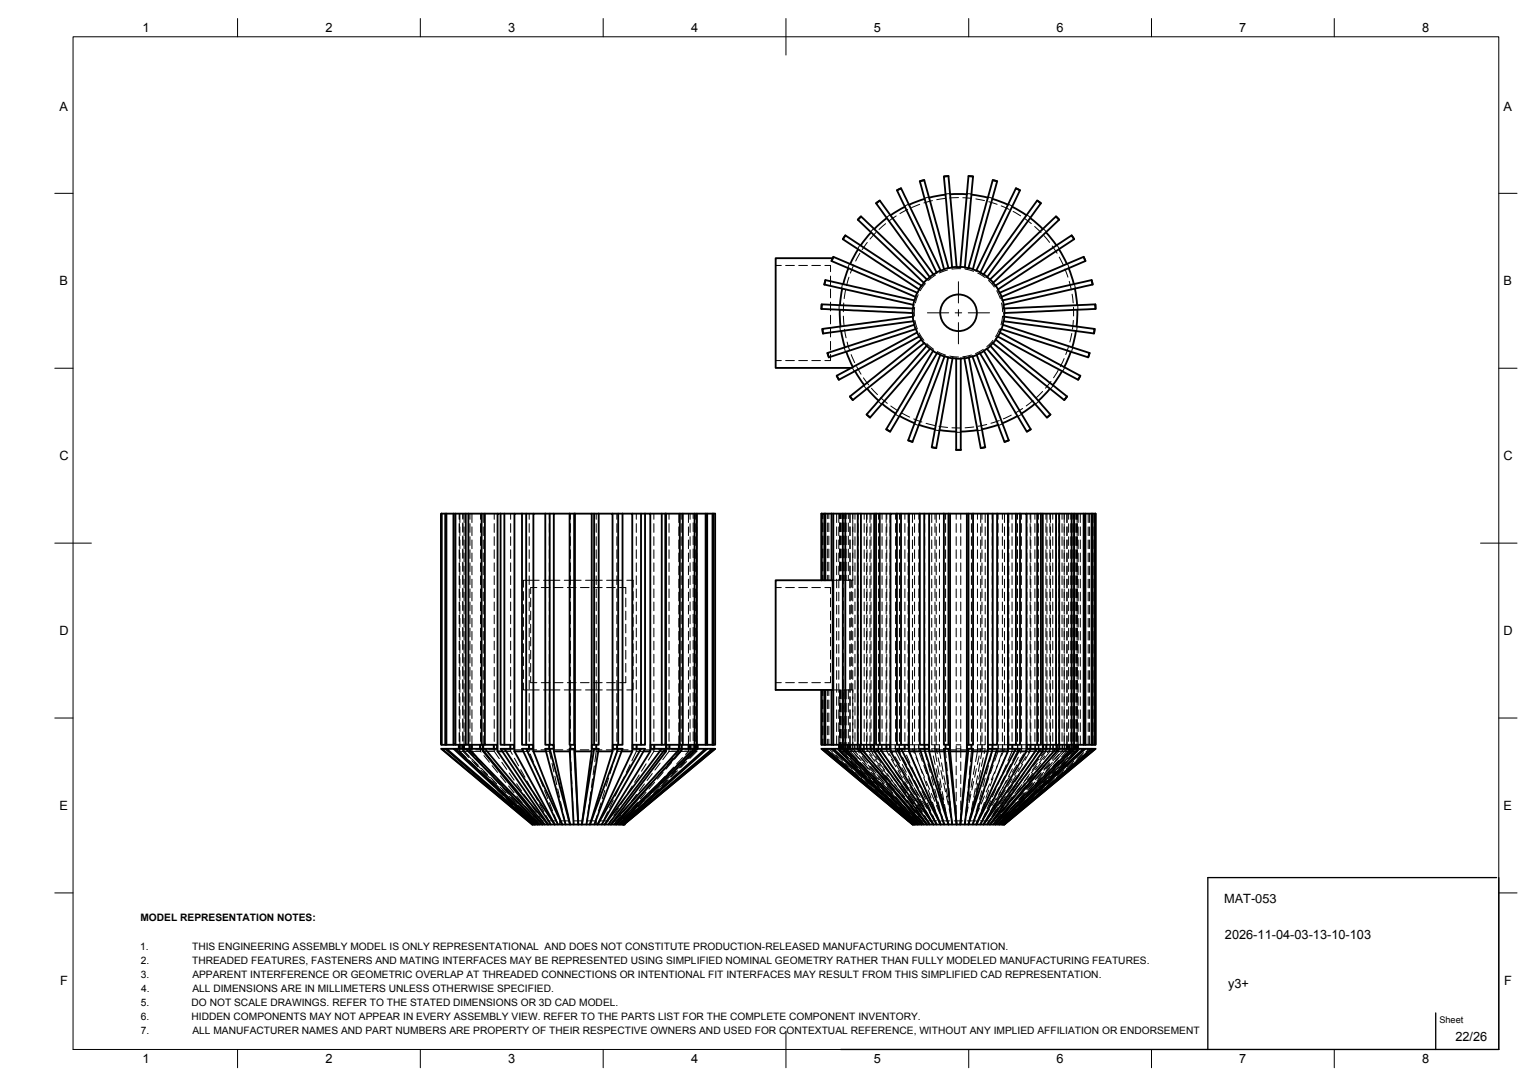
ISO-10303-21;
HEADER;
FILE_DESCRIPTION (('STEP AP214'),
    '1' );
FILE_NAME ('y3+.step',
    '2026-10-10T03:43:58',
    ( '' ),
    ( '' ),
    'SwSTEP 2.0',
    'SolidWorks 2026',
    '' );
FILE_SCHEMA (( 'AUTOMOTIVE_DESIGN' ));
ENDSEC;

DATA;
#2=ORIENTED_EDGE ( 'NONE', *, *, #57099, .F. ) ;
#4=DIRECTION ( 'NONE',  ( 0.000000000000000000, 0.000000000000000000, -1.000000000000000000 ) ) ;
#5=CARTESIAN_POINT ( 'NONE',  ( -64.61430802170492882, 7.070445451047391749, 170.0000000000000000 ) ) ;
#16=VERTEX_POINT ( 'NONE', #24964 ) ;
#40=CARTESIAN_POINT ( 'NONE',  ( 0.000000000000000000, 0.000000000000000000, 170.0000000000000000 ) ) ;
#47=ORIENTED_EDGE ( 'NONE', *, *, #8300, .T. ) ;
#51=CARTESIAN_POINT ( 'NONE',  ( -21.95369412746239846, -11.95973721106846455, 0.000000000000000000 ) ) ;
#52=ORIENTED_EDGE ( 'NONE', *, *, #19951, .T. ) ;
#76=ORIENTED_EDGE ( 'NONE', *, *, #47792, .F. ) ;
#86=ORIENTED_EDGE ( 'NONE', *, *, #42856, .F. ) ;
#93=ORIENTED_EDGE ( 'NONE', *, *, #10645, .F. ) ;
#99=CARTESIAN_POINT ( 'NONE',  ( -67.57266509268163190, 32.54128043381644630, 0.000000000000000000 ) ) ;
#100=DIRECTION ( 'NONE',  ( -0.000000000000000000, -0.000000000000000000, -1.000000000000000000 ) ) ;
#117=DIRECTION ( 'NONE',  ( 1.000000000000000000, 0.000000000000000000, 0.000000000000000000 ) ) ;
#121=ORIENTED_EDGE ( 'NONE', *, *, #21419, .T. ) ;
#132=ORIENTED_EDGE ( 'NONE', *, *, #17716, .F. ) ;
#133=EDGE_CURVE ( 'NONE', #13308, #45468, #35156, .T. ) ;
#167=CIRCLE ( 'NONE', #18114, 65.36598343705435354 ) ;
#172=DIRECTION ( 'NONE',  ( -0.000000000000000000, -0.000000000000000000, -1.000000000000000000 ) ) ;
#181=ORIENTED_EDGE ( 'NONE', *, *, #66204, .T. ) ;
#187=LINE ( 'NONE', #36804, #20712 ) ;
#194=CARTESIAN_POINT ( 'NONE',  ( 0.000000000000000000, 0.000000000000000000, 43.58025477438756212 ) ) ;
#196=CARTESIAN_POINT ( 'NONE',  ( -9.964117946888929822, -64.24592483216726180, 170.0000000000000000 ) ) ;
#200=DIRECTION ( 'NONE',  ( -0.000000000000000000, -0.000000000000000000, -1.000000000000000000 ) ) ;
#201=CIRCLE ( 'NONE', #46254, 65.00000000000000000 ) ;
#202=ORIENTED_EDGE ( 'NONE', *, *, #20149, .F. ) ;
#211=EDGE_CURVE ( 'NONE', #44289, #2530, #5891, .T. ) ;
#214=ORIENTED_EDGE ( 'NONE', *, *, #67051, .T. ) ;
#215=ORIENTED_EDGE ( 'NONE', *, *, #11970, .T. ) ;
#220=DIRECTION ( 'NONE',  ( 0.9639628606958550172, -0.2660368455666687892, 0.000000000000000000 ) ) ;
#221=DIRECTION ( 'NONE',  ( -0.3930250316539278255, 0.9195277725514487965, 0.000000000000000000 ) ) ;
#223=CARTESIAN_POINT ( 'NONE',  ( 23.81581464765719502, -7.603089679099516829, 0.000000000000000000 ) ) ;
#238=CARTESIAN_POINT ( 'NONE',  ( -44.00727179482512241, -47.83680621839620528, 170.0000000000000000 ) ) ;
#240=CARTESIAN_POINT ( 'NONE',  ( -52.69240448066584293, -53.30312580971443026, 41.38025477438755928 ) ) ;
#242=VERTEX_POINT ( 'NONE', #53046 ) ;
#247=CARTESIAN_POINT ( 'NONE',  ( -51.55432476821989951, -3.384920738951192387, 26.66469104408689006 ) ) ;
#249=CARTESIAN_POINT ( 'NONE',  ( 53.32245423372616244, -37.19594572654634845, 0.000000000000000000 ) ) ;
#251=ORIENTED_EDGE ( 'NONE', *, *, #47236, .T. ) ;
#252=VECTOR ( 'NONE', #36887, 999.9999999999998863 ) ;
#254=CARTESIAN_POINT ( 'NONE',  ( 63.74253542338309586, -39.54050679744447194, 170.0000000000000000 ) ) ;
#255=CARTESIAN_POINT ( 'NONE',  ( -3.364862276288897558, 74.92447999059858432, 0.000000000000000000 ) ) ;
#259=ORIENTED_EDGE ( 'NONE', *, *, #53036, .T. ) ;
#288=EDGE_CURVE ( 'NONE', #56752, #64051, #11518, .T. ) ;
#291=CARTESIAN_POINT ( 'NONE',  ( 21.98745393275193294, 71.71550996510526943, 170.0000000000000000 ) ) ;
#304=FACE_OUTER_BOUND ( 'NONE', #28790, .T. ) ;
#308=VERTEX_POINT ( 'NONE', #33352 ) ;
#310=ORIENTED_EDGE ( 'NONE', *, *, #16110, .F. ) ;
#337=ORIENTED_EDGE ( 'NONE', *, *, #57085, .T. ) ;
#341=LINE ( 'NONE', #41886, #16088 ) ;
#348=CARTESIAN_POINT ( 'NONE',  ( 46.76173513940489812, 58.63736118510233553, 0.000000000000000000 ) ) ;
#351=CARTESIAN_POINT ( 'NONE',  ( 0.000000000000000000, 0.000000000000000000, 170.0000000000000000 ) ) ;
#354=VECTOR ( 'NONE', #29148, 1000.000000000000000 ) ;
#363=EDGE_CURVE ( 'NONE', #35105, #14663, #10362, .T. ) ;
#367=LINE ( 'NONE', #1073, #48782 ) ;
#369=FACE_OUTER_BOUND ( 'NONE', #27784, .T. ) ;
#378=FACE_OUTER_BOUND ( 'NONE', #48491, .T. ) ;
#380=EDGE_CURVE ( 'NONE', #35096, #37085, #27704, .T. ) ;
#391=CARTESIAN_POINT ( 'NONE',  ( 43.69793136154977020, -27.56441338823224640, 26.66469104408688651 ) ) ;
#407=ADVANCED_FACE ( 'NONE', ( #49850 ), #23142, .T. ) ;
#411=VECTOR ( 'NONE', #777, 999.9999999999998863 ) ;
#417=VERTEX_POINT ( 'NONE', #18553 ) ;
#424=LINE ( 'NONE', #15226, #9320 ) ;
#425=ORIENTED_EDGE ( 'NONE', *, *, #19954, .T. ) ;
#434=DIRECTION ( 'NONE',  ( 3.687791819402438921E-18, 3.525890001671295931E-18, -1.000000000000000000 ) ) ;
#438=LINE ( 'NONE', #10639, #37259 ) ;
#451=PLANE ( 'NONE',  #68993 ) ;
#452=LINE ( 'NONE', #27883, #8566 ) ;
#460=VECTOR ( 'NONE', #45689, 1000.000000000000000 ) ;
#461=CARTESIAN_POINT ( 'NONE',  ( -4.337405327940998312, -24.62086340933521456, 0.000000000000000000 ) ) ;
#469=EDGE_CURVE ( 'NONE', #64523, #66077, #7997, .T. ) ;
#472=DIRECTION ( 'NONE',  ( -1.000000000000000000, 0.000000000000000000, 0.000000000000000000 ) ) ;
#475=CARTESIAN_POINT ( 'NONE',  ( -59.42430146430388049, -27.22983999535795618, 41.38025477438755928 ) ) ;
#476=VERTEX_POINT ( 'NONE', #20615 ) ;
#478=ORIENTED_EDGE ( 'NONE', *, *, #43254, .F. ) ;
#482=FACE_OUTER_BOUND ( 'NONE', #35633, .T. ) ;
#488=ORIENTED_EDGE ( 'NONE', *, *, #3364, .T. ) ;
#489=LINE ( 'NONE', #22994, #3698 ) ;
#496=LINE ( 'NONE', #54649, #32650 ) ;
#497=CARTESIAN_POINT ( 'NONE',  ( 7.533997733928855745, 64.93035244659017735, 43.58025477438756212 ) ) ;
#498=EDGE_CURVE ( 'NONE', #7475, #40883, #67262, .T. ) ;
#501=ORIENTED_EDGE ( 'NONE', *, *, #47379, .F. ) ;
#509=EDGE_LOOP ( 'NONE', ( #15892, #23987, #55681, #42144 ) ) ;
#510=VECTOR ( 'NONE', #66224, 1000.000000000000227 ) ;
#511=DIRECTION ( 'NONE',  ( -1.000000000000000000, 0.000000000000000000, 0.000000000000000000 ) ) ;
#515=FACE_OUTER_BOUND ( 'NONE', #61318, .T. ) ;
#520=DIRECTION ( 'NONE',  ( -0.000000000000000000, -0.000000000000000000, -1.000000000000000000 ) ) ;
#523=AXIS2_PLACEMENT_3D ( 'NONE', #9987, #4698, #14905 ) ;
#528=FACE_OUTER_BOUND ( 'NONE', #60025, .T. ) ;
#531=ORIENTED_EDGE ( 'NONE', *, *, #31450, .F. ) ;
#532=ORIENTED_EDGE ( 'NONE', *, *, #61150, .T. ) ;
#535=CARTESIAN_POINT ( 'NONE',  ( -45.81425895439360829, -46.10914959592906115, 40.00000000000003553 ) ) ;
#541=ORIENTED_EDGE ( 'NONE', *, *, #47134, .F. ) ;
#547=LINE ( 'NONE', #52959, #56357 ) ;
#552=AXIS2_PLACEMENT_3D ( 'NONE', #54276, #10682, #49001 ) ;
#554=EDGE_CURVE ( 'NONE', #23240, #35650, #11353, .T. ) ;
#555=DIRECTION ( 'NONE',  ( -0.9909497617679352555, 0.1342332658176522697, 2.500042656554811326E-16 ) ) ;
#562=AXIS2_PLACEMENT_3D ( 'NONE', #30602, #57334, #47443 ) ;
#563=AXIS2_PLACEMENT_3D ( 'NONE', #26561, #16346, #37803 ) ;
#566=DIRECTION ( 'NONE',  ( 0.000000000000000000, 0.000000000000000000, 1.000000000000000000 ) ) ;
#567=CARTESIAN_POINT ( 'NONE',  ( -65.36598343705435354, 0.000000000000000000, 41.38025477438755928 ) ) ;
#574=DIRECTION ( 'NONE',  ( -0.000000000000000000, -0.000000000000000000, -1.000000000000000000 ) ) ;
#579=LINE ( 'NONE', #5503, #875 ) ;
#581=DIRECTION ( 'NONE',  ( 0.000000000000000000, 0.000000000000000000, 1.000000000000000000 ) ) ;
#590=DIRECTION ( 'NONE',  ( -0.000000000000000000, -0.000000000000000000, 1.000000000000000000 ) ) ;
#591=LINE ( 'NONE', #22043, #68889 ) ;
#594=CARTESIAN_POINT ( 'NONE',  ( -4.613603609465552147, 74.86839895266042788, 43.58025477438756923 ) ) ;
#597=CARTESIAN_POINT ( 'NONE',  ( -58.00979178563854077, 29.32343869649098878, 170.0000000000000000 ) ) ;
#608=VECTOR ( 'NONE', #24397, 1000.000000000000000 ) ;
#611=FACE_OUTER_BOUND ( 'NONE', #10480, .T. ) ;
#616=ORIENTED_EDGE ( 'NONE', *, *, #58079, .T. ) ;
#623=EDGE_CURVE ( 'NONE', #36282, #8304, #15353, .T. ) ;
#634=VERTEX_POINT ( 'NONE', #30845 ) ;
#636=B_SPLINE_CURVE_WITH_KNOTS ( 'NONE', 3,
 ( #25804, #40931, #40580, #34971, #29685, #46197 ),
 .UNSPECIFIED., .F., .F.,
 ( 4, 2, 4 ),
 ( 1.095770181104900047E-06, 0.03239442681617710901, 0.06478775786217311206 ),
 .UNSPECIFIED. ) ;
#659=VECTOR ( 'NONE', #43417, 1000.000000000000000 ) ;
#662=CARTESIAN_POINT ( 'NONE',  ( 8.820885042878503057, -74.43053605947400797, 41.38025477438755928 ) ) ;
#668=AXIS2_PLACEMENT_3D ( 'NONE', #7424, #55591, #18310 ) ;
#670=LINE ( 'NONE', #22117, #19760 ) ;
#671=VERTEX_POINT ( 'NONE', #68799 ) ;
#672=CARTESIAN_POINT ( 'NONE',  ( 36.85262215550149278, -53.56030941157680303, 41.38025477438755928 ) ) ;
#677=CARTESIAN_POINT ( 'NONE',  ( 21.98745393275290994, -71.71550996510497100, 170.0000000000000000 ) ) ;
#679=CARTESIAN_POINT ( 'NONE',  ( -39.55079474733700096, 51.59997227570983114, 43.58025477438756923 ) ) ;
#682=DIRECTION ( 'NONE',  ( -0.000000000000000000, -0.000000000000000000, -1.000000000000000000 ) ) ;
#686=CARTESIAN_POINT ( 'NONE',  ( -28.30427060690108476, 69.40159203110296460, 41.38025477438755928 ) ) ;
#688=ORIENTED_EDGE ( 'NONE', *, *, #20639, .F. ) ;
#695=VERTEX_POINT ( 'NONE', #62510 ) ;
#697=LINE ( 'NONE', #39377, #69339 ) ;
#700=CYLINDRICAL_SURFACE ( 'NONE', #28223, 65.00000000000000000 ) ;
#704=EDGE_CURVE ( 'NONE', #58577, #50465, #36961, .T. ) ;
#705=FACE_OUTER_BOUND ( 'NONE', #37615, .T. ) ;
#706=AXIS2_PLACEMENT_3D ( 'NONE', #9153, #14435, #51716 ) ;
#707=B_SPLINE_CURVE_WITH_KNOTS ( 'NONE', 3,
 ( #53839, #38731, #5658, #1443, #27118, #43988 ),
 .UNSPECIFIED., .F., .F.,
 ( 4, 2, 4 ),
 ( 1.095770181099519270E-06, 0.03239442681617710207, 0.06478775786217311206 ),
 .UNSPECIFIED. ) ;
#714=CARTESIAN_POINT ( 'NONE',  ( 49.76301652092224970, -41.81676920493044491, 170.0000000000000000 ) ) ;
#716=EDGE_CURVE ( 'NONE', #67683, #29070, #35781, .T. ) ;
#718=VECTOR ( 'NONE', #42490, 1000.000000000000227 ) ;
#720=DIRECTION ( 'NONE',  ( -0.000000000000000000, -0.000000000000000000, -1.000000000000000000 ) ) ;
#724=ORIENTED_EDGE ( 'NONE', *, *, #31613, .F. ) ;
#725=ADVANCED_FACE ( 'NONE', ( #30491 ), #68140, .T. ) ;
#731=ORIENTED_EDGE ( 'NONE', *, *, #55277, .F. ) ;
#733=CARTESIAN_POINT ( 'NONE',  ( -2.116120943111210906, -74.98056102853675497, 170.0000000000000000 ) ) ;
#736=DIRECTION ( 'NONE',  ( -1.000000000000000000, 0.000000000000000000, 0.000000000000000000 ) ) ;
#739=ORIENTED_EDGE ( 'NONE', *, *, #39691, .T. ) ;
#741=CARTESIAN_POINT ( 'NONE',  ( 0.000000000000000000, 0.000000000000000000, 43.58025477438756212 ) ) ;
#747=LINE ( 'NONE', #64413, #62651 ) ;
#749=DIRECTION ( 'NONE',  ( -0.000000000000000000, -0.000000000000000000, 1.000000000000000000 ) ) ;
#759=DIRECTION ( 'NONE',  ( 1.469488203625002396E-16, 2.022576995815139509E-16, 1.000000000000000000 ) ) ;
#766=AXIS2_PLACEMENT_3D ( 'NONE', #19277, #30885, #3455 ) ;
#775=ADVANCED_FACE ( 'NONE', ( #1507 ), #17696, .F. ) ;
#777=DIRECTION ( 'NONE',  ( 0.7530714660036099684, 0.6579387259397138088, 0.000000000000000000 ) ) ;
#786=CARTESIAN_POINT ( 'NONE',  ( 18.66447700095702444, -37.32227186998856894, 13.79046340968177553 ) ) ;
#797=EDGE_CURVE ( 'NONE', #15914, #43922, #8376, .T. ) ;
#809=EDGE_CURVE ( 'NONE', #32676, #18463, #67463, .T. ) ;
#813=CARTESIAN_POINT ( 'NONE',  ( 0.000000000000000000, 0.000000000000000000, 43.58025477438756212 ) ) ;
#816=EDGE_CURVE ( 'NONE', #58443, #61153, #12692, .T. ) ;
#822=VECTOR ( 'NONE', #43573, 1000.000000000000114 ) ;
#830=ORIENTED_EDGE ( 'NONE', *, *, #22808, .F. ) ;
#831=ORIENTED_EDGE ( 'NONE', *, *, #67075, .T. ) ;
#834=CARTESIAN_POINT ( 'NONE',  ( 17.98081503251174240, -17.36923402935755689, 0.000000000000000000 ) ) ;
#852=ORIENTED_EDGE ( 'NONE', *, *, #43049, .T. ) ;
#860=VECTOR ( 'NONE', #7201, 1000.000000000000000 ) ;
#863=VERTEX_POINT ( 'NONE', #31892 ) ;
#871=EDGE_CURVE ( 'NONE', #64668, #6453, #9752, .T. ) ;
#872=LINE ( 'NONE', #58556, #659 ) ;
#875=VECTOR ( 'NONE', #26956, 1000.000000000000000 ) ;
#887=CARTESIAN_POINT ( 'NONE',  ( 0.000000000000000000, 0.000000000000000000, 170.0000000000000000 ) ) ;
#900=VECTOR ( 'NONE', #4776, 1000.000000000000000 ) ;
#905=CARTESIAN_POINT ( 'NONE',  ( -65.00200000000002376, 1.249999999999979350, 170.0000000000000000 ) ) ;
#925=VERTEX_POINT ( 'NONE', #60704 ) ;
#926=DIRECTION ( 'NONE',  ( 0.2660368455666687892, 0.9639628606958550172, -0.000000000000000000 ) ) ;
#928=CARTESIAN_POINT ( 'NONE',  ( 32.06997139192792901, -56.95813133885440749, 41.38025477438755928 ) ) ;
#936=EDGE_CURVE ( 'NONE', #57871, #43209, #58711, .T. ) ;
#937=VERTEX_POINT ( 'NONE', #1979 ) ;
#939=EDGE_LOOP ( 'NONE', ( #6618, #33629, #34700, #50943, #34117, #44911, #4182, #50730, #17595 ) ) ;
#945=LINE ( 'NONE', #32946, #35612 ) ;
#948=CARTESIAN_POINT ( 'NONE',  ( -23.98664764928003734, -23.27925803097926050, 6.893343212288939981 ) ) ;
#951=CARTESIAN_POINT ( 'NONE',  ( -18.89790202299212396, 62.20684691518604836, 170.0000000000000000 ) ) ;
#962=ADVANCED_FACE ( 'NONE', ( #2322 ), #45219, .F. ) ;
#974=CARTESIAN_POINT ( 'NONE',  ( -16.20761984364699870, -34.73915265837867850, 13.32819397642333037 ) ) ;
#976=CARTESIAN_POINT ( 'NONE',  ( -58.00979178563811445, -29.32343869649178814, 170.0000000000000000 ) ) ;
#995=FACE_OUTER_BOUND ( 'NONE', #20434, .T. ) ;
#998=CARTESIAN_POINT ( 'NONE',  ( 0.000000000000000000, 0.000000000000000000, 40.00000000000003553 ) ) ;
#1004=ORIENTED_EDGE ( 'NONE', *, *, #19047, .F. ) ;
#1012=CARTESIAN_POINT ( 'NONE',  ( -4.610955605662443446, -74.80943656680585718, 41.38025477438755928 ) ) ;
#1026=CARTESIAN_POINT ( 'NONE',  ( 9.962235950564874543, 64.23203137738424573, 170.0000000000000000 ) ) ;
#1032=EDGE_LOOP ( 'NONE', ( #4642, #65171, #45931, #15526 ) ) ;
#1043=EDGE_CURVE ( 'NONE', #48718, #23096, #46599, .T. ) ;
#1044=EDGE_CURVE ( 'NONE', #21376, #7953, #3355, .T. ) ;
#1046=ORIENTED_EDGE ( 'NONE', *, *, #35292, .F. ) ;
#1048=ORIENTED_EDGE ( 'NONE', *, *, #61066, .T. ) ;
#1050=DIRECTION ( 'NONE',  ( 0.000000000000000000, 0.000000000000000000, 1.000000000000000000 ) ) ;
#1061=DIRECTION ( 'NONE',  ( 0.000000000000000000, 0.000000000000000000, 1.000000000000000000 ) ) ;
#1064=CARTESIAN_POINT ( 'NONE',  ( 9.068001575458771057, -57.63052812422861138, 27.58472369369409094 ) ) ;
#1071=DIRECTION ( 'NONE',  ( 1.000000000000000000, 0.000000000000000000, 0.000000000000000000 ) ) ;
#1073=CARTESIAN_POINT ( 'NONE',  ( -31.90315521289150524, 56.64813493366005304, 41.38025477438755928 ) ) ;
#1074=CIRCLE ( 'NONE', #13440, 25.12245591505646303 ) ;
#1085=VERTEX_POINT ( 'NONE', #8291 ) ;
#1088=B_SPLINE_CURVE_WITH_KNOTS ( 'NONE', 3,
 ( #39692, #51297, #61148, #29140, #22816, #34436 ),
 .UNSPECIFIED., .F., .F.,
 ( 4, 2, 4 ),
 ( 1.095770181107971388E-06, 0.03239442681617708819, 0.06478775786217308430 ),
 .UNSPECIFIED. ) ;
#1094=DIRECTION ( 'NONE',  ( -1.000000000000000000, 0.000000000000000000, 0.000000000000000000 ) ) ;
#1096=DIRECTION ( 'NONE',  ( -0.5877852522924686962, -0.8090169943749506709, 2.500042656554809354E-16 ) ) ;
#1097=DIRECTION ( 'NONE',  ( 1.000000000000000000, 0.000000000000000000, 0.000000000000000000 ) ) ;
#1115=AXIS2_PLACEMENT_3D ( 'NONE', #49664, #60929, #1492 ) ;
#1123=LINE ( 'NONE', #12371, #41190 ) ;
#1124=DIRECTION ( 'NONE',  ( -0.3513748240813305279, -0.9362348706397417564, 5.102127870520021228E-18 ) ) ;
#1127=ADVANCED_FACE ( 'NONE', ( #53591 ), #52006, .T. ) ;
#1143=CYLINDRICAL_SURFACE ( 'NONE', #35228, 65.36598343705435354 ) ;
#1144=CONICAL_SURFACE ( 'NONE', #55059, 65.00000000000000000, 0.7853981633974497223 ) ;
#1146=VERTEX_POINT ( 'NONE', #15293 ) ;
#1148=CARTESIAN_POINT ( 'NONE',  ( -1.666933348992581942, 64.97862212458815634, 40.00000000000003553 ) ) ;
#1152=CARTESIAN_POINT ( 'NONE',  ( -28.30427060690011132, -69.40159203110334829, 41.38025477438755928 ) ) ;
#1154=ORIENTED_EDGE ( 'NONE', *, *, #54505, .F. ) ;
#1156=CARTESIAN_POINT ( 'NONE',  ( -41.50537345350635121, -50.04124777106354571, 3.061616997868437868E-16 ) ) ;
#1161=CARTESIAN_POINT ( 'NONE',  ( 1.667562369266827327, 64.99262834925669097, 170.0000000000000000 ) ) ;
#1168=CARTESIAN_POINT ( 'NONE',  ( 70.34686579112866411, -18.11777090454118877, 41.38025477438755928 ) ) ;
#1171=ORIENTED_EDGE ( 'NONE', *, *, #16376, .T. ) ;
#1182=CARTESIAN_POINT ( 'NONE',  ( 47.70222499156757578, 57.81185381817647340, 41.38025477438755928 ) ) ;
#1185=ORIENTED_EDGE ( 'NONE', *, *, #50012, .T. ) ;
#1197=DIRECTION ( 'NONE',  ( -0.000000000000000000, -0.000000000000000000, -1.000000000000000000 ) ) ;
#1199=ORIENTED_EDGE ( 'NONE', *, *, #5184, .F. ) ;
#1215=LINE ( 'NONE', #65590, #12769 ) ;
#1217=FACE_OUTER_BOUND ( 'NONE', #47662, .T. ) ;
#1223=AXIS2_PLACEMENT_3D ( 'NONE', #64449, #31748, #54221 ) ;
#1230=ORIENTED_EDGE ( 'NONE', *, *, #60967, .T. ) ;
#1237=LINE ( 'NONE', #11423, #47052 ) ;
#1240=DIRECTION ( 'NONE',  ( -0.1342332658176667304, 0.9909497617679331460, 0.000000000000000000 ) ) ;
#1243=CARTESIAN_POINT ( 'NONE',  ( -25.87147652227456263, 70.00000000000000000, 129.5802547743875550 ) ) ;
#1246=EDGE_CURVE ( 'NONE', #2785, #21253, #66340, .T. ) ;
#1258=CARTESIAN_POINT ( 'NONE',  ( 14.59045944429412600, 20.30070179093326743, 0.000000000000000000 ) ) ;
#1259=FACE_OUTER_BOUND ( 'NONE', #14240, .T. ) ;
#1266=DIRECTION ( 'NONE',  ( -0.000000000000000000, -0.000000000000000000, 1.000000000000000000 ) ) ;
#1269=ORIENTED_EDGE ( 'NONE', *, *, #19129, .T. ) ;
#1270=EDGE_CURVE ( 'NONE', #30832, #4530, #489, .T. ) ;
#1278=CARTESIAN_POINT ( 'NONE',  ( 18.66447740837935854, 37.32227262710744498, 13.79046412339527805 ) ) ;
#1284=LINE ( 'NONE', #28007, #53475 ) ;
#1286=AXIS2_PLACEMENT_3D ( 'NONE', #32056, #27454, #22537 ) ;
#1290=LINE ( 'NONE', #61422, #65606 ) ;
#1294=PLANE ( 'NONE',  #9088 ) ;
#1295=ADVANCED_FACE ( 'NONE', ( #22639 ), #18070, .T. ) ;
#1296=ADVANCED_FACE ( 'NONE', ( #39520 ), #6806, .T. ) ;
#1298=CARTESIAN_POINT ( 'NONE',  ( -29.72794928047597551, -29.28418875150963174, 13.79046340968179329 ) ) ;
#1305=CARTESIAN_POINT ( 'NONE',  ( 19.62566184736102315, -15.48655536434847413, 0.000000000000000000 ) ) ;
#1318=DIRECTION ( 'NONE',  ( -0.000000000000000000, -0.000000000000000000, -1.000000000000000000 ) ) ;
#1325=AXIS2_PLACEMENT_3D ( 'NONE', #67107, #4108, #14995 ) ;
#1327=ORIENTED_EDGE ( 'NONE', *, *, #10704, .T. ) ;
#1328=CARTESIAN_POINT ( 'NONE',  ( -42.36049017605959932, 61.90437280228238137, 170.0000000000000000 ) ) ;
#1341=DIRECTION ( 'NONE',  ( -1.000000000000000000, 0.000000000000000000, 0.000000000000000000 ) ) ;
#1343=EDGE_LOOP ( 'NONE', ( #19373, #43322, #68066, #46993 ) ) ;
#1345=ADVANCED_FACE ( 'NONE', ( #65205 ), #27915, .T. ) ;
#1354=ORIENTED_EDGE ( 'NONE', *, *, #2252, .T. ) ;
#1360=CARTESIAN_POINT ( 'NONE',  ( 64.38365952014046911, -38.46744580544211800, 0.000000000000000000 ) ) ;
#1364=ORIENTED_EDGE ( 'NONE', *, *, #65796, .F. ) ;
#1367=B_SPLINE_CURVE_WITH_KNOTS ( 'NONE', 3,
 ( #22102, #64670, #38274, #43542, #60435, #59720 ),
 .UNSPECIFIED., .F., .F.,
 ( 4, 2, 4 ),
 ( 0.03218934490037923812, 0.06469832469447826806, 0.09720730448857729800 ),
 .UNSPECIFIED. ) ;
#1372=CIRCLE ( 'NONE', #41799, 65.36598343705435354 ) ;
#1376=CARTESIAN_POINT ( 'NONE',  ( 24.36509522348982060, 70.94296747916789059, 170.0000000000000000 ) ) ;
#1377=FACE_OUTER_BOUND ( 'NONE', #3277, .T. ) ;
#1380=EDGE_CURVE ( 'NONE', #42777, #60210, #17354, .T. ) ;
#1388=ORIENTED_EDGE ( 'NONE', *, *, #34429, .T. ) ;
#1401=ORIENTED_EDGE ( 'NONE', *, *, #67407, .F. ) ;
#1403=FACE_OUTER_BOUND ( 'NONE', #22851, .T. ) ;
#1407=LINE ( 'NONE', #55564, #7161 ) ;
#1412=ORIENTED_EDGE ( 'NONE', *, *, #13505, .F. ) ;
#1418=EDGE_LOOP ( 'NONE', ( #66100, #12328, #6607, #20703 ) ) ;
#1423=VERTEX_POINT ( 'NONE', #51467 ) ;
#1430=AXIS2_PLACEMENT_3D ( 'NONE', #24335, #67253, #13759 ) ;
#1439=AXIS2_PLACEMENT_3D ( 'NONE', #31545, #574, #22025 ) ;
#1443=CARTESIAN_POINT ( 'NONE',  ( 32.23328773803155656, 26.50150638838968931, 13.79046340968178441 ) ) ;
#1444=DIRECTION ( 'NONE',  ( -1.000000000000000000, 0.000000000000000000, 0.000000000000000000 ) ) ;
#1447=CYLINDRICAL_SURFACE ( 'NONE', #33698, 65.36598343705435354 ) ;
#1452=ORIENTED_EDGE ( 'NONE', *, *, #49262, .F. ) ;
#1455=CARTESIAN_POINT ( 'NONE',  ( 0.000000000000000000, 0.000000000000000000, 170.0000000000000000 ) ) ;
#1461=FACE_OUTER_BOUND ( 'NONE', #63718, .T. ) ;
#1472=ORIENTED_EDGE ( 'NONE', *, *, #33458, .F. ) ;
#1490=EDGE_CURVE ( 'NONE', #21376, #25377, #62094, .T. ) ;
#1492=DIRECTION ( 'NONE',  ( -1.000000000000000000, 0.000000000000000000, 0.000000000000000000 ) ) ;
#1499=EDGE_CURVE ( 'NONE', #64497, #58120, #57102, .T. ) ;
#1501=ORIENTED_EDGE ( 'NONE', *, *, #10704, .F. ) ;
#1504=DIRECTION ( 'NONE',  ( -1.000000000000000000, 0.000000000000000000, 0.000000000000000000 ) ) ;
#1507=FACE_OUTER_BOUND ( 'NONE', #30878, .T. ) ;
#1511=CIRCLE ( 'NONE', #41934, 25.12245591505646303 ) ;
#1512=DIRECTION ( 'NONE',  ( -1.000000000000000000, 0.000000000000000000, 0.000000000000000000 ) ) ;
#1517=DIRECTION ( 'NONE',  ( 0.000000000000000000, -0.000000000000000000, -1.000000000000000000 ) ) ;
#1527=VECTOR ( 'NONE', #25037, 1000.000000000000000 ) ;
#1542=CARTESIAN_POINT ( 'NONE',  ( 20.89850557012451659, -13.94239061780404043, 0.000000000000000000 ) ) ;
#1546=EDGE_LOOP ( 'NONE', ( #41839, #52195, #39224, #64714 ) ) ;
#1547=LINE ( 'NONE', #6482, #48398 ) ;
#1567=CARTESIAN_POINT ( 'NONE',  ( -51.84164840787185113, 39.21024726209461875, 40.00000000000003553 ) ) ;
#1568=PLANE ( 'NONE',  #65557 ) ;
#1571=CARTESIAN_POINT ( 'NONE',  ( 0.000000000000000000, 0.000000000000000000, 41.38025477438755928 ) ) ;
#1572=VERTEX_POINT ( 'NONE', #44260 ) ;
#1573=AXIS2_PLACEMENT_3D ( 'NONE', #37705, #53531, #59155 ) ;
#1574=ORIENTED_EDGE ( 'NONE', *, *, #43551, .F. ) ;
#1576=VECTOR ( 'NONE', #39227, 1000.000000000000000 ) ;
#1579=EDGE_LOOP ( 'NONE', ( #58682, #202, #19140, #26203 ) ) ;
#1584=DIRECTION ( 'NONE',  ( -0.000000000000000000, -0.000000000000000000, -1.000000000000000000 ) ) ;
#1585=EDGE_LOOP ( 'NONE', ( #52041, #42802, #63554, #14608 ) ) ;
#1586=CARTESIAN_POINT ( 'NONE',  ( 55.46196446482127840, -34.59309596431295120, 6.377659838150088165E-18 ) ) ;
#1587=LINE ( 'NONE', #12150, #22150 ) ;
#1604=ADVANCED_FACE ( 'NONE', ( #63911 ), #11468, .F. ) ;
#1605=ORIENTED_EDGE ( 'NONE', *, *, #40738, .T. ) ;
#1614=CARTESIAN_POINT ( 'NONE',  ( -33.00964028082890422, -25.52799247005623329, 13.79046412380261799 ) ) ;
#1622=DIRECTION ( 'NONE',  ( -1.000000000000000000, 0.000000000000000000, 0.000000000000000000 ) ) ;
#1630=VECTOR ( 'NONE', #25226, 1000.000000000000000 ) ;
#1633=PLANE ( 'NONE',  #28492 ) ;
#1637=CARTESIAN_POINT ( 'NONE',  ( 55.46196446482078812, 34.59309596431376121, 43.58025477438756212 ) ) ;
#1647=DIRECTION ( 'NONE',  ( -0.9749279121818227312, -0.2225209339563184729, 2.500042656554810833E-16 ) ) ;
#1649=DIRECTION ( 'NONE',  ( -1.000000000000000000, 0.000000000000000000, 0.000000000000000000 ) ) ;
#1655=CARTESIAN_POINT ( 'NONE',  ( 0.000000000000000000, 0.000000000000000000, 0.000000000000000000 ) ) ;
#1667=CARTESIAN_POINT ( 'NONE',  ( -21.44923269555038203, 47.00251555413245796, 26.66469066592269144 ) ) ;
#1671=CARTESIAN_POINT ( 'NONE',  ( -21.27554331372999741, 61.43430442924864820, 41.38025477438755928 ) ) ;
#1678=LINE ( 'NONE', #60760, #6233 ) ;
#1682=AXIS2_PLACEMENT_3D ( 'NONE', #36378, #26165, #16299 ) ;
#1683=ORIENTED_EDGE ( 'NONE', *, *, #47236, .F. ) ;
#1684=ORIENTED_EDGE ( 'NONE', *, *, #9687, .F. ) ;
#1689=DIRECTION ( 'NONE',  ( 0.000000000000000000, 0.000000000000000000, -1.000000000000000000 ) ) ;
#1691=CARTESIAN_POINT ( 'NONE',  ( -14.79841479960649053, 20.14961338137236524, 0.000000000000000000 ) ) ;
#1692=CARTESIAN_POINT ( 'NONE',  ( 0.000000000000000000, 0.000000000000000000, 170.0000000000000000 ) ) ;
#1693=ADVANCED_FACE ( 'NONE', ( #50514 ), #28004, .F. ) ;
#1710=DIRECTION ( 'NONE',  ( -0.000000000000000000, -0.000000000000000000, 1.000000000000000000 ) ) ;
#1714=VERTEX_POINT ( 'NONE', #60375 ) ;
#1720=EDGE_LOOP ( 'NONE', ( #58958, #10654, #36258, #10054 ) ) ;
#1723=AXIS2_PLACEMENT_3D ( 'NONE', #47192, #4301, #14500 ) ;
#1733=CARTESIAN_POINT ( 'NONE',  ( -65.36598343705435354, 0.000000000000000000, 41.38025477438755928 ) ) ;
#1734=VERTEX_POINT ( 'NONE', #23450 ) ;
#1747=ORIENTED_EDGE ( 'NONE', *, *, #14153, .F. ) ;
#1749=ORIENTED_EDGE ( 'NONE', *, *, #35351, .F. ) ;
#1751=CARTESIAN_POINT ( 'NONE',  ( -53.09243148547984248, -24.18057212396687206, 27.58472315868180402 ) ) ;
#1757=CARTESIAN_POINT ( 'NONE',  ( -25.87147652227456263, 70.00000000000000000, 129.5802547743875550 ) ) ;
#1758=ORIENTED_EDGE ( 'NONE', *, *, #20251, .T. ) ;
#1760=LINE ( 'NONE', #39734, #62732 ) ;
#1762=ORIENTED_EDGE ( 'NONE', *, *, #15857, .T. ) ;
#1765=LINE ( 'NONE', #12662, #64488 ) ;
#1766=FACE_OUTER_BOUND ( 'NONE', #21460, .T. ) ;
#1773=CONICAL_SURFACE ( 'NONE', #21987, 74.95140232871122521, 0.8777644062502172329 ) ;
#1775=DIRECTION ( 'NONE',  ( -0.000000000000000000, -0.000000000000000000, -1.000000000000000000 ) ) ;
#1777=ORIENTED_EDGE ( 'NONE', *, *, #26829, .F. ) ;
#1782=CIRCLE ( 'NONE', #53411, 65.00000000000000000 ) ;
#1809=CARTESIAN_POINT ( 'NONE',  ( -7.486743542469090684, -64.58150799671139453, 0.000000000000000000 ) ) ;
#1816=DIRECTION ( 'NONE',  ( -0.9639628606958550172, 0.2660368455666687892, 0.000000000000000000 ) ) ;
#1820=CARTESIAN_POINT ( 'NONE',  ( 69.72313848477159581, -27.50266661387038170, 41.38025477438755928 ) ) ;
#1825=EDGE_LOOP ( 'NONE', ( #14686, #30540, #26848, #56419 ) ) ;
#1829=DIRECTION ( 'NONE',  ( -1.000000000000000000, 0.000000000000000000, 0.000000000000000000 ) ) ;
#1830=AXIS2_PLACEMENT_3D ( 'NONE', #9232, #40890, #24728 ) ;
#1834=AXIS2_PLACEMENT_3D ( 'NONE', #63579, #5178, #9774 ) ;
#1862=ORIENTED_EDGE ( 'NONE', *, *, #67850, .F. ) ;
#1865=CARTESIAN_POINT ( 'NONE',  ( 41.49663191311347532, 50.03028622612080767, 170.0000000000000000 ) ) ;
#1871=DIRECTION ( 'NONE',  ( 0.9510565162951545304, -0.3090169943749447312, 5.102127870520021228E-18 ) ) ;
#1874=LINE ( 'NONE', #65182, #66878 ) ;
#1880=CARTESIAN_POINT ( 'NONE',  ( -53.31111153860250340, -37.18770477615797176, 40.00000000000003553 ) ) ;
#1884=CARTESIAN_POINT ( 'NONE',  ( 15.68296563925591514, -63.09411298019745828, 41.38025477438755928 ) ) ;
#1889=EDGE_LOOP ( 'NONE', ( #31139, #2749, #9487, #15334 ) ) ;
#1897=DIRECTION ( 'NONE',  ( -1.000000000000000000, 0.000000000000000000, 0.000000000000000000 ) ) ;
#1905=DIRECTION ( 'NONE',  ( 0.000000000000000000, 0.000000000000000000, 1.000000000000000000 ) ) ;
#1906=CARTESIAN_POINT ( 'NONE',  ( 60.74750367560238828, -24.13405452624855130, 6.377659838150107425E-18 ) ) ;
#1908=CARTESIAN_POINT ( 'NONE',  ( 69.72313848477159581, -27.50266661387038170, 41.38025477438755928 ) ) ;
#1913=VERTEX_POINT ( 'NONE', #62456 ) ;
#1919=LINE ( 'NONE', #23373, #50231 ) ;
#1932=CYLINDRICAL_SURFACE ( 'NONE', #27329, 65.36598343705435354 ) ;
#1948=ORIENTED_EDGE ( 'NONE', *, *, #5686, .T. ) ;
#1953=DIRECTION ( 'NONE',  ( -0.000000000000000000, -0.000000000000000000, 1.000000000000000000 ) ) ;
#1954=ORIENTED_EDGE ( 'NONE', *, *, #17726, .F. ) ;
#1962=CARTESIAN_POINT ( 'NONE',  ( -2.368959188627906887, 24.88750755625416744, 0.000000000000000000 ) ) ;
#1969=VERTEX_POINT ( 'NONE', #10026 ) ;
#1971=VECTOR ( 'NONE', #42579, 1000.000000000000227 ) ;
#1976=VECTOR ( 'NONE', #23288, 1000.000000000000000 ) ;
#1979=CARTESIAN_POINT ( 'NONE',  ( 0.1285234777254253835, 24.99966963213046611, 0.000000000000000000 ) ) ;
#1995=ORIENTED_EDGE ( 'NONE', *, *, #35814, .T. ) ;
#1998=PLANE ( 'NONE',  #19559 ) ;
#1999=VECTOR ( 'NONE', #221, 1000.000000000000114 ) ;
#2009=DIRECTION ( 'NONE',  ( 0.000000000000000000, 0.000000000000000000, 1.000000000000000000 ) ) ;
#2010=EDGE_LOOP ( 'NONE', ( #40359, #25395, #54246, #10560 ) ) ;
#2017=EDGE_CURVE ( 'NONE', #53513, #46954, #10698, .T. ) ;
#2024=ORIENTED_EDGE ( 'NONE', *, *, #65884, .F. ) ;
#2026=VECTOR ( 'NONE', #28313, 1000.000000000000000 ) ;
#2028=LINE ( 'NONE', #13271, #49296 ) ;
#2030=VECTOR ( 'NONE', #4341, 1000.000000000000227 ) ;
#2031=CARTESIAN_POINT ( 'NONE',  ( 50.03867889673313130, 42.05760816978183669, 41.38025477438755928 ) ) ;
#2032=ORIENTED_EDGE ( 'NONE', *, *, #30523, .F. ) ;
#2037=DIRECTION ( 'NONE',  ( 1.000000000000000000, 0.000000000000000000, -0.000000000000000000 ) ) ;
#2039=DIRECTION ( 'NONE',  ( 1.000000000000000000, 0.000000000000000000, 0.000000000000000000 ) ) ;
#2042=VERTEX_POINT ( 'NONE', #47293 ) ;
#2050=LINE ( 'NONE', #45644, #44193 ) ;
#2052=VERTEX_POINT ( 'NONE', #36760 ) ;
#2061=ORIENTED_EDGE ( 'NONE', *, *, #33182, .T. ) ;
#2062=ORIENTED_EDGE ( 'NONE', *, *, #21925, .T. ) ;
#2064=CARTESIAN_POINT ( 'NONE',  ( -59.94154301275570162, 45.09516516490385385, 43.58025477438756212 ) ) ;
#2073=EDGE_CURVE ( 'NONE', #52786, #23236, #40804, .T. ) ;
#2074=VERTEX_POINT ( 'NONE', #55348 ) ;
#2077=DIRECTION ( 'NONE',  ( -0.000000000000000000, -0.000000000000000000, -1.000000000000000000 ) ) ;
#2078=VERTEX_POINT ( 'NONE', #44452 ) ;
#2081=VECTOR ( 'NONE', #29184, 1000.000000000000114 ) ;
#2082=DIRECTION ( 'NONE',  ( -0.9009688679024155933, -0.4338837391175656699, 0.000000000000000000 ) ) ;
#2085=CARTESIAN_POINT ( 'NONE',  ( 73.79471914489741380, -13.39176710989671726, 0.000000000000000000 ) ) ;
#2110=CARTESIAN_POINT ( 'NONE',  ( 15.68296563925591514, -63.09411298019745828, 170.0000000000000000 ) ) ;
#2117=DIRECTION ( 'NONE',  ( 0.4338837391175656699, -0.9009688679024155933, 2.500042656554809847E-16 ) ) ;
#2118=CARTESIAN_POINT ( 'NONE',  ( 34.76618902119740540, 54.93755186520760958, 170.0000000000000000 ) ) ;
#2142=ORIENTED_EDGE ( 'NONE', *, *, #4964, .F. ) ;
#2150=CARTESIAN_POINT ( 'NONE',  ( 19.62566184736079578, 15.48655536434876900, 0.000000000000000000 ) ) ;
#2151=FACE_OUTER_BOUND ( 'NONE', #2415, .T. ) ;
#2153=ADVANCED_FACE ( 'NONE', ( #50772 ), #39873, .F. ) ;
#2155=EDGE_CURVE ( 'NONE', #64382, #37468, #14528, .T. ) ;
#2190=EDGE_CURVE ( 'NONE', #41640, #36722, #58803, .T. ) ;
#2192=DIRECTION ( 'NONE',  ( -1.000000000000000000, 0.000000000000000000, 0.000000000000000000 ) ) ;
#2194=CARTESIAN_POINT ( 'NONE',  ( 0.000000000000000000, 0.000000000000000000, 133.5802547743875550 ) ) ;
#2197=AXIS2_PLACEMENT_3D ( 'NONE', #57678, #3864, #3179 ) ;
#2202=ORIENTED_EDGE ( 'NONE', *, *, #5625, .T. ) ;
#2204=VERTEX_POINT ( 'NONE', #69369 ) ;
#2212=AXIS2_PLACEMENT_3D ( 'NONE', #15468, #36921, #58360 ) ;
#2218=ADVANCED_FACE ( 'NONE', ( #5683 ), #9947, .F. ) ;
#2228=ORIENTED_EDGE ( 'NONE', *, *, #33111, .F. ) ;
#2245=ORIENTED_EDGE ( 'NONE', *, *, #24861, .F. ) ;
#2246=EDGE_CURVE ( 'NONE', #31208, #26272, #51977, .T. ) ;
#2252=EDGE_CURVE ( 'NONE', #18701, #68876, #20486, .T. ) ;
#2266=ORIENTED_EDGE ( 'NONE', *, *, #53514, .T. ) ;
#2274=CARTESIAN_POINT ( 'NONE',  ( 0.000000000000000000, 0.000000000000000000, 0.000000000000000000 ) ) ;
#2284=AXIS2_PLACEMENT_3D ( 'NONE', #40684, #4107, #3755 ) ;
#2289=EDGE_LOOP ( 'NONE', ( #44687, #20070, #18258, #6680 ) ) ;
#2290=ORIENTED_EDGE ( 'NONE', *, *, #17551, .F. ) ;
#2304=VERTEX_POINT ( 'NONE', #12717 ) ;
#2309=DIRECTION ( 'NONE',  ( 0.4738686624729966379, 0.8805955318567391110, 0.000000000000000000 ) ) ;
#2322=FACE_OUTER_BOUND ( 'NONE', #39212, .T. ) ;
#2323=ORIENTED_EDGE ( 'NONE', *, *, #38041, .F. ) ;
#2324=EDGE_CURVE ( 'NONE', #66023, #3025, #33490, .T. ) ;
#2326=EDGE_CURVE ( 'NONE', #19391, #30922, #18475, .T. ) ;
#2351=ORIENTED_EDGE ( 'NONE', *, *, #40585, .F. ) ;
#2353=CARTESIAN_POINT ( 'NONE',  ( -59.94154301275507635, -45.09516516490467808, 170.0000000000000000 ) ) ;
#2355=CARTESIAN_POINT ( 'NONE',  ( -65.36598343705435354, 0.000000000000000000, 41.38025477438755928 ) ) ;
#2359=ORIENTED_EDGE ( 'NONE', *, *, #8756, .T. ) ;
#2364=CARTESIAN_POINT ( 'NONE',  ( -72.57286576968782299, -18.73210786364450442, 41.38025477438755928 ) ) ;
#2377=ORIENTED_EDGE ( 'NONE', *, *, #20334, .T. ) ;
#2380=EDGE_CURVE ( 'NONE', #27926, #37383, #54205, .T. ) ;
#2386=DIRECTION ( 'NONE',  ( 1.000000000000000000, 0.000000000000000000, 0.000000000000000000 ) ) ;
#2393=VECTOR ( 'NONE', #37049, 1000.000000000000000 ) ;
#2399=CARTESIAN_POINT ( 'NONE',  ( 0.000000000000000000, 0.000000000000000000, 0.000000000000000000 ) ) ;
#2402=VERTEX_POINT ( 'NONE', #56664 ) ;
#2404=VERTEX_POINT ( 'NONE', #13411 ) ;
#2415=EDGE_LOOP ( 'NONE', ( #22354, #8411, #56637, #13834 ) ) ;
#2419=CARTESIAN_POINT ( 'NONE',  ( 20.79325243092023001, -13.87950479462515396, 0.000000000000000000 ) ) ;
#2423=PLANE ( 'NONE',  #28142 ) ;
#2424=ORIENTED_EDGE ( 'NONE', *, *, #44709, .F. ) ;
#2439=ORIENTED_EDGE ( 'NONE', *, *, #13053, .F. ) ;
#2444=EDGE_CURVE ( 'NONE', #13950, #58737, #55978, .T. ) ;
#2450=AXIS2_PLACEMENT_3D ( 'NONE', #32714, #5964, #27425 ) ;
#2452=ORIENTED_EDGE ( 'NONE', *, *, #16743, .T. ) ;
#2457=FACE_OUTER_BOUND ( 'NONE', #58163, .T. ) ;
#2465=LINE ( 'NONE', #61884, #68216 ) ;
#2471=CARTESIAN_POINT ( 'NONE',  ( -25.87147652227456263, 70.00000000000000000, 77.58025477438755502 ) ) ;
#2472=CARTESIAN_POINT ( 'NONE',  ( 0.000000000000000000, 0.000000000000000000, 40.00000000000003553 ) ) ;
#2491=VECTOR ( 'NONE', #11976, 1000.000000000000114 ) ;
#2496=VECTOR ( 'NONE', #42537, 1000.000000000000000 ) ;
#2499=DIRECTION ( 'NONE',  ( -1.000000000000000000, 0.000000000000000000, 0.000000000000000000 ) ) ;
#2508=DIRECTION ( 'NONE',  ( 1.000000000000000000, 0.000000000000000000, 0.000000000000000000 ) ) ;
#2514=EDGE_LOOP ( 'NONE', ( #42301, #32097, #17830, #68201, #41419, #24026, #6192, #42764, #12951 ) ) ;
#2516=CARTESIAN_POINT ( 'NONE',  ( 41.49663191311417165, -50.03028622612021792, 40.00000000000003553 ) ) ;
#2522=CARTESIAN_POINT ( 'NONE',  ( -3.120068508582665157, -41.61225602822255354, 13.79046340968177553 ) ) ;
#2525=CARTESIAN_POINT ( 'NONE',  ( 7.484861546145032740, 64.56761454192837846, 170.0000000000000000 ) ) ;
#2530=VERTEX_POINT ( 'NONE', #64348 ) ;
#2531=DIRECTION ( 'NONE',  ( -1.000000000000000000, 0.000000000000000000, 0.000000000000000000 ) ) ;
#2547=LINE ( 'NONE', #40867, #69041 ) ;
#2551=EDGE_CURVE ( 'NONE', #35639, #58973, #65437, .T. ) ;
#2556=EDGE_CURVE ( 'NONE', #10732, #61153, #15137, .T. ) ;
#2567=ORIENTED_EDGE ( 'NONE', *, *, #16266, .F. ) ;
#2591=LINE ( 'NONE', #61331, #12397 ) ;
#2592=DIRECTION ( 'NONE',  ( -1.000000000000000000, 0.000000000000000000, 0.000000000000000000 ) ) ;
#2599=VECTOR ( 'NONE', #20855, 1000.000000000000000 ) ;
#2615=VERTEX_POINT ( 'NONE', #44275 ) ;
#2619=LINE ( 'NONE', #39563, #860 ) ;
#2620=LINE ( 'NONE', #24085, #58061 ) ;
#2627=AXIS2_PLACEMENT_3D ( 'NONE', #18525, #51577, #23805 ) ;
#2628=PLANE ( 'NONE',  #6078 ) ;
#2632=ORIENTED_EDGE ( 'NONE', *, *, #31478, .F. ) ;
#2639=CARTESIAN_POINT ( 'NONE',  ( 11.70038220502452297, -40.05515866293553984, 13.79046340968177553 ) ) ;
#2652=CARTESIAN_POINT ( 'NONE',  ( -12.71198166530289342, -21.52685583500284139, 0.000000000000000000 ) ) ;
#2653=VECTOR ( 'NONE', #5003, 1000.000000000000114 ) ;
#2658=CARTESIAN_POINT ( 'NONE',  ( 0.000000000000000000, 0.000000000000000000, 41.38025477438755928 ) ) ;
#2665=ORIENTED_EDGE ( 'NONE', *, *, #60967, .F. ) ;
#2675=ORIENTED_EDGE ( 'NONE', *, *, #59329, .T. ) ;
#2676=EDGE_LOOP ( 'NONE', ( #13530, #3406, #22223, #37378, #48877, #45798, #46771, #41194, #5341 ) ) ;
#2685=VECTOR ( 'NONE', #29942, 1000.000000000000000 ) ;
#2693=CIRCLE ( 'NONE', #30760, 24.99999999999985434 ) ;
#2696=EDGE_CURVE ( 'NONE', #22856, #4959, #22574, .T. ) ;
#2698=AXIS2_PLACEMENT_3D ( 'NONE', #27431, #33074, #22512 ) ;
#2700=ADVANCED_FACE ( 'NONE', ( #39025 ), #49904, .T. ) ;
#2702=ORIENTED_EDGE ( 'NONE', *, *, #58656, .F. ) ;
#2705=PLANE ( 'NONE',  #8270 ) ;
#2714=ADVANCED_FACE ( 'NONE', ( #37969 ), #53779, .T. ) ;
#2719=ADVANCED_FACE ( 'NONE', ( #1377 ), #48841, .F. ) ;
#2729=VECTOR ( 'NONE', #44518, 1000.000000000000000 ) ;
#2737=VERTEX_POINT ( 'NONE', #59750 ) ;
#2743=DIRECTION ( 'NONE',  ( -1.000000000000000000, 0.000000000000000000, 0.000000000000000000 ) ) ;
#2746=CARTESIAN_POINT ( 'NONE',  ( -61.34830047412111043, 62.92641549729705019, 73.58025477438758344 ) ) ;
#2748=ORIENTED_EDGE ( 'NONE', *, *, #4984, .T. ) ;
#2749=ORIENTED_EDGE ( 'NONE', *, *, #60610, .F. ) ;
#2753=DIRECTION ( 'NONE',  ( 0.7530714660036195163, -0.6579387259397027066, 0.000000000000000000 ) ) ;
#2754=CARTESIAN_POINT ( 'NONE',  ( -41.50537345350708307, 50.04124777106294886, 170.0000000000000000 ) ) ;
#2770=ORIENTED_EDGE ( 'NONE', *, *, #33124, .F. ) ;
#2777=ORIENTED_EDGE ( 'NONE', *, *, #40056, .F. ) ;
#2778=CARTESIAN_POINT ( 'NONE',  ( 40.81683821231161602, -8.677580169988223346, 13.79046340968177731 ) ) ;
#2785=VERTEX_POINT ( 'NONE', #27754 ) ;
#2786=EDGE_CURVE ( 'NONE', #2737, #32221, #49196, .T. ) ;
#2788=CARTESIAN_POINT ( 'NONE',  ( -56.55682214211910974, -14.31196067865754173, 27.58472315868180402 ) ) ;
#2801=VERTEX_POINT ( 'NONE', #4074 ) ;
#2806=CARTESIAN_POINT ( 'NONE',  ( 10.06749493632391967, 74.32123213259514216, 43.58025477438756212 ) ) ;
#2807=ORIENTED_EDGE ( 'NONE', *, *, #46761, .T. ) ;
#2810=ORIENTED_EDGE ( 'NONE', *, *, #43574, .F. ) ;
#2813=ORIENTED_EDGE ( 'NONE', *, *, #33035, .F. ) ;
#2820=FACE_OUTER_BOUND ( 'NONE', #53008, .T. ) ;
#2827=ORIENTED_EDGE ( 'NONE', *, *, #13092, .F. ) ;
#2829=CARTESIAN_POINT ( 'NONE',  ( -52.69240448066660321, 53.30312580971368419, 41.38025477438755928 ) ) ;
#2835=AXIS2_PLACEMENT_3D ( 'NONE', #39813, #25639, #30556 ) ;
#2840=( GEOMETRIC_REPRESENTATION_CONTEXT ( 3 ) GLOBAL_UNCERTAINTY_ASSIGNED_CONTEXT ( ( #34628 ) ) GLOBAL_UNIT_ASSIGNED_CONTEXT ( ( #27587, #26214, #43758 ) ) REPRESENTATION_CONTEXT ( 'NONE', 'WORKASPACE' ) );
#2845=VERTEX_POINT ( 'NONE', #14956 ) ;
#2846=DIRECTION ( 'NONE',  ( 1.000000000000000000, 0.000000000000000000, 0.000000000000000000 ) ) ;
#2854=CARTESIAN_POINT ( 'NONE',  ( 0.000000000000000000, 0.000000000000000000, 40.82842712474622004 ) ) ;
#2861=DIRECTION ( 'NONE',  ( 1.000000000000000000, 0.000000000000000000, 0.000000000000000000 ) ) ;
#2866=PLANE ( 'NONE',  #1430 ) ;
#2868=CARTESIAN_POINT ( 'NONE',  ( -3.865535725358708596, -58.21137331173960661, 27.58472315868180402 ) ) ;
#2873=AXIS2_PLACEMENT_3D ( 'NONE', #2658, #40623, #50495 ) ;
#2875=EDGE_CURVE ( 'NONE', #42385, #61117, #18253, .T. ) ;
#2876=ORIENTED_EDGE ( 'NONE', *, *, #29372, .T. ) ;
#2877=ORIENTED_EDGE ( 'NONE', *, *, #26267, .F. ) ;
#2881=CARTESIAN_POINT ( 'NONE',  ( -62.66631205405160188, -18.59153367093452758, 43.58025477438756212 ) ) ;
#2913=ORIENTED_EDGE ( 'NONE', *, *, #469, .T. ) ;
#2928=AXIS2_PLACEMENT_3D ( 'NONE', #57417, #46861, #14505 ) ;
#2937=AXIS2_PLACEMENT_3D ( 'NONE', #60307, #49735, #55372 ) ;
#2938=VECTOR ( 'NONE', #32124, 1000.000000000000000 ) ;
#2945=EDGE_CURVE ( 'NONE', #18983, #62629, #43058, .T. ) ;
#2951=CARTESIAN_POINT ( 'NONE',  ( 64.97411640938653932, -37.36411256620218069, 41.38025477438755928 ) ) ;
#2977=EDGE_CURVE ( 'NONE', #2404, #30106, #39541, .T. ) ;
#2988=CARTESIAN_POINT ( 'NONE',  ( 7.484861546145933353, -64.56761454192826477, 40.00000000000003553 ) ) ;
#2989=CONICAL_SURFACE ( 'NONE', #27665, 74.95140232871122521, 0.8777644062502172329 ) ;
#2993=LINE ( 'NONE', #45893, #29240 ) ;
#2997=ORIENTED_EDGE ( 'NONE', *, *, #22900, .T. ) ;
#3004=ORIENTED_EDGE ( 'NONE', *, *, #29144, .F. ) ;
#3005=CARTESIAN_POINT ( 'NONE',  ( 0.000000000000000000, 0.000000000000000000, 170.0000000000000000 ) ) ;
#3016=VERTEX_POINT ( 'NONE', #7885 ) ;
#3018=DIRECTION ( 'NONE',  ( -0.000000000000000000, -0.000000000000000000, -1.000000000000000000 ) ) ;
#3019=DIRECTION ( 'NONE',  ( 1.000000000000000000, 0.000000000000000000, -0.000000000000000000 ) ) ;
#3025=VERTEX_POINT ( 'NONE', #49725 ) ;
#3032=VECTOR ( 'NONE', #4571, 1000.000000000000000 ) ;
#3046=CARTESIAN_POINT ( 'NONE',  ( 73.95984195137799588, -12.15131637179793955, 41.38025477438755928 ) ) ;
#3049=DIRECTION ( 'NONE',  ( -0.8584487936018655452, -0.5128992774059070170, 0.000000000000000000 ) ) ;
#3054=VERTEX_POINT ( 'NONE', #12118 ) ;
#3071=DIRECTION ( 'NONE',  ( 1.000000000000000000, 0.000000000000000000, 0.000000000000000000 ) ) ;
#3106=CARTESIAN_POINT ( 'NONE',  ( -37.04655464516766727, -53.85410457537912521, 6.377659838150125914E-18 ) ) ;
#3117=ORIENTED_EDGE ( 'NONE', *, *, #29794, .F. ) ;
#3128=CARTESIAN_POINT ( 'NONE',  ( -16.68907004672388084, 73.11959341363670717, 0.000000000000000000 ) ) ;
#3130=LINE ( 'NONE', #4162, #38433 ) ;
#3131=DIRECTION ( 'NONE',  ( 0.6234898018587318180, 0.7818314824680311359, 0.000000000000000000 ) ) ;
#3133=ORIENTED_EDGE ( 'NONE', *, *, #33675, .T. ) ;
#3134=B_SPLINE_CURVE_WITH_KNOTS ( 'NONE', 3,
 ( #16768, #10451, #59668, #21356, #53703, #11481 ),
 .UNSPECIFIED., .F., .F.,
 ( 4, 2, 4 ),
 ( 0.03218947840871073246, 0.06469842185262329737, 0.09720736529653584146 ),
 .UNSPECIFIED. ) ;
#3139=DIRECTION ( 'NONE',  ( -1.000000000000000000, 0.000000000000000000, 0.000000000000000000 ) ) ;
#3142=ORIENTED_EDGE ( 'NONE', *, *, #54067, .T. ) ;
#3148=ORIENTED_EDGE ( 'NONE', *, *, #20639, .T. ) ;
#3153=CONICAL_SURFACE ( 'NONE', #46918, 74.95140232871122521, 0.8777644062502172329 ) ;
#3155=ORIENTED_EDGE ( 'NONE', *, *, #17216, .F. ) ;
#3160=CARTESIAN_POINT ( 'NONE',  ( 0.000000000000000000, 0.000000000000000000, 40.00000000000003553 ) ) ;
#3163=ORIENTED_EDGE ( 'NONE', *, *, #53873, .F. ) ;
#3177=DIRECTION ( 'NONE',  ( -0.000000000000000000, -0.000000000000000000, -1.000000000000000000 ) ) ;
#3179=DIRECTION ( 'NONE',  ( -1.000000000000000000, 0.000000000000000000, 0.000000000000000000 ) ) ;
#3183=CARTESIAN_POINT ( 'NONE',  ( 34.76618902119824384, -54.93755186520707667, 170.0000000000000000 ) ) ;
#3187=EDGE_CURVE ( 'NONE', #40883, #22781, #424, .T. ) ;
#3190=CARTESIAN_POINT ( 'NONE',  ( 0.1230226671127766652, 25.12215469714594107, 0.000000000000000000 ) ) ;
#3197=CARTESIAN_POINT ( 'NONE',  ( 0.000000000000000000, 0.000000000000000000, 170.0010000000000048 ) ) ;
#3203=EDGE_CURVE ( 'NONE', #40013, #14673, #39651, .T. ) ;
#3211=DIRECTION ( 'NONE',  ( -0.000000000000000000, -0.000000000000000000, -1.000000000000000000 ) ) ;
#3214=ORIENTED_EDGE ( 'NONE', *, *, #44601, .T. ) ;
#3222=FACE_OUTER_BOUND ( 'NONE', #5487, .T. ) ;
#3230=VERTEX_POINT ( 'NONE', #37355 ) ;
#3239=B_SPLINE_CURVE_WITH_KNOTS ( 'NONE', 3,
 ( #58474, #37364, #5369, #786, #10287, #59165 ),
 .UNSPECIFIED., .F., .F.,
 ( 4, 2, 4 ),
 ( 1.095770181108577017E-06, 0.03239442681617711595, 0.06478775786217312593 ),
 .UNSPECIFIED. ) ;
#3247=ORIENTED_EDGE ( 'NONE', *, *, #55021, .F. ) ;
#3275=EDGE_LOOP ( 'NONE', ( #20431, #61803, #15637, #3793 ) ) ;
#3277=EDGE_LOOP ( 'NONE', ( #37757, #39085, #17297, #3492 ) ) ;
#3286=AXIS2_PLACEMENT_3D ( 'NONE', #22504, #42574, #16179 ) ;
#3292=VERTEX_POINT ( 'NONE', #53533 ) ;
#3303=CYLINDRICAL_SURFACE ( 'NONE', #9373, 65.00000000000000000 ) ;
#3306=ORIENTED_EDGE ( 'NONE', *, *, #52121, .F. ) ;
#3317=EDGE_LOOP ( 'NONE', ( #10425, #3809, #37410, #62214 ) ) ;
#3320=DIRECTION ( 'NONE',  ( -0.9009688679024155933, -0.4338837391175656699, 0.000000000000000000 ) ) ;
#3325=AXIS2_PLACEMENT_3D ( 'NONE', #33184, #21917, #38095 ) ;
#3326=DIRECTION ( 'NONE',  ( -0.6234898018587318180, -0.7818314824680311359, 0.000000000000000000 ) ) ;
#3334=EDGE_LOOP ( 'NONE', ( #10103, #31150, #43388, #49165 ) ) ;
#3345=VECTOR ( 'NONE', #10581, 1000.000000000000000 ) ;
#3348=CARTESIAN_POINT ( 'NONE',  ( 7.705763971469675511, -66.19838173227481093, 34.48241795236665297 ) ) ;
#3350=DIRECTION ( 'NONE',  ( 0.4738686624730094610, -0.8805955318567321166, 0.000000000000000000 ) ) ;
#3355=LINE ( 'NONE', #13564, #8173 ) ;
#3364=EDGE_CURVE ( 'NONE', #29619, #68173, #28557, .T. ) ;
#3378=CARTESIAN_POINT ( 'NONE',  ( 60.74750367560205433, 24.13405452624939329, 3.125053320693559764E-16 ) ) ;
#3382=ORIENTED_EDGE ( 'NONE', *, *, #57602, .T. ) ;
#3383=DIRECTION ( 'NONE',  ( -1.000000000000000000, 0.000000000000000000, 0.000000000000000000 ) ) ;
#3406=ORIENTED_EDGE ( 'NONE', *, *, #15857, .F. ) ;
#3409=CARTESIAN_POINT ( 'NONE',  ( -46.95151391448268896, 47.29862502947880643, 34.48241824012614387 ) ) ;
#3417=VERTEX_POINT ( 'NONE', #18005 ) ;
#3431=CARTESIAN_POINT ( 'NONE',  ( -41.31727360890708667, -62.59299402909810084, 43.58025477438756212 ) ) ;
#3433=ORIENTED_EDGE ( 'NONE', *, *, #31602, .T. ) ;
#3455=DIRECTION ( 'NONE',  ( 0.000000000000000000, 0.000000000000000000, -1.000000000000000000 ) ) ;
#3457=LINE ( 'NONE', #19631, #60271 ) ;
#3469=CARTESIAN_POINT ( 'NONE',  ( 24.46491470961361614, -5.710143558202974923, 0.000000000000000000 ) ) ;
#3479=DIRECTION ( 'NONE',  ( -0.000000000000000000, -0.000000000000000000, -1.000000000000000000 ) ) ;
#3489=CARTESIAN_POINT ( 'NONE',  ( 0.000000000000000000, 0.000000000000000000, 170.0000000000000000 ) ) ;
#3492=ORIENTED_EDGE ( 'NONE', *, *, #60667, .T. ) ;
#3501=ORIENTED_EDGE ( 'NONE', *, *, #36557, .F. ) ;
#3517=ORIENTED_EDGE ( 'NONE', *, *, #33458, .T. ) ;
#3523=ADVANCED_FACE ( 'NONE', ( #56675 ), #2866, .F. ) ;
#3537=CYLINDRICAL_SURFACE ( 'NONE', #63646, 65.00000000000000000 ) ;
#3538=VERTEX_POINT ( 'NONE', #8494 ) ;
#3552=CARTESIAN_POINT ( 'NONE',  ( -4.238248308523542285, -66.51046379052904456, 34.48241795236666718 ) ) ;
#3558=EDGE_CURVE ( 'NONE', #38399, #17506, #28422, .T. ) ;
#3560=ADVANCED_FACE ( 'NONE', ( #39678 ), #67728, .T. ) ;
#3564=CARTESIAN_POINT ( 'NONE',  ( 0.000000000000000000, 0.000000000000000000, 0.000000000000000000 ) ) ;
#3570=VERTEX_POINT ( 'NONE', #13307 ) ;
#3593=CARTESIAN_POINT ( 'NONE',  ( 73.57152302639893549, 14.62167909564604429, 170.0000000000000000 ) ) ;
#3624=ORIENTED_EDGE ( 'NONE', *, *, #9148, .T. ) ;
#3627=DIRECTION ( 'NONE',  ( -0.000000000000000000, -0.000000000000000000, -1.000000000000000000 ) ) ;
#3633=DIRECTION ( 'NONE',  ( 1.792759282944491616E-18, -4.776790026843708002E-18, -1.000000000000000000 ) ) ;
#3642=EDGE_CURVE ( 'NONE', #3054, #66077, #28394, .T. ) ;
#3643=AXIS2_PLACEMENT_3D ( 'NONE', #58333, #69236, #32312 ) ;
#3657=DIRECTION ( 'NONE',  ( -0.000000000000000000, -0.000000000000000000, -1.000000000000000000 ) ) ;
#3658=ORIENTED_EDGE ( 'NONE', *, *, #56244, .F. ) ;
#3662=CARTESIAN_POINT ( 'NONE',  ( -64.83840629396348731, 4.580509716059292913, 170.0000000000000000 ) ) ;
#3672=ORIENTED_EDGE ( 'NONE', *, *, #12701, .F. ) ;
#3678=EDGE_LOOP ( 'NONE', ( #22909, #31406, #7315, #35548, #23744, #13705, #14515, #10673, #19243 ) ) ;
#3681=CONICAL_SURFACE ( 'NONE', #16025, 65.00000000000000000, 0.7853981633974497223 ) ;
#3683=VECTOR ( 'NONE', #69513, 1000.000000000000000 ) ;
#3685=DIRECTION ( 'NONE',  ( 1.000000000000000000, 0.000000000000000000, -0.000000000000000000 ) ) ;
#3688=AXIS2_PLACEMENT_3D ( 'NONE', #57880, #42390, #47306 ) ;
#3697=LINE ( 'NONE', #61741, #36098 ) ;
#3698=VECTOR ( 'NONE', #49701, 1000.000000000000000 ) ;
#3710=CARTESIAN_POINT ( 'NONE',  ( -24.87827947785784133, 3.494138152041632583, 0.000000000000000000 ) ) ;
#3720=CARTESIAN_POINT ( 'NONE',  ( -56.44201257846587083, -32.26641783793643725, 41.38025477438755928 ) ) ;
#3727=ORIENTED_EDGE ( 'NONE', *, *, #39222, .F. ) ;
#3728=AXIS2_PLACEMENT_3D ( 'NONE', #49624, #7078, #1816 ) ;
#3730=EDGE_CURVE ( 'NONE', #40116, #20254, #63256, .T. ) ;
#3731=CARTESIAN_POINT ( 'NONE',  ( 48.11816970607237209, 43.69944786994017250, 40.00000000000003553 ) ) ;
#3736=VERTEX_POINT ( 'NONE', #33589 ) ;
#3737=CIRCLE ( 'NONE', #64433, 10.00000000000000000 ) ;
#3741=B_SPLINE_CURVE_WITH_KNOTS ( 'NONE', 3,
 ( #26161, #58495, #46573, #63103 ),
 .UNSPECIFIED., .F., .F.,
 ( 4, 4 ),
 ( 0.1259919275528360028, 0.1829744153748751323 ),
 .UNSPECIFIED. ) ;
#3755=DIRECTION ( 'NONE',  ( -1.000000000000000000, 0.000000000000000000, 0.000000000000000000 ) ) ;
#3757=CARTESIAN_POINT ( 'NONE',  ( 0.000000000000000000, 0.000000000000000000, 40.00000000000003553 ) ) ;
#3758=ORIENTED_EDGE ( 'NONE', *, *, #8617, .T. ) ;
#3760=ORIENTED_EDGE ( 'NONE', *, *, #30873, .F. ) ;
#3762=DIRECTION ( 'NONE',  ( -1.000000000000000000, 0.000000000000000000, 0.000000000000000000 ) ) ;
#3765=ORIENTED_EDGE ( 'NONE', *, *, #65097, .T. ) ;
#3768=ORIENTED_EDGE ( 'NONE', *, *, #68082, .T. ) ;
#3769=CYLINDRICAL_SURFACE ( 'NONE', #69250, 65.00000000000000000 ) ;
#3773=CARTESIAN_POINT ( 'NONE',  ( -71.90777365577140756, 21.14201501538314076, 41.38025477438755928 ) ) ;
#3780=CARTESIAN_POINT ( 'NONE',  ( -31.90315521289150524, 56.64813493366005304, 43.58025477438756923 ) ) ;
#3785=CARTESIAN_POINT ( 'NONE',  ( -72.62976060914719767, -18.74780984163136566, 170.0000000000000000 ) ) ;
#3788=FACE_OUTER_BOUND ( 'NONE', #19947, .T. ) ;
#3793=ORIENTED_EDGE ( 'NONE', *, *, #13114, .T. ) ;
#3796=VECTOR ( 'NONE', #59516, 1000.000000000000000 ) ;
#3798=EDGE_LOOP ( 'NONE', ( #4231, #15355, #58430, #58254 ) ) ;
#3800=DIRECTION ( 'NONE',  ( -0.9639628606958512425, -0.2660368455666826670, 0.000000000000000000 ) ) ;
#3806=DIRECTION ( 'NONE',  ( -0.000000000000000000, -0.000000000000000000, -1.000000000000000000 ) ) ;
#3809=ORIENTED_EDGE ( 'NONE', *, *, #30277, .F. ) ;
#3818=ADVANCED_FACE ( 'NONE', ( #1217 ), #1932, .T. ) ;
#3819=ORIENTED_EDGE ( 'NONE', *, *, #66204, .F. ) ;
#3830=CARTESIAN_POINT ( 'NONE',  ( 73.95984195137785377, 12.15131637179898583, 41.38025477438755928 ) ) ;
#3831=VECTOR ( 'NONE', #5641, 1000.000000000000114 ) ;
#3845=ORIENTED_EDGE ( 'NONE', *, *, #1380, .F. ) ;
#3852=AXIS2_PLACEMENT_3D ( 'NONE', #4188, #25656, #42829 ) ;
#3858=VERTEX_POINT ( 'NONE', #65592 ) ;
#3859=CARTESIAN_POINT ( 'NONE',  ( 28.73969596345624211, -50.76944258518214070, 27.58472369392173107 ) ) ;
#3863=CARTESIAN_POINT ( 'NONE',  ( 53.32245423372562243, 37.19594572654711584, 3.061616997868437868E-16 ) ) ;
#3864=DIRECTION ( 'NONE',  ( -0.000000000000000000, -0.000000000000000000, -1.000000000000000000 ) ) ;
#3871=CARTESIAN_POINT ( 'NONE',  ( -40.24154210098803475, 63.23235722614447951, 41.38025477438755928 ) ) ;
#3874=PLANE ( 'NONE',  #706 ) ;
#3875=DIRECTION ( 'NONE',  ( -0.000000000000000000, 0.000000000000000000, -1.000000000000000000 ) ) ;
#3882=CARTESIAN_POINT ( 'NONE',  ( 0.000000000000000000, 0.000000000000000000, 0.000000000000000000 ) ) ;
#3885=DIRECTION ( 'NONE',  ( -0.04486483035050447404, -0.9989930665413151445, 0.000000000000000000 ) ) ;
#3894=EDGE_LOOP ( 'NONE', ( #61364, #1472, #45906, #56335 ) ) ;
#3897=ADVANCED_FACE ( 'NONE', ( #56414 ), #3303, .T. ) ;
#3903=CIRCLE ( 'NONE', #523, 65.36598343705435354 ) ;
#3920=EDGE_CURVE ( 'NONE', #35022, #39565, #636, .T. ) ;
#3921=B_SPLINE_CURVE_WITH_KNOTS ( 'NONE', 3,
 ( #27555, #33895, #6801, #18755, #66959, #33557 ),
 .UNSPECIFIED., .F., .F.,
 ( 4, 2, 4 ),
 ( 0.03218945466321621734, 0.06469840457090983432, 0.09720735447860343048 ),
 .UNSPECIFIED. ) ;
#3924=EDGE_CURVE ( 'NONE', #671, #69067, #51148, .T. ) ;
#3925=CARTESIAN_POINT ( 'NONE',  ( 13.24564585880136036, -63.65041531508826012, 170.0000000000000000 ) ) ;
#3930=AXIS2_PLACEMENT_3D ( 'NONE', #64672, #21748, #44244 ) ;
#3936=CARTESIAN_POINT ( 'NONE',  ( 55.65793654284613012, 50.28674377798307660, 43.58025477438756923 ) ) ;
#3938=CIRCLE ( 'NONE', #23016, 65.00000000000000000 ) ;
#3940=VERTEX_POINT ( 'NONE', #13851 ) ;
#3941=CONICAL_SURFACE ( 'NONE', #67971, 74.95140232871122521, 0.8777644062502172329 ) ;
#3960=CARTESIAN_POINT ( 'NONE',  ( -10.96274578891745755, -22.46815979931523799, 0.000000000000000000 ) ) ;
#3964=EDGE_CURVE ( 'NONE', #11003, #3736, #67338, .T. ) ;
#3971=DIRECTION ( 'NONE',  ( -1.000000000000000000, 0.000000000000000000, 0.000000000000000000 ) ) ;
#3974=CARTESIAN_POINT ( 'NONE',  ( -15.67984581961064450, 63.08044415722863363, 170.0000000000000000 ) ) ;
#3983=DIRECTION ( 'NONE',  ( 0.8584487936018728726, -0.5128992774058949156, 0.000000000000000000 ) ) ;
#3985=EDGE_CURVE ( 'NONE', #26979, #34764, #36288, .T. ) ;
#3986=EDGE_CURVE ( 'NONE', #49220, #59826, #14882, .T. ) ;
#3991=AXIS2_PLACEMENT_3D ( 'NONE', #255, #64636, #38596 ) ;
#3994=CARTESIAN_POINT ( 'NONE',  ( 0.000000000000000000, 0.000000000000000000, 40.00000000000003553 ) ) ;
#4001=ORIENTED_EDGE ( 'NONE', *, *, #55018, .T. ) ;
#4004=CARTESIAN_POINT ( 'NONE',  ( -1.368053087914143706, -58.32353603131943487, 27.58472369367942889 ) ) ;
#4019=PLANE ( 'NONE',  #57823 ) ;
#4030=CARTESIAN_POINT ( 'NONE',  ( 0.000000000000000000, 0.000000000000000000, 0.000000000000000000 ) ) ;
#4035=VERTEX_POINT ( 'NONE', #68691 ) ;
#4040=DIRECTION ( 'NONE',  ( -0.000000000000000000, -0.000000000000000000, -1.000000000000000000 ) ) ;
#4042=PRODUCT_DEFINITION_FORMATION_WITH_SPECIFIED_SOURCE ( 'ANY', '', #51893, .NOT_KNOWN. ) ;
#4047=LINE ( 'NONE', #20909, #68127 ) ;
#4049=VECTOR ( 'NONE', #11638, 1000.000000000000000 ) ;
#4051=DIRECTION ( 'NONE',  ( 0.000000000000000000, 0.000000000000000000, 1.000000000000000000 ) ) ;
#4066=DIRECTION ( 'NONE',  ( -0.000000000000000000, -0.000000000000000000, -1.000000000000000000 ) ) ;
#4072=B_SPLINE_CURVE_WITH_KNOTS ( 'NONE', 3,
 ( #48225, #37009, #48565, #51 ),
 .UNSPECIFIED., .F., .F.,
 ( 4, 4 ),
 ( 9.900409499089635938E-07, 0.05658314289920116785 ),
 .UNSPECIFIED. ) ;
#4074=CARTESIAN_POINT ( 'NONE',  ( -24.75616454008739709, -3.483147608717210630, 0.000000000000000000 ) ) ;
#4077=VERTEX_POINT ( 'NONE', #69027 ) ;
#4078=PLANE ( 'NONE',  #3688 ) ;
#4089=CARTESIAN_POINT ( 'NONE',  ( 23.63370729589335184, -52.11334794818031924, 133.5802547743875550 ) ) ;
#4090=CARTESIAN_POINT ( 'NONE',  ( -12.77952633087662093, -21.62918162951127243, 3.061616997868437868E-16 ) ) ;
#4095=CIRCLE ( 'NONE', #6335, 65.36598343705435354 ) ;
#4103=EDGE_LOOP ( 'NONE', ( #11564, #8330, #38539, #59538 ) ) ;
#4107=DIRECTION ( 'NONE',  ( -0.000000000000000000, -0.000000000000000000, -1.000000000000000000 ) ) ;
#4108=DIRECTION ( 'NONE',  ( -0.000000000000000000, -0.000000000000000000, 1.000000000000000000 ) ) ;
#4109=DIRECTION ( 'NONE',  ( -1.000000000000000000, 0.000000000000000000, 0.000000000000000000 ) ) ;
#4111=DIRECTION ( 'NONE',  ( -0.000000000000000000, -0.000000000000000000, -1.000000000000000000 ) ) ;
#4113=ORIENTED_EDGE ( 'NONE', *, *, #40667, .T. ) ;
#4121=EDGE_LOOP ( 'NONE', ( #15370, #59184, #63446, #6452 ) ) ;
#4127=CARTESIAN_POINT ( 'NONE',  ( -23.85457283326439182, 7.880174245944055578, 0.000000000000000000 ) ) ;
#4129=ORIENTED_EDGE ( 'NONE', *, *, #4673, .T. ) ;
#4137=CARTESIAN_POINT ( 'NONE',  ( 61.28323125814129213, -21.66484633135379667, 40.00000000000003553 ) ) ;
#4139=FACE_OUTER_BOUND ( 'NONE', #54207, .T. ) ;
#4144=ORIENTED_EDGE ( 'NONE', *, *, #53038, .F. ) ;
#4153=CARTESIAN_POINT ( 'NONE',  ( 70.60157554497493493, -25.16207943727098950, 41.38025477438755928 ) ) ;
#4158=DIRECTION ( 'NONE',  ( -1.000000000000000000, 0.000000000000000000, 0.000000000000000000 ) ) ;
#4160=CARTESIAN_POINT ( 'NONE',  ( -23.14886993799567705, -9.760512885997105315, 0.000000000000000000 ) ) ;
#4162=CARTESIAN_POINT ( 'NONE',  ( 74.39890044415633952, 7.951074708187157114, 170.0000000000000000 ) ) ;
#4171=CARTESIAN_POINT ( 'NONE',  ( -13.24252603915519444, -63.63674649211960599, 170.0000000000000000 ) ) ;
#4180=CARTESIAN_POINT ( 'NONE',  ( 0.000000000000000000, 0.000000000000000000, 43.58025477438756212 ) ) ;
#4182=ORIENTED_EDGE ( 'NONE', *, *, #46122, .F. ) ;
#4188=CARTESIAN_POINT ( 'NONE',  ( 0.000000000000000000, 0.000000000000000000, 0.000000000000000000 ) ) ;
#4191=EDGE_CURVE ( 'NONE', #55532, #38915, #26137, .T. ) ;
#4200=DIRECTION ( 'NONE',  ( 0.000000000000000000, 0.000000000000000000, 1.000000000000000000 ) ) ;
#4206=FACE_OUTER_BOUND ( 'NONE', #56753, .T. ) ;
#4209=FACE_OUTER_BOUND ( 'NONE', #6614, .T. ) ;
#4210=ORIENTED_EDGE ( 'NONE', *, *, #53344, .T. ) ;
#4222=FACE_OUTER_BOUND ( 'NONE', #2289, .T. ) ;
#4226=CARTESIAN_POINT ( 'NONE',  ( 37.34307124463426675, -44.82188588777072624, 27.58472369417913583 ) ) ;
#4228=ORIENTED_EDGE ( 'NONE', *, *, #11749, .T. ) ;
#4231=ORIENTED_EDGE ( 'NONE', *, *, #26052, .T. ) ;
#4236=CARTESIAN_POINT ( 'NONE',  ( 0.000000000000000000, 0.000000000000000000, 40.00000000000003553 ) ) ;
#4239=EDGE_CURVE ( 'NONE', #2530, #28747, #69404, .T. ) ;
#4240=EDGE_CURVE ( 'NONE', #40678, #25506, #42573, .T. ) ;
#4243=DIRECTION ( 'NONE',  ( -1.000000000000000000, 0.000000000000000000, 0.000000000000000000 ) ) ;
#4245=CARTESIAN_POINT ( 'NONE',  ( 16.83496191631032346, 55.85777011067597897, 27.58472369377037481 ) ) ;
#4261=DIRECTION ( 'NONE',  ( -0.9639628606958550172, 0.2660368455666687892, 0.000000000000000000 ) ) ;
#4262=ORIENTED_EDGE ( 'NONE', *, *, #58288, .T. ) ;
#4267=CARTESIAN_POINT ( 'NONE',  ( 29.31537786019797664, 16.05900809008567975, 6.893343212288939093 ) ) ;
#4282=VECTOR ( 'NONE', #5457, 1000.000000000000114 ) ;
#4283=VERTEX_POINT ( 'NONE', #4938 ) ;
#4289=EDGE_CURVE ( 'NONE', #66440, #49450, #4845, .T. ) ;
#4290=EDGE_CURVE ( 'NONE', #36739, #40678, #341, .T. ) ;
#4297=EDGE_CURVE ( 'NONE', #24824, #66237, #10464, .T. ) ;
#4299=DIRECTION ( 'NONE',  ( -0.000000000000000000, -0.000000000000000000, -1.000000000000000000 ) ) ;
#4301=DIRECTION ( 'NONE',  ( -0.000000000000000000, -0.000000000000000000, -1.000000000000000000 ) ) ;
#4304=DIRECTION ( 'NONE',  ( -1.000000000000000000, 0.000000000000000000, 0.000000000000000000 ) ) ;
#4309=CARTESIAN_POINT ( 'NONE',  ( -23.70047331481904251, -76.98764151615553430, 133.5802547743875550 ) ) ;
#4312=ORIENTED_EDGE ( 'NONE', *, *, #17546, .T. ) ;
#4320=FACE_OUTER_BOUND ( 'NONE', #58122, .T. ) ;
#4323=DIRECTION ( 'NONE',  ( 1.000000000000000000, 0.000000000000000000, -0.000000000000000000 ) ) ;
#4330=ORIENTED_EDGE ( 'NONE', *, *, #55674, .F. ) ;
#4331=VECTOR ( 'NONE', #69217, 1000.000000000000000 ) ;
#4341=DIRECTION ( 'NONE',  ( 0.5508969814520944253, 0.8345732537213078617, -0.000000000000000000 ) ) ;
#4346=DIRECTION ( 'NONE',  ( -1.000000000000000000, 0.000000000000000000, 0.000000000000000000 ) ) ;
#4347=DIRECTION ( 'NONE',  ( -1.000000000000000000, 0.000000000000000000, 0.000000000000000000 ) ) ;
#4349=CARTESIAN_POINT ( 'NONE',  ( -6.774725108395606377, -24.06456107444444825, 0.000000000000000000 ) ) ;
#4350=DIRECTION ( 'NONE',  ( -0.3930250316539278255, 0.9195277725514487965, 0.000000000000000000 ) ) ;
#4354=CARTESIAN_POINT ( 'NONE',  ( -4.164416015344989397, -64.86646004871190030, 170.0000000000000000 ) ) ;
#4366=CARTESIAN_POINT ( 'NONE',  ( 24.39800339187844003, 60.26242556095705538, 41.38025477438755928 ) ) ;
#4369=CARTESIAN_POINT ( 'NONE',  ( 0.000000000000000000, 0.000000000000000000, 41.38025477438755928 ) ) ;
#4375=EDGE_CURVE ( 'NONE', #56665, #43797, #55551, .T. ) ;
#4382=ORIENTED_EDGE ( 'NONE', *, *, #4520, .T. ) ;
#4383=VERTEX_POINT ( 'NONE', #34811 ) ;
#4393=ORIENTED_EDGE ( 'NONE', *, *, #4520, .F. ) ;
#4401=ADVANCED_FACE ( 'NONE', ( #14035 ), #66831, .F. ) ;
#4402=CARTESIAN_POINT ( 'NONE',  ( 1.667562369267758360, -64.99262834925670518, 43.58025477438756923 ) ) ;
#4406=DIRECTION ( 'NONE',  ( -1.000000000000000000, 0.000000000000000000, 0.000000000000000000 ) ) ;
#4412=CYLINDRICAL_SURFACE ( 'NONE', #21049, 65.00000000000000000 ) ;
#4416=CARTESIAN_POINT ( 'NONE',  ( 16.92909711280922735, 28.82167224275331208, 6.893343212288921329 ) ) ;
#4418=DIRECTION ( 'NONE',  ( -1.000000000000000000, 0.000000000000000000, 0.000000000000000000 ) ) ;
#4419=CARTESIAN_POINT ( 'NONE',  ( -13.24252603915608617, 63.63674649211943546, 133.5802547743875550 ) ) ;
#4423=EDGE_LOOP ( 'NONE', ( #51163, #12212, #67956, #68008 ) ) ;
#4427=CARTESIAN_POINT ( 'NONE',  ( -17.35806700812657155, -28.56537427343508995, 6.893342935626296963 ) ) ;
#4440=DIRECTION ( 'NONE',  ( -1.000000000000000000, 0.000000000000000000, 0.000000000000000000 ) ) ;
#4444=CARTESIAN_POINT ( 'NONE',  ( -25.87147652227456263, 70.00000000000000000, 129.5802547743875550 ) ) ;
#4456=EDGE_CURVE ( 'NONE', #7966, #64522, #50106, .T. ) ;
#4462=DIRECTION ( 'NONE',  ( 1.156482317317871478E-16, 0.000000000000000000, 1.000000000000000000 ) ) ;
#4463=AXIS2_PLACEMENT_3D ( 'NONE', #8026, #23865, #29827 ) ;
#4465=VERTEX_POINT ( 'NONE', #38962 ) ;
#4477=CIRCLE ( 'NONE', #13469, 25.12245591505646303 ) ;
#4485=PLANE ( 'NONE',  #61384 ) ;
#4488=PLANE ( 'NONE',  #10493 ) ;
#4491=CARTESIAN_POINT ( 'NONE',  ( -67.03031041878467988, 33.66749151869449008, 170.0000000000000000 ) ) ;
#4495=VECTOR ( 'NONE', #58359, 1000.000000000000227 ) ;
#4497=EDGE_LOOP ( 'NONE', ( #21687, #30146, #44935, #48645 ) ) ;
#4500=CARTESIAN_POINT ( 'NONE',  ( 64.98797965777978902, -1.250000000000021094, 170.0000000000000000 ) ) ;
#4501=CARTESIAN_POINT ( 'NONE',  ( -27.92096271590487788, -31.01184599629533167, 13.79046412439886460 ) ) ;
#4518=EDGE_CURVE ( 'NONE', #28008, #68407, #60749, .T. ) ;
#4520=EDGE_CURVE ( 'NONE', #9355, #65052, #29182, .T. ) ;
#4528=CARTESIAN_POINT ( 'NONE',  ( -21.27554331372911278, -61.43430442924894663, 41.38025477438755928 ) ) ;
#4529=VECTOR ( 'NONE', #51177, 1000.000000000000000 ) ;
#4530=VERTEX_POINT ( 'NONE', #44576 ) ;
#4543=VERTEX_POINT ( 'NONE', #5882 ) ;
#4545=DIRECTION ( 'NONE',  ( -0.04486483035051862939, 0.9989930665413143673, 0.000000000000000000 ) ) ;
#4553=VECTOR ( 'NONE', #17826, 1000.000000000000000 ) ;
#4562=CARTESIAN_POINT ( 'NONE',  ( -15.45727656667689409, 73.34020256436167529, 41.38025477438755928 ) ) ;
#4569=LINE ( 'NONE', #30280, #63057 ) ;
#4571=DIRECTION ( 'NONE',  ( -0.8090169943749422332, -0.5877852522924802425, 0.000000000000000000 ) ) ;
#4575=CARTESIAN_POINT ( 'NONE',  ( 0.000000000000000000, 0.000000000000000000, 0.000000000000000000 ) ) ;
#4577=VERTEX_POINT ( 'NONE', #23126 ) ;
#4582=CARTESIAN_POINT ( 'NONE',  ( -26.28838124991334979, 20.64471194235530049, 6.893343212288937316 ) ) ;
#4592=DIRECTION ( 'NONE',  ( -0.000000000000000000, -0.000000000000000000, -1.000000000000000000 ) ) ;
#4603=AXIS2_PLACEMENT_3D ( 'NONE', #54725, #6552, #6195 ) ;
#4606=CARTESIAN_POINT ( 'NONE',  ( 11.30618213853490239, -74.15344055032291237, 170.0000000000000000 ) ) ;
#4608=ORIENTED_EDGE ( 'NONE', *, *, #19669, .T. ) ;
#4612=ORIENTED_EDGE ( 'NONE', *, *, #31145, .F. ) ;
#4619=ORIENTED_EDGE ( 'NONE', *, *, #21593, .T. ) ;
#4620=DIRECTION ( 'NONE',  ( 0.9839295885986295565, 0.1785568947986370392, 0.000000000000000000 ) ) ;
#4621=LINE ( 'NONE', #59459, #61269 ) ;
#4622=LINE ( 'NONE', #38017, #64786 ) ;
#4625=CARTESIAN_POINT ( 'NONE',  ( -13.24252603915608617, 63.63674649211943546, 40.00000000000003553 ) ) ;
#4628=CARTESIAN_POINT ( 'NONE',  ( 47.91750368872954624, -19.31887499200363223, 26.66469104408689006 ) ) ;
#4639=VECTOR ( 'NONE', #59498, 1000.000000000000114 ) ;
#4642=ORIENTED_EDGE ( 'NONE', *, *, #18650, .T. ) ;
#4645=ORIENTED_EDGE ( 'NONE', *, *, #62722, .F. ) ;
#4655=LINE ( 'NONE', #26116, #55110 ) ;
#4671=ADVANCED_FACE ( 'NONE', ( #46909 ), #52095, .T. ) ;
#4673=EDGE_CURVE ( 'NONE', #3292, #41626, #41975, .T. ) ;
#4678=VECTOR ( 'NONE', #35673, 1000.000000000000114 ) ;
#4681=EDGE_CURVE ( 'NONE', #64121, #16854, #19506, .T. ) ;
#4686=ORIENTED_EDGE ( 'NONE', *, *, #66109, .F. ) ;
#4694=CARTESIAN_POINT ( 'NONE',  ( -50.92620509423012720, -55.07344309828840068, 170.0000000000000000 ) ) ;
#4696=VERTEX_POINT ( 'NONE', #32805 ) ;
#4698=DIRECTION ( 'NONE',  ( -0.000000000000000000, -0.000000000000000000, -1.000000000000000000 ) ) ;
#4714=CARTESIAN_POINT ( 'NONE',  ( 74.39890044415652426, -7.951074708186050444, 170.0000000000000000 ) ) ;
#4725=ORIENTED_EDGE ( 'NONE', *, *, #60038, .T. ) ;
#4733=CARTESIAN_POINT ( 'NONE',  ( -68.06184294702747195, 31.38946074233368222, 41.38025477438755928 ) ) ;
#4738=VERTEX_POINT ( 'NONE', #6056 ) ;
#4741=CARTESIAN_POINT ( 'NONE',  ( -63.73419499958998813, 12.83646726144838013, 41.38025477438755928 ) ) ;
#4745=DIRECTION ( 'NONE',  ( -0.000000000000000000, -0.000000000000000000, -1.000000000000000000 ) ) ;
#4748=ORIENTED_EDGE ( 'NONE', *, *, #50280, .T. ) ;
#4754=PLANE ( 'NONE',  #29745 ) ;
#4756=CARTESIAN_POINT ( 'NONE',  ( 63.72039997003725631, -12.83396383267754537, 40.00000000000003553 ) ) ;
#4758=DIRECTION ( 'NONE',  ( 0.9510565162951500895, 0.3090169943749583314, 2.500042656554809847E-16 ) ) ;
#4761=EDGE_CURVE ( 'NONE', #28769, #14491, #60577, .T. ) ;
#4770=EDGE_LOOP ( 'NONE', ( #62843, #29806, #13390, #1354 ) ) ;
#4776=DIRECTION ( 'NONE',  ( -2.616877698022195692E-18, -4.379915515250404077E-18, -1.000000000000000000 ) ) ;
#4780=ADVANCED_FACE ( 'NONE', ( #33159 ), #1143, .T. ) ;
#4783=CIRCLE ( 'NONE', #63194, 65.36598343705435354 ) ;
#4787=DIRECTION ( 'NONE',  ( -0.000000000000000000, -0.000000000000000000, -1.000000000000000000 ) ) ;
#4788=ORIENTED_EDGE ( 'NONE', *, *, #53257, .F. ) ;
#4793=LINE ( 'NONE', #26258, #10044 ) ;
#4806=ORIENTED_EDGE ( 'NONE', *, *, #27448, .F. ) ;
#4820=EDGE_LOOP ( 'NONE', ( #62298, #10740, #2877, #36069, #7715, #7144, #60896, #28446, #21234 ) ) ;
#4824=CARTESIAN_POINT ( 'NONE',  ( 14.66690460840507804, -20.39656099473392814, 0.000000000000000000 ) ) ;
#4828=DIRECTION ( 'NONE',  ( 4.974206872490772509E-18, 1.135330258912677140E-18, -1.000000000000000000 ) ) ;
#4835=DIRECTION ( 'NONE',  ( 0.1342332658176667304, -0.9909497617679331460, 0.000000000000000000 ) ) ;
#4845=CIRCLE ( 'NONE', #31809, 74.95140232871122521 ) ;
#4857=LINE ( 'NONE', #42492, #4331 ) ;
#4862=ORIENTED_EDGE ( 'NONE', *, *, #45702, .F. ) ;
#4863=LINE ( 'NONE', #16793, #36809 ) ;
#4866=DIRECTION ( 'NONE',  ( -0.3090169943749447312, -0.9510565162951544194, 0.000000000000000000 ) ) ;
#4879=FACE_OUTER_BOUND ( 'NONE', #7002, .T. ) ;
#4884=VECTOR ( 'NONE', #12771, 999.9999999999998863 ) ;
#4891=VERTEX_POINT ( 'NONE', #9893 ) ;
#4896=CARTESIAN_POINT ( 'NONE',  ( 36.64089410029568228, 65.45232906116417837, 43.58025477438756212 ) ) ;
#4902=CARTESIAN_POINT ( 'NONE',  ( -51.82969867401513397, 54.20961478705410030, 43.58025477438756212 ) ) ;
#4905=CARTESIAN_POINT ( 'NONE',  ( 63.00000000000000000, 7.715274834628325378E-15, 170.0000000000000000 ) ) ;
#4906=ORIENTED_EDGE ( 'NONE', *, *, #35345, .F. ) ;
#4908=EDGE_CURVE ( 'NONE', #37858, #36451, #7392, .T. ) ;
#4909=EDGE_LOOP ( 'NONE', ( #310, #34298, #9189, #55164 ) ) ;
#4917=EDGE_LOOP ( 'NONE', ( #61243, #18481, #55829, #16565 ) ) ;
#4920=ORIENTED_EDGE ( 'NONE', *, *, #2190, .T. ) ;
#4922=CARTESIAN_POINT ( 'NONE',  ( 0.000000000000000000, 0.000000000000000000, 0.000000000000000000 ) ) ;
#4925=DIRECTION ( 'NONE',  ( 1.000000000000000000, 0.000000000000000000, 0.000000000000000000 ) ) ;
#4928=EDGE_CURVE ( 'NONE', #9934, #23357, #60498, .T. ) ;
#4930=CIRCLE ( 'NONE', #44230, 10.00000000000000000 ) ;
#4931=EDGE_LOOP ( 'NONE', ( #41920, #43256, #8121, #49854, #5742, #37890, #29263, #26525, #1154 ) ) ;
#4936=CONICAL_SURFACE ( 'NONE', #1573, 74.95140232871122521, 0.8777644062502172329 ) ;
#4938=CARTESIAN_POINT ( 'NONE',  ( -12.77952633087691403, 21.62918162951106993, 0.000000000000000000 ) ) ;
#4939=CIRCLE ( 'NONE', #12784, 65.36598343705435354 ) ;
#4940=DIRECTION ( 'NONE',  ( -0.9639628606958550172, 0.2660368455666687892, 0.000000000000000000 ) ) ;
#4942=DIRECTION ( 'NONE',  ( -0.000000000000000000, -0.000000000000000000, -1.000000000000000000 ) ) ;
#4952=CARTESIAN_POINT ( 'NONE',  ( 49.76301652092226391, -41.81676920493045202, 40.00000000000003553 ) ) ;
#4959=VERTEX_POINT ( 'NONE', #27791 ) ;
#4964=EDGE_CURVE ( 'NONE', #5356, #3417, #49229, .T. ) ;
#4973=AXIS2_PLACEMENT_3D ( 'NONE', #13671, #50611, #3131 ) ;
#4979=DIRECTION ( 'NONE',  ( -0.8584487936018655452, -0.5128992774059070170, 0.000000000000000000 ) ) ;
#4984=EDGE_CURVE ( 'NONE', #12323, #24023, #34483, .T. ) ;
#4991=CARTESIAN_POINT ( 'NONE',  ( -7.306921717852591591, 37.63116478967256739, 13.32819397642332504 ) ) ;
#5003=DIRECTION ( 'NONE',  ( 0.7693125429406515448, 0.000000000000000000, 0.6388726095820577155 ) ) ;
#5004=ORIENTED_EDGE ( 'NONE', *, *, #35996, .T. ) ;
#5009=EDGE_CURVE ( 'NONE', #33759, #34668, #37367, .T. ) ;
#5028=VECTOR ( 'NONE', #63305, 1000.000000000000000 ) ;
#5039=CARTESIAN_POINT ( 'NONE',  ( 0.000000000000000000, 0.000000000000000000, 41.38025477438755928 ) ) ;
#5048=ADVANCED_FACE ( 'NONE', ( #2457 ), #65562, .T. ) ;
#5051=FACE_OUTER_BOUND ( 'NONE', #45723, .T. ) ;
#5055=LINE ( 'NONE', #32486, #53418 ) ;
#5057=ORIENTED_EDGE ( 'NONE', *, *, #30929, .F. ) ;
#5063=EDGE_CURVE ( 'NONE', #29619, #53557, #1407, .T. ) ;
#5065=DIRECTION ( 'NONE',  ( -0.4338837391175656699, 0.9009688679024155933, 5.102127870520019688E-18 ) ) ;
#5070=ORIENTED_EDGE ( 'NONE', *, *, #6132, .T. ) ;
#5071=EDGE_CURVE ( 'NONE', #29654, #21604, #65432, .T. ) ;
#5073=AXIS2_PLACEMENT_3D ( 'NONE', #51772, #46483, #51435 ) ;
#5085=ORIENTED_EDGE ( 'NONE', *, *, #28263, .T. ) ;
#5091=DIRECTION ( 'NONE',  ( 5.096990367256702165E-18, 2.289061013375335776E-19, -1.000000000000000000 ) ) ;
#5093=CARTESIAN_POINT ( 'NONE',  ( 21.38432669263065833, -61.76910524360950916, 3.125053320693560257E-16 ) ) ;
#5096=EDGE_CURVE ( 'NONE', #66616, #22625, #52147, .T. ) ;
#5112=FACE_OUTER_BOUND ( 'NONE', #62244, .T. ) ;
#5114=VERTEX_POINT ( 'NONE', #40430 ) ;
#5119=FACE_OUTER_BOUND ( 'NONE', #39832, .T. ) ;
#5138=VECTOR ( 'NONE', #28617, 1000.000000000000000 ) ;
#5143=ORIENTED_EDGE ( 'NONE', *, *, #21925, .F. ) ;
#5145=ORIENTED_EDGE ( 'NONE', *, *, #67910, .F. ) ;
#5148=ADVANCED_FACE ( 'NONE', ( #51683 ), #13364, .F. ) ;
#5150=EDGE_CURVE ( 'NONE', #417, #634, #12847, .T. ) ;
#5157=EDGE_LOOP ( 'NONE', ( #14135, #29533, #1574, #37825 ) ) ;
#5162=DIRECTION ( 'NONE',  ( -0.3930250316539278255, 0.9195277725514487965, 0.000000000000000000 ) ) ;
#5163=DIRECTION ( 'NONE',  ( -0.5508969814521065267, 0.8345732537212999791, 0.000000000000000000 ) ) ;
#5166=CARTESIAN_POINT ( 'NONE',  ( 23.37466875127750754, -46.07527483894288878, 26.66469104408689361 ) ) ;
#5172=ORIENTED_EDGE ( 'NONE', *, *, #42706, .T. ) ;
#5178=DIRECTION ( 'NONE',  ( -0.000000000000000000, -0.000000000000000000, -1.000000000000000000 ) ) ;
#5182=DIRECTION ( 'NONE',  ( -0.1342332658176522420, -0.9909497617679351444, 0.000000000000000000 ) ) ;
#5184=EDGE_CURVE ( 'NONE', #22856, #4077, #33009, .T. ) ;
#5185=AXIS2_PLACEMENT_3D ( 'NONE', #67857, #26320, #19651 ) ;
#5192=CARTESIAN_POINT ( 'NONE',  ( 22.91085947427763614, -30.73415342201930756, 13.32819397642333392 ) ) ;
#5199=EDGE_LOOP ( 'NONE', ( #19131, #50473, #60429, #68962 ) ) ;
#5212=LINE ( 'NONE', #48433, #21044 ) ;
#5226=ORIENTED_EDGE ( 'NONE', *, *, #40932, .F. ) ;
#5233=DIRECTION ( 'NONE',  ( 0.000000000000000000, 0.000000000000000000, 1.000000000000000000 ) ) ;
#5238=EDGE_CURVE ( 'NONE', #13950, #30161, #35854, .T. ) ;
#5241=EDGE_CURVE ( 'NONE', #30922, #11740, #52371, .T. ) ;
#5244=DIRECTION ( 'NONE',  ( -0.000000000000000000, -0.000000000000000000, -1.000000000000000000 ) ) ;
#5250=CARTESIAN_POINT ( 'NONE',  ( 9.962235950564870990, 64.23203137738423152, 170.0000000000000000 ) ) ;
#5252=CARTESIAN_POINT ( 'NONE',  ( 24.33197399592810228, 22.91807451166457810, 6.893342938366306072 ) ) ;
#5253=ORIENTED_EDGE ( 'NONE', *, *, #58288, .F. ) ;
#5254=CARTESIAN_POINT ( 'NONE',  ( 23.63370729589335895, -52.11334794818031213, 73.58025477438755502 ) ) ;
#5274=CYLINDRICAL_SURFACE ( 'NONE', #41754, 65.00000000000000000 ) ;
#5281=ORIENTED_EDGE ( 'NONE', *, *, #24163, .T. ) ;
#5287=FACE_OUTER_BOUND ( 'NONE', #18779, .T. ) ;
#5290=CARTESIAN_POINT ( 'NONE',  ( 0.000000000000000000, 0.000000000000000000, 133.5802547743875550 ) ) ;
#5296=LINE ( 'NONE', #9892, #65809 ) ;
#5305=ORIENTED_EDGE ( 'NONE', *, *, #22711, .F. ) ;
#5317=DIRECTION ( 'NONE',  ( -0.7227948638273978821, 0.6910626489868580968, 5.102127870520021999E-18 ) ) ;
#5319=CARTESIAN_POINT ( 'NONE',  ( 55.04622673932353649, 19.32405938320713545, 27.58472315868179692 ) ) ;
#5323=VECTOR ( 'NONE', #24064, 1000.000000000000000 ) ;
#5329=CYLINDRICAL_SURFACE ( 'NONE', #1723, 65.36598343705435354 ) ;
#5337=FACE_OUTER_BOUND ( 'NONE', #17010, .T. ) ;
#5341=ORIENTED_EDGE ( 'NONE', *, *, #59299, .F. ) ;
#5342=AXIS2_PLACEMENT_3D ( 'NONE', #63389, #9578, #4304 ) ;
#5344=ORIENTED_EDGE ( 'NONE', *, *, #35996, .F. ) ;
#5347=CARTESIAN_POINT ( 'NONE',  ( 41.49663191311347532, 50.03028622612080767, 40.00000000000003553 ) ) ;
#5349=CARTESIAN_POINT ( 'NONE',  ( -31.90315521289063128, -56.64813493366051489, 170.0000000000000000 ) ) ;
#5350=CARTESIAN_POINT ( 'NONE',  ( -13.90880002535191373, -35.72171433227753568, 13.32819299319724848 ) ) ;
#5356=VERTEX_POINT ( 'NONE', #10485 ) ;
#5369=CARTESIAN_POINT ( 'NONE',  ( 26.53820682833769951, -51.95411367369387534, 27.58472315868180402 ) ) ;
#5372=DIRECTION ( 'NONE',  ( 1.000000000000000000, 0.000000000000000000, 0.000000000000000000 ) ) ;
#5376=VECTOR ( 'NONE', #24854, 1000.000000000000227 ) ;
#5378=CARTESIAN_POINT ( 'NONE',  ( 36.61292551086603453, 65.40035471292272007, 41.38025477438755928 ) ) ;
#5383=ORIENTED_EDGE ( 'NONE', *, *, #25327, .T. ) ;
#5386=ADVANCED_FACE ( 'NONE', ( #37216 ), #43179, .T. ) ;
#5389=EDGE_LOOP ( 'NONE', ( #16285, #24039, #36941, #57316 ) ) ;
#5392=EDGE_CURVE ( 'NONE', #66440, #11134, #64302, .T. ) ;
#5394=ORIENTED_EDGE ( 'NONE', *, *, #8361, .T. ) ;
#5404=CARTESIAN_POINT ( 'NONE',  ( 24.91130694661013578, 3.250319586706704733, 0.000000000000000000 ) ) ;
#5405=EDGE_CURVE ( 'NONE', #34747, #44455, #54167, .T. ) ;
#5408=CARTESIAN_POINT ( 'NONE',  ( -29.87147652227455552, 68.79592317125366208, 133.5802547743875550 ) ) ;
#5411=ORIENTED_EDGE ( 'NONE', *, *, #10375, .T. ) ;
#5415=CARTESIAN_POINT ( 'NONE',  ( 0.000000000000000000, 0.000000000000000000, 41.38025477438755928 ) ) ;
#5420=DIRECTION ( 'NONE',  ( 0.000000000000000000, 0.000000000000000000, 1.000000000000000000 ) ) ;
#5421=ORIENTED_EDGE ( 'NONE', *, *, #32183, .T. ) ;
#5424=ORIENTED_EDGE ( 'NONE', *, *, #44321, .T. ) ;
#5430=VECTOR ( 'NONE', #47117, 1000.000000000000000 ) ;
#5432=DIRECTION ( 'NONE',  ( 1.000000000000000000, 0.000000000000000000, 0.000000000000000000 ) ) ;
#5439=LINE ( 'NONE', #43057, #22524 ) ;
#5441=ORIENTED_EDGE ( 'NONE', *, *, #53962, .F. ) ;
#5442=CARTESIAN_POINT ( 'NONE',  ( -64.18058723658653264, 10.37664328995176888, 170.0000000000000000 ) ) ;
#5443=DIRECTION ( 'NONE',  ( -0.000000000000000000, -0.000000000000000000, -1.000000000000000000 ) ) ;
#5445=CARTESIAN_POINT ( 'NONE',  ( -68.11501976657811497, -31.41506934893937952, 170.0000000000000000 ) ) ;
#5450=DIRECTION ( 'NONE',  ( 1.000000000000000000, 6.217248937900876626E-15, 0.000000000000000000 ) ) ;
#5457=DIRECTION ( 'NONE',  ( -0.04486483035050447404, -0.9989930665413151445, 0.000000000000000000 ) ) ;
#5464=ADVANCED_FACE ( 'NONE', ( #53384 ), #63275, .T. ) ;
#5466=VERTEX_POINT ( 'NONE', #31603 ) ;
#5470=CARTESIAN_POINT ( 'NONE',  ( 4.165045035621077751, -64.88046627338039229, 0.000000000000000000 ) ) ;
#5473=DIRECTION ( 'NONE',  ( 1.000000000000000000, 0.000000000000000000, 0.000000000000000000 ) ) ;
#5474=EDGE_CURVE ( 'NONE', #40228, #3230, #51002, .T. ) ;
#5487=EDGE_LOOP ( 'NONE', ( #6115, #65095, #7510, #30011 ) ) ;
#5492=LINE ( 'NONE', #24635, #69443 ) ;
#5493=CARTESIAN_POINT ( 'NONE',  ( 31.22608597448339651, 41.16111765196011163, 26.66469066592269144 ) ) ;
#5503=CARTESIAN_POINT ( 'NONE',  ( -37.04655464516844177, 53.85410457537858520, 3.125053320693551875E-16 ) ) ;
#5504=AXIS2_PLACEMENT_3D ( 'NONE', #28343, #51459, #6548 ) ;
#5505=DIRECTION ( 'NONE',  ( -0.000000000000000000, -0.000000000000000000, -1.000000000000000000 ) ) ;
#5508=DIRECTION ( 'NONE',  ( -1.000000000000000000, 0.000000000000000000, 0.000000000000000000 ) ) ;
#5524=DIRECTION ( 'NONE',  ( 0.000000000000000000, 0.000000000000000000, 1.000000000000000000 ) ) ;
#5526=EDGE_CURVE ( 'NONE', #15204, #59881, #42001, .T. ) ;
#5527=ORIENTED_EDGE ( 'NONE', *, *, #40906, .T. ) ;
#5528=FACE_OUTER_BOUND ( 'NONE', #23837, .T. ) ;
#5550=EDGE_CURVE ( 'NONE', #63750, #6327, #16795, .T. ) ;
#5551=ORIENTED_EDGE ( 'NONE', *, *, #32245, .T. ) ;
#5555=DIRECTION ( 'NONE',  ( 0.000000000000000000, 0.000000000000000000, -1.000000000000000000 ) ) ;
#5557=CARTESIAN_POINT ( 'NONE',  ( 0.000000000000000000, 0.000000000000000000, 0.000000000000000000 ) ) ;
#5571=EDGE_LOOP ( 'NONE', ( #45400, #6325, #17133, #21972 ) ) ;
#5580=CARTESIAN_POINT ( 'NONE',  ( -24.07306039673040132, -53.14126562679988552, 27.58472315868179692 ) ) ;
#5582=CARTESIAN_POINT ( 'NONE',  ( 48.11816970607237209, 43.69944786994017250, 170.0000000000000000 ) ) ;
#5584=FACE_OUTER_BOUND ( 'NONE', #8189, .T. ) ;
#5586=DIRECTION ( 'NONE',  ( -0.000000000000000000, -0.000000000000000000, 1.000000000000000000 ) ) ;
#5587=ORIENTED_EDGE ( 'NONE', *, *, #8252, .T. ) ;
#5592=CARTESIAN_POINT ( 'NONE',  ( -84.49322488516129681, 0.000000000000000000, 43.58025477438756212 ) ) ;
#5598=CARTESIAN_POINT ( 'NONE',  ( -15.67984581960975632, -63.08044415722883969, 170.0000000000000000 ) ) ;
#5618=DIRECTION ( 'NONE',  ( -1.000000000000000000, 0.000000000000000000, 0.000000000000000000 ) ) ;
#5622=EDGE_CURVE ( 'NONE', #66616, #58443, #6222, .T. ) ;
#5625=EDGE_CURVE ( 'NONE', #25903, #20206, #65615, .T. ) ;
#5632=AXIS2_PLACEMENT_3D ( 'NONE', #45663, #56916, #51293 ) ;
#5639=ORIENTED_EDGE ( 'NONE', *, *, #36868, .F. ) ;
#5641=DIRECTION ( 'NONE',  ( -0.9639628606958512425, -0.2660368455666826670, 0.000000000000000000 ) ) ;
#5649=CARTESIAN_POINT ( 'NONE',  ( 23.93060502292675196, 7.646171227524815706, 0.000000000000000000 ) ) ;
#5654=B_SPLINE_CURVE_WITH_KNOTS ( 'NONE', 3,
 ( #66629, #56062, #13500, #13159, #29327, #50776 ),
 .UNSPECIFIED., .F., .F.,
 ( 4, 2, 4 ),
 ( 0.03218932648122794365, 0.06469831129177422424, 0.09720729610232048401 ),
 .UNSPECIFIED. ) ;
#5658=CARTESIAN_POINT ( 'NONE',  ( 44.74620900418437941, 37.43371647374308964, 27.58472315868181468 ) ) ;
#5659=DIRECTION ( 'NONE',  ( 0.4738686624729965824, 0.8805955318567391110, 0.000000000000000000 ) ) ;
#5670=CARTESIAN_POINT ( 'NONE',  ( 0.000000000000000000, 0.000000000000000000, 40.00000000000003553 ) ) ;
#5681=MECHANICAL_DESIGN_GEOMETRIC_PRESENTATION_REPRESENTATION('',(#61878),#13587);
#5683=FACE_OUTER_BOUND ( 'NONE', #3275, .T. ) ;
#5686=EDGE_CURVE ( 'NONE', #38444, #28906, #48354, .T. ) ;
#5701=DIRECTION ( 'NONE',  ( -0.000000000000000000, -0.000000000000000000, -1.000000000000000000 ) ) ;
#5707=ADVANCED_FACE ( 'NONE', ( #63877 ), #46518, .T. ) ;
#5711=CARTESIAN_POINT ( 'NONE',  ( -30.62628708973388569, 68.47330165179126027, 170.0000000000000000 ) ) ;
#5712=LINE ( 'NONE', #26491, #61329 ) ;
#5718=EDGE_LOOP ( 'NONE', ( #31667, #35976, #1683, #31606, #32399, #42424, #44453, #22662, #11941 ) ) ;
#5741=ORIENTED_EDGE ( 'NONE', *, *, #35158, .F. ) ;
#5742=ORIENTED_EDGE ( 'NONE', *, *, #56209, .F. ) ;
#5747=CARTESIAN_POINT ( 'NONE',  ( 46.76173513940573656, -58.63736118510165340, 0.000000000000000000 ) ) ;
#5758=DIRECTION ( 'NONE',  ( -0.000000000000000000, -0.000000000000000000, -1.000000000000000000 ) ) ;
#5762=DIRECTION ( 'NONE',  ( 0.000000000000000000, 0.000000000000000000, 1.000000000000000000 ) ) ;
#5766=ORIENTED_EDGE ( 'NONE', *, *, #50193, .F. ) ;
#5768=EDGE_LOOP ( 'NONE', ( #13742, #63676, #32036, #66265 ) ) ;
#5786=DIRECTION ( 'NONE',  ( -0.000000000000000000, 0.000000000000000000, -1.000000000000000000 ) ) ;
#5789=EDGE_CURVE ( 'NONE', #9160, #55620, #187, .T. ) ;
#5802=ORIENTED_EDGE ( 'NONE', *, *, #53599, .F. ) ;
#5813=CARTESIAN_POINT ( 'NONE',  ( -84.49322488516129681, 0.000000000000000000, 43.58025477438756212 ) ) ;
#5821=ORIENTED_EDGE ( 'NONE', *, *, #25287, .T. ) ;
#5824=ORIENTED_EDGE ( 'NONE', *, *, #31478, .T. ) ;
#5826=ADVANCED_FACE ( 'NONE', ( #47678 ), #52283, .T. ) ;
#5829=CIRCLE ( 'NONE', #63150, 74.95140232871122521 ) ;
#5868=CARTESIAN_POINT ( 'NONE',  ( 74.94097818310312675, 1.250000000000011546, 41.38025477438755928 ) ) ;
#5875=CARTESIAN_POINT ( 'NONE',  ( 7.484861546145031852, 64.56761454192836425, 170.0000000000000000 ) ) ;
#5882=CARTESIAN_POINT ( 'NONE',  ( 25.09133896793782981, -1.250000000000021982, 0.000000000000000000 ) ) ;
#5886=DIRECTION ( 'NONE',  ( 1.000000000000000000, 0.000000000000000000, 0.000000000000000000 ) ) ;
#5887=ORIENTED_EDGE ( 'NONE', *, *, #64559, .T. ) ;
#5891=CIRCLE ( 'NONE', #12648, 74.95140232871122521 ) ;
#5894=EDGE_LOOP ( 'NONE', ( #28372, #66726, #22629, #16537 ) ) ;
#5895=ORIENTED_EDGE ( 'NONE', *, *, #37393, .F. ) ;
#5901=DIRECTION ( 'NONE',  ( -0.2225209339563184452, 0.9749279121818226201, 0.000000000000000000 ) ) ;
#5903=ORIENTED_EDGE ( 'NONE', *, *, #61323, .T. ) ;
#5904=EDGE_CURVE ( 'NONE', #66023, #20436, #10747, .T. ) ;
#5911=EDGE_LOOP ( 'NONE', ( #25814, #22824, #25180, #69077 ) ) ;
#5918=LINE ( 'NONE', #16828, #32555 ) ;
#5919=PLANE ( 'NONE',  #17971 ) ;
#5923=CARTESIAN_POINT ( 'NONE',  ( 49.35747016781629526, 44.78219207638765909, 34.48241824007786249 ) ) ;
#5932=DIRECTION ( 'NONE',  ( -0.9989930665413151445, 0.04486483035050446017, 0.000000000000000000 ) ) ;
#5934=DIRECTION ( 'NONE',  ( 1.000000000000000000, 0.000000000000000000, 0.000000000000000000 ) ) ;
#5939=DIRECTION ( 'NONE',  ( -0.000000000000000000, -0.000000000000000000, -1.000000000000000000 ) ) ;
#5941=VERTEX_POINT ( 'NONE', #6522 ) ;
#5948=DIRECTION ( 'NONE',  ( 1.000000000000000000, 0.000000000000000000, 0.000000000000000000 ) ) ;
#5958=ORIENTED_EDGE ( 'NONE', *, *, #36362, .F. ) ;
#5964=DIRECTION ( 'NONE',  ( -0.000000000000000000, -0.000000000000000000, -1.000000000000000000 ) ) ;
#5965=AXIS2_PLACEMENT_3D ( 'NONE', #10715, #12124, #49383 ) ;
#5976=ORIENTED_EDGE ( 'NONE', *, *, #41471, .T. ) ;
#5984=ORIENTED_EDGE ( 'NONE', *, *, #33057, .F. ) ;
#5985=DIRECTION ( 'NONE',  ( 0.4738686624730094610, -0.8805955318567321166, 0.000000000000000000 ) ) ;
#5987=PLANE ( 'NONE',  #26082 ) ;
#5989=DIRECTION ( 'NONE',  ( 0.8584487936018728726, -0.5128992774058949156, 0.000000000000000000 ) ) ;
#5997=ORIENTED_EDGE ( 'NONE', *, *, #63943, .T. ) ;
#6004=PLANE ( 'NONE',  #15849 ) ;
#6018=LINE ( 'NONE', #11295, #50880 ) ;
#6026=VECTOR ( 'NONE', #14535, 1000.000000000000114 ) ;
#6029=ORIENTED_EDGE ( 'NONE', *, *, #21529, .T. ) ;
#6031=ORIENTED_EDGE ( 'NONE', *, *, #38207, .F. ) ;
#6049=EDGE_CURVE ( 'NONE', #20617, #62854, #67021, .T. ) ;
#6053=CARTESIAN_POINT ( 'NONE',  ( -29.70166638324878150, -57.83280658984300970, 43.58025477438756923 ) ) ;
#6055=CARTESIAN_POINT ( 'NONE',  ( 21.27121078971613244, 61.42097029141973508, 170.0000000000000000 ) ) ;
#6056=CARTESIAN_POINT ( 'NONE',  ( -24.39249304643357519, -60.24953346690487166, 40.00000000000003553 ) ) ;
#6063=VECTOR ( 'NONE', #200, 1000.000000000000000 ) ;
#6078=AXIS2_PLACEMENT_3D ( 'NONE', #18807, #40952, #41304 ) ;
#6082=AXIS2_PLACEMENT_3D ( 'NONE', #36546, #16462, #5555 ) ;
#6090=VERTEX_POINT ( 'NONE', #59791 ) ;
#6101=CARTESIAN_POINT ( 'NONE',  ( 15.68296563925494702, 63.09411298019766434, 170.0000000000000000 ) ) ;
#6107=DIRECTION ( 'NONE',  ( -0.5508969814521065267, 0.8345732537212999791, 0.000000000000000000 ) ) ;
#6115=ORIENTED_EDGE ( 'NONE', *, *, #51628, .T. ) ;
#6126=LINE ( 'NONE', #59938, #12679 ) ;
#6131=DIRECTION ( 'NONE',  ( -1.000000000000000000, 0.000000000000000000, 0.000000000000000000 ) ) ;
#6132=EDGE_CURVE ( 'NONE', #29614, #23495, #3741, .T. ) ;
#6137=ORIENTED_EDGE ( 'NONE', *, *, #4375, .T. ) ;
#6144=ORIENTED_EDGE ( 'NONE', *, *, #18397, .F. ) ;
#6145=EDGE_LOOP ( 'NONE', ( #2439, #4920, #47219, #8611 ) ) ;
#6147=CARTESIAN_POINT ( 'NONE',  ( 0.000000000000000000, 0.000000000000000000, 170.0000000000000000 ) ) ;
#6149=ORIENTED_EDGE ( 'NONE', *, *, #34558, .F. ) ;
#6158=CARTESIAN_POINT ( 'NONE',  ( 23.05216796272336666, 9.986758404124199018, 3.061616997868437868E-16 ) ) ;
#6174=EDGE_CURVE ( 'NONE', #10843, #21469, #37057, .T. ) ;
#6182=VECTOR ( 'NONE', #34667, 1000.000000000000000 ) ;
#6190=ORIENTED_EDGE ( 'NONE', *, *, #19312, .T. ) ;
#6191=ADVANCED_FACE ( 'NONE', ( #11607 ), #56673, .T. ) ;
#6192=ORIENTED_EDGE ( 'NONE', *, *, #9056, .T. ) ;
#6193=ADVANCED_FACE ( 'NONE', ( #36026 ), #4019, .T. ) ;
#6195=DIRECTION ( 'NONE',  ( -0.000000000000000000, 0.000000000000000000, -1.000000000000000000 ) ) ;
#6197=PLANE ( 'NONE',  #24495 ) ;
#6199=LINE ( 'NONE', #22379, #31098 ) ;
#6204=VERTEX_POINT ( 'NONE', #20190 ) ;
#6222=B_SPLINE_CURVE_WITH_KNOTS ( 'NONE', 3,
 ( #13959, #51601, #62848, #56886, #3409, #24868 ),
 .UNSPECIFIED., .F., .F.,
 ( 4, 2, 4 ),
 ( 0.03218953612796865427, 0.06469846386257042947, 0.09720739159717220468 ),
 .UNSPECIFIED. ) ;
#6224=VECTOR ( 'NONE', #52718, 1000.000000000000227 ) ;
#6233=VECTOR ( 'NONE', #49492, 1000.000000000000114 ) ;
#6234=CARTESIAN_POINT ( 'NONE',  ( 8.828807734115068584, -74.48902371486708773, 170.0000000000000000 ) ) ;
#6236=CARTESIAN_POINT ( 'NONE',  ( -49.77357484059193382, 41.82599373102802076, 0.000000000000000000 ) ) ;
#6239=VECTOR ( 'NONE', #30416, 1000.000000000000000 ) ;
#6242=CARTESIAN_POINT ( 'NONE',  ( -16.20761945673107363, 34.73915175314249382, 13.32819299319723605 ) ) ;
#6251=EDGE_CURVE ( 'NONE', #24023, #32779, #3903, .T. ) ;
#6259=EDGE_CURVE ( 'NONE', #22131, #59849, #36371, .T. ) ;
#6262=ORIENTED_EDGE ( 'NONE', *, *, #363, .F. ) ;
#6263=DIRECTION ( 'NONE',  ( -1.000000000000000000, 0.000000000000000000, 0.000000000000000000 ) ) ;
#6264=AXIS2_PLACEMENT_3D ( 'NONE', #45732, #66859, #18998 ) ;
#6272=VECTOR ( 'NONE', #35114, 1000.000000000000000 ) ;
#6273=VERTEX_POINT ( 'NONE', #68715 ) ;
#6274=CARTESIAN_POINT ( 'NONE',  ( -27.33809837083532557, -60.78020170929433874, 34.48241795236666007 ) ) ;
#6276=AXIS2_PLACEMENT_3D ( 'NONE', #34371, #7282, #28735 ) ;
#6285=VECTOR ( 'NONE', #38101, 1000.000000000000000 ) ;
#6287=ORIENTED_EDGE ( 'NONE', *, *, #13678, .F. ) ;
#6300=VERTEX_POINT ( 'NONE', #69051 ) ;
#6303=ORIENTED_EDGE ( 'NONE', *, *, #5241, .T. ) ;
#6305=CARTESIAN_POINT ( 'NONE',  ( -1.068536297472280960, -51.65427651052054614, 26.66469066592268433 ) ) ;
#6309=CARTESIAN_POINT ( 'NONE',  ( 0.000000000000000000, 0.000000000000000000, 170.0000000000000000 ) ) ;
#6317=CARTESIAN_POINT ( 'NONE',  ( 0.000000000000000000, 0.000000000000000000, 170.0000000000000000 ) ) ;
#6325=ORIENTED_EDGE ( 'NONE', *, *, #65862, .F. ) ;
#6327=VERTEX_POINT ( 'NONE', #29198 ) ;
#6330=PLANE ( 'NONE',  #40632 ) ;
#6331=CIRCLE ( 'NONE', #36672, 65.00000000000000000 ) ;
#6332=CARTESIAN_POINT ( 'NONE',  ( -71.96466849523078224, 21.15771699336999845, 170.0000000000000000 ) ) ;
#6335=AXIS2_PLACEMENT_3D ( 'NONE', #10289, #16265, #4347 ) ;
#6338=EDGE_CURVE ( 'NONE', #16525, #37239, #59168, .T. ) ;
#6344=AXIS2_PLACEMENT_3D ( 'NONE', #44362, #23279, #17644 ) ;
#6345=CARTESIAN_POINT ( 'NONE',  ( 19.25636590080467769, -33.14646233425818878, 13.32819299319722894 ) ) ;
#6346=ORIENTED_EDGE ( 'NONE', *, *, #46476, .T. ) ;
#6352=CARTESIAN_POINT ( 'NONE',  ( 61.62594073580542897, 21.79346734965000820, 6.377659838150158269E-18 ) ) ;
#6357=LINE ( 'NONE', #32055, #17698 ) ;
#6358=CARTESIAN_POINT ( 'NONE',  ( -84.49322488516129681, 0.000000000000000000, 43.58025477438756212 ) ) ;
#6363=ORIENTED_EDGE ( 'NONE', *, *, #5405, .T. ) ;
#6364=EDGE_CURVE ( 'NONE', #37468, #45637, #17234, .T. ) ;
#6365=EDGE_CURVE ( 'NONE', #64051, #48012, #7400, .T. ) ;
#6402=CARTESIAN_POINT ( 'NONE',  ( -59.09450113343203270, -27.07101652673575032, 170.0000000000000000 ) ) ;
#6407=CARTESIAN_POINT ( 'NONE',  ( 45.82394788922869822, -46.11928342727429708, 43.58025477438756923 ) ) ;
#6422=ORIENTED_EDGE ( 'NONE', *, *, #18455, .T. ) ;
#6423=FACE_OUTER_BOUND ( 'NONE', #23439, .T. ) ;
#6424=EDGE_CURVE ( 'NONE', #26839, #37838, #31963, .T. ) ;
#6430=EDGE_CURVE ( 'NONE', #7966, #38444, #21856, .T. ) ;
#6434=EDGE_LOOP ( 'NONE', ( #43960, #21401, #58839, #66124, #25080, #24775, #21189, #501, #27098 ) ) ;
#6439=CARTESIAN_POINT ( 'NONE',  ( -18.89790202299119315, -62.20684691518632548, 170.0000000000000000 ) ) ;
#6444=AXIS2_PLACEMENT_3D ( 'NONE', #32738, #60159, #39408 ) ;
#6452=ORIENTED_EDGE ( 'NONE', *, *, #43333, .T. ) ;
#6453=VERTEX_POINT ( 'NONE', #25317 ) ;
#6456=ORIENTED_EDGE ( 'NONE', *, *, #54218, .F. ) ;
#6465=CARTESIAN_POINT ( 'NONE',  ( 4.360227613243417011, 41.50064055034692956, 13.79046412288134249 ) ) ;
#6474=AXIS2_PLACEMENT_3D ( 'NONE', #7658, #66411, #6945 ) ;
#6479=ORIENTED_EDGE ( 'NONE', *, *, #26766, .F. ) ;
#6481=AXIS2_PLACEMENT_3D ( 'NONE', #44370, #17652, #1829 ) ;
#6482=CARTESIAN_POINT ( 'NONE',  ( -62.66631205405185057, 18.59153367093362874, 6.377659838150142862E-18 ) ) ;
#6498=DIRECTION ( 'NONE',  ( -0.5508969814521065267, 0.8345732537212999791, 0.000000000000000000 ) ) ;
#6512=CARTESIAN_POINT ( 'NONE',  ( -15.47041015649658391, 73.39774458108210808, 170.0000000000000000 ) ) ;
#6513=VERTEX_POINT ( 'NONE', #63630 ) ;
#6517=CARTESIAN_POINT ( 'NONE',  ( 0.000000000000000000, 0.000000000000000000, 170.0000000000000000 ) ) ;
#6522=CARTESIAN_POINT ( 'NONE',  ( 60.40479419793764038, 24.00543350795394915, 40.00000000000003553 ) ) ;
#6528=CIRCLE ( 'NONE', #28993, 24.99999999999985434 ) ;
#6530=CARTESIAN_POINT ( 'NONE',  ( 30.12852347772543737, -74.98256102853682137, 133.5802547743875550 ) ) ;
#6532=CIRCLE ( 'NONE', #45855, 65.00000000000000000 ) ;
#6537=AXIS2_PLACEMENT_3D ( 'NONE', #33889, #28246, #60266 ) ;
#6545=CIRCLE ( 'NONE', #22259, 65.00000000000000000 ) ;
#6546=CARTESIAN_POINT ( 'NONE',  ( 2.112947028649122760, -24.91054906769651112, 0.000000000000000000 ) ) ;
#6548=DIRECTION ( 'NONE',  ( -1.000000000000000000, 0.000000000000000000, 0.000000000000000000 ) ) ;
#6551=EDGE_LOOP ( 'NONE', ( #58643, #8070, #32987, #39910 ) ) ;
#6552=DIRECTION ( 'NONE',  ( -0.3930250316539278810, 0.9195277725514489076, 0.000000000000000000 ) ) ;
#6555=CARTESIAN_POINT ( 'NONE',  ( -25.03927893945753169, 61.76276428842881216, 34.48241795236666718 ) ) ;
#6557=CARTESIAN_POINT ( 'NONE',  ( 34.76618902119740540, 54.93755186520760958, 0.000000000000000000 ) ) ;
#6564=FACE_OUTER_BOUND ( 'NONE', #55655, .T. ) ;
#6570=FACE_OUTER_BOUND ( 'NONE', #48929, .T. ) ;
#6571=DIRECTION ( 'NONE',  ( -1.000000000000000000, 0.000000000000000000, 0.000000000000000000 ) ) ;
#6577=CARTESIAN_POINT ( 'NONE',  ( 14.59045944429442443, -20.30070179093305427, 0.000000000000000000 ) ) ;
#6580=EDGE_CURVE ( 'NONE', #8790, #22641, #69045, .T. ) ;
#6585=AXIS2_PLACEMENT_3D ( 'NONE', #17131, #49136, #38250 ) ;
#6586=ORIENTED_EDGE ( 'NONE', *, *, #29227, .T. ) ;
#6588=CARTESIAN_POINT ( 'NONE',  ( 63.69186821587179281, -39.51023455020688857, 41.38025477438755928 ) ) ;
#6594=DIRECTION ( 'NONE',  ( -0.6910626489868685329, 0.7227948638273878901, 0.000000000000000000 ) ) ;
#6607=ORIENTED_EDGE ( 'NONE', *, *, #8676, .F. ) ;
#6614=EDGE_LOOP ( 'NONE', ( #86, #12869, #17143, #25315 ) ) ;
#6615=CARTESIAN_POINT ( 'NONE',  ( 0.000000000000000000, 0.000000000000000000, 0.000000000000000000 ) ) ;
#6616=CARTESIAN_POINT ( 'NONE',  ( 69.77839676787897361, -27.52340539439948586, 170.0000000000000000 ) ) ;
#6618=ORIENTED_EDGE ( 'NONE', *, *, #67910, .T. ) ;
#6619=CARTESIAN_POINT ( 'NONE',  ( 0.000000000000000000, 0.000000000000000000, 170.0000000000000000 ) ) ;
#6625=AXIS2_PLACEMENT_3D ( 'NONE', #17410, #38887, #56101 ) ;
#6637=CARTESIAN_POINT ( 'NONE',  ( 31.89651141207616192, -56.63578868294582946, 170.0000000000000000 ) ) ;
#6645=LINE ( 'NONE', #17549, #47949 ) ;
#6647=CARTESIAN_POINT ( 'NONE',  ( -4.613603609465520172, 74.86839895266042788, 170.0000000000000000 ) ) ;
#6651=DIRECTION ( 'NONE',  ( -1.000000000000000000, 0.000000000000000000, 0.000000000000000000 ) ) ;
#6654=CARTESIAN_POINT ( 'NONE',  ( 0.000000000000000000, 0.000000000000000000, 40.00000000000003553 ) ) ;
#6656=EDGE_LOOP ( 'NONE', ( #30988, #55051, #251, #3624 ) ) ;
#6664=EDGE_CURVE ( 'NONE', #6513, #7998, #51913, .T. ) ;
#6668=ORIENTED_EDGE ( 'NONE', *, *, #20192, .T. ) ;
#6675=VERTEX_POINT ( 'NONE', #14289 ) ;
#6680=ORIENTED_EDGE ( 'NONE', *, *, #55858, .T. ) ;
#6682=DIRECTION ( 'NONE',  ( -1.000000000000000000, 0.000000000000000000, 0.000000000000000000 ) ) ;
#6686=DIRECTION ( 'NONE',  ( 0.6234898018587431423, -0.7818314824680220321, 0.000000000000000000 ) ) ;
#6693=DIRECTION ( 'NONE',  ( 1.000000000000000000, 0.000000000000000000, 0.000000000000000000 ) ) ;
#6694=ORIENTED_EDGE ( 'NONE', *, *, #28577, .T. ) ;
#6699=ORIENTED_EDGE ( 'NONE', *, *, #35581, .T. ) ;
#6708=VERTEX_POINT ( 'NONE', #9348 ) ;
#6714=CARTESIAN_POINT ( 'NONE',  ( 0.000000000000000000, 0.000000000000000000, 43.58025477438756212 ) ) ;
#6719=CARTESIAN_POINT ( 'NONE',  ( 24.36509522348982060, 70.94296747916789059, 43.58025477438756212 ) ) ;
#6725=ORIENTED_EDGE ( 'NONE', *, *, #53176, .F. ) ;
#6727=ORIENTED_EDGE ( 'NONE', *, *, #2556, .F. ) ;
#6728=DIRECTION ( 'NONE',  ( 0.000000000000000000, 0.000000000000000000, 1.000000000000000000 ) ) ;
#6731=DIRECTION ( 'NONE',  ( -0.000000000000000000, -0.000000000000000000, -1.000000000000000000 ) ) ;
#6737=CARTESIAN_POINT ( 'NONE',  ( -4.610955605663495938, 74.80943656680578613, 41.38025477438755928 ) ) ;
#6743=PLANE ( 'NONE',  #28937 ) ;
#6745=EDGE_CURVE ( 'NONE', #61117, #57624, #65271, .T. ) ;
#6758=ORIENTED_EDGE ( 'NONE', *, *, #52575, .T. ) ;
#6760=DIRECTION ( 'NONE',  ( 1.000000000000000000, 0.000000000000000000, 0.000000000000000000 ) ) ;
#6768=ORIENTED_EDGE ( 'NONE', *, *, #56706, .F. ) ;
#6770=CARTESIAN_POINT ( 'NONE',  ( 0.000000000000000000, 0.000000000000000000, 170.0000000000000000 ) ) ;
#6771=ORIENTED_EDGE ( 'NONE', *, *, #43046, .T. ) ;
#6772=ORIENTED_EDGE ( 'NONE', *, *, #9851, .T. ) ;
#6776=EDGE_LOOP ( 'NONE', ( #2142, #56466, #43071, #32842 ) ) ;
#6778=CARTESIAN_POINT ( 'NONE',  ( 0.000000000000000000, 0.000000000000000000, 41.38025477438755928 ) ) ;
#6786=CYLINDRICAL_SURFACE ( 'NONE', #59485, 65.00000000000000000 ) ;
#6787=DIRECTION ( 'NONE',  ( -0.000000000000000000, -0.000000000000000000, -1.000000000000000000 ) ) ;
#6789=CYLINDRICAL_SURFACE ( 'NONE', #9624, 65.36598343705435354 ) ;
#6790=DIRECTION ( 'NONE',  ( -1.000000000000000000, 0.000000000000000000, 0.000000000000000000 ) ) ;
#6793=VECTOR ( 'NONE', #65656, 1000.000000000000227 ) ;
#6801=CARTESIAN_POINT ( 'NONE',  ( -34.47910341156048020, 23.50544998411836772, 13.79046412380261621 ) ) ;
#6806=PLANE ( 'NONE',  #63259 ) ;
#6810=LINE ( 'NONE', #39523, #32095 ) ;
#6815=LINE ( 'NONE', #28265, #39439 ) ;
#6827=ADVANCED_FACE ( 'NONE', ( #60689 ), #54706, .T. ) ;
#6829=LINE ( 'NONE', #44467, #23697 ) ;
#6831=ORIENTED_EDGE ( 'NONE', *, *, #1246, .T. ) ;
#6839=FACE_OUTER_BOUND ( 'NONE', #47891, .T. ) ;
#6846=ADVANCED_FACE ( 'NONE', ( #23062 ), #39246, .T. ) ;
#6847=DIRECTION ( 'NONE',  ( -0.000000000000000000, -0.000000000000000000, -1.000000000000000000 ) ) ;
#6868=CARTESIAN_POINT ( 'NONE',  ( 54.16779028252168615, 21.66464678626688567, 27.58472369380032774 ) ) ;
#6874=CARTESIAN_POINT ( 'NONE',  ( 32.06997139192709056, 56.95813133885486934, 6.377659838150122832E-18 ) ) ;
#6880=CARTESIAN_POINT ( 'NONE',  ( 22.91085886047801168, 30.73415265233982296, 13.32819299319723605 ) ) ;
#6881=LINE ( 'NONE', #39596, #14118 ) ;
#6884=DIRECTION ( 'NONE',  ( -0.000000000000000000, -0.000000000000000000, -1.000000000000000000 ) ) ;
#6894=DIRECTION ( 'NONE',  ( 0.000000000000000000, 0.000000000000000000, -1.000000000000000000 ) ) ;
#6902=EDGE_CURVE ( 'NONE', #50073, #34263, #55055, .T. ) ;
#6904=ORIENTED_EDGE ( 'NONE', *, *, #54962, .F. ) ;
#6905=CARTESIAN_POINT ( 'NONE',  ( 0.000000000000000000, 0.000000000000000000, 170.0000000000000000 ) ) ;
#6907=VECTOR ( 'NONE', #42934, 1000.000000000000114 ) ;
#6910=CARTESIAN_POINT ( 'NONE',  ( 7.484861546145031852, 64.56761454192836425, 73.58025477438756923 ) ) ;
#6917=AXIS2_PLACEMENT_3D ( 'NONE', #37014, #46877, #9940 ) ;
#6920=CARTESIAN_POINT ( 'NONE',  ( 32.23328838621442571, -26.50150695468921214, 13.79046412417416789 ) ) ;
#6921=CARTESIAN_POINT ( 'NONE',  ( 0.000000000000000000, 0.000000000000000000, 41.38025477438755928 ) ) ;
#6927=CARTESIAN_POINT ( 'NONE',  ( -65.36598343705435354, 0.000000000000000000, 41.38025477438755928 ) ) ;
#6928=DIRECTION ( 'NONE',  ( -0.8090169943749506709, 0.5877852522924686962, 0.000000000000000000 ) ) ;
#6932=CARTESIAN_POINT ( 'NONE',  ( 20.89850557012451659, -13.94239061780404043, 0.000000000000000000 ) ) ;
#6938=DIRECTION ( 'NONE',  ( -0.000000000000000000, -0.000000000000000000, -1.000000000000000000 ) ) ;
#6945=DIRECTION ( 'NONE',  ( -1.000000000000000000, 0.000000000000000000, 0.000000000000000000 ) ) ;
#6965=CARTESIAN_POINT ( 'NONE',  ( -74.81012118577224612, 5.477980300262961677, 170.0000000000000000 ) ) ;
#6967=VERTEX_POINT ( 'NONE', #51533 ) ;
#6968=FACE_OUTER_BOUND ( 'NONE', #36495, .T. ) ;
#6969=EDGE_CURVE ( 'NONE', #24447, #26335, #36538, .T. ) ;
#6977=VERTEX_POINT ( 'NONE', #62430 ) ;
#6987=ORIENTED_EDGE ( 'NONE', *, *, #48024, .F. ) ;
#6989=ORIENTED_EDGE ( 'NONE', *, *, #4518, .F. ) ;
#6992=VERTEX_POINT ( 'NONE', #36041 ) ;
#7002=EDGE_LOOP ( 'NONE', ( #5421, #66848, #37262, #64584 ) ) ;
#7003=VECTOR ( 'NONE', #56273, 1000.000000000000000 ) ;
#7005=CARTESIAN_POINT ( 'NONE',  ( 0.000000000000000000, 0.000000000000000000, 0.000000000000000000 ) ) ;
#7007=LINE ( 'NONE', #23545, #56715 ) ;
#7014=VECTOR ( 'NONE', #55877, 999.9999999999998863 ) ;
#7030=DIRECTION ( 'NONE',  ( 1.000000000000000000, 0.000000000000000000, -0.000000000000000000 ) ) ;
#7044=DIRECTION ( 'NONE',  ( -0.9639628606958513535, -0.2660368455666826670, 0.000000000000000000 ) ) ;
#7048=EDGE_CURVE ( 'NONE', #60623, #47253, #47609, .T. ) ;
#7049=VECTOR ( 'NONE', #39546, 1000.000000000000000 ) ;
#7052=LINE ( 'NONE', #7418, #38717 ) ;
#7054=DIRECTION ( 'NONE',  ( 0.000000000000000000, 1.000000000000000000, 0.000000000000000000 ) ) ;
#7062=ADVANCED_FACE ( 'NONE', ( #27195 ), #25304, .T. ) ;
#7068=CARTESIAN_POINT ( 'NONE',  ( 49.76301652092167416, 41.81676920493115546, 40.00000000000003553 ) ) ;
#7078=DIRECTION ( 'NONE',  ( 0.2660368455666687892, 0.9639628606958550172, 5.102127870520021999E-18 ) ) ;
#7083=DIRECTION ( 'NONE',  ( -1.000000000000000000, 0.000000000000000000, 0.000000000000000000 ) ) ;
#7087=CARTESIAN_POINT ( 'NONE',  ( -3.865535754268288660, 58.21137395544315751, 27.58472369367945376 ) ) ;
#7092=CARTESIAN_POINT ( 'NONE',  ( -84.49322488516129681, 0.000000000000000000, 43.58025477438756212 ) ) ;
#7098=ORIENTED_EDGE ( 'NONE', *, *, #44235, .F. ) ;
#7110=VERTEX_POINT ( 'NONE', #53228 ) ;
#7115=CARTESIAN_POINT ( 'NONE',  ( 0.000000000000000000, 0.000000000000000000, 0.000000000000000000 ) ) ;
#7119=DIRECTION ( 'NONE',  ( -0.000000000000000000, -0.000000000000000000, -1.000000000000000000 ) ) ;
#7120=LINE ( 'NONE', #38431, #45059 ) ;
#7137=DIRECTION ( 'NONE',  ( 0.8805955318567391110, -0.4738686624729965824, 0.000000000000000000 ) ) ;
#7140=DIRECTION ( 'NONE',  ( -1.000000000000000000, 0.000000000000000000, 0.000000000000000000 ) ) ;
#7144=ORIENTED_EDGE ( 'NONE', *, *, #58200, .F. ) ;
#7146=AXIS2_PLACEMENT_3D ( 'NONE', #23872, #2077, #66801 ) ;
#7161=VECTOR ( 'NONE', #65081, 999.9999999999998863 ) ;
#7163=ORIENTED_EDGE ( 'NONE', *, *, #8617, .F. ) ;
#7168=LINE ( 'NONE', #1906, #66495 ) ;
#7186=CARTESIAN_POINT ( 'NONE',  ( 65.35403040894466642, 1.250000000000011546, 41.38025477438755928 ) ) ;
#7195=B_SPLINE_CURVE_WITH_KNOTS ( 'NONE', 3,
 ( #35590, #8158, #45441, #24351 ),
 .UNSPECIFIED., .F., .F.,
 ( 4, 4 ),
 ( 9.900409499100981944E-07, 0.05658314289920116785 ),
 .UNSPECIFIED. ) ;
#7197=VECTOR ( 'NONE', #47640, 1000.000000000000114 ) ;
#7201=DIRECTION ( 'NONE',  ( -9.110201094255651812E-19, -5.020134576618378958E-18, -1.000000000000000000 ) ) ;
#7205=ORIENTED_EDGE ( 'NONE', *, *, #29454, .F. ) ;
#7208=VECTOR ( 'NONE', #61197, 1000.000000000000000 ) ;
#7211=EDGE_CURVE ( 'NONE', #22641, #28657, #50745, .T. ) ;
#7212=ORIENTED_EDGE ( 'NONE', *, *, #15410, .T. ) ;
#7226=ADVANCED_FACE ( 'NONE', ( #44782 ), #6789, .T. ) ;
#7231=CARTESIAN_POINT ( 'NONE',  ( -29.70166638324878150, -57.83280658984300970, 170.0000000000000000 ) ) ;
#7240=LINE ( 'NONE', #28699, #52325 ) ;
#7243=CARTESIAN_POINT ( 'NONE',  ( 65.02478361689782105, -37.39438481343979959, 170.0000000000000000 ) ) ;
#7248=VERTEX_POINT ( 'NONE', #31031 ) ;
#7255=EDGE_CURVE ( 'NONE', #30161, #33967, #41236, .T. ) ;
#7261=AXIS2_PLACEMENT_3D ( 'NONE', #41099, #35475, #30205 ) ;
#7265=VECTOR ( 'NONE', #12636, 1000.000000000000114 ) ;
#7267=CARTESIAN_POINT ( 'NONE',  ( -84.49322488516129681, 0.000000000000000000, 43.58025477438756212 ) ) ;
#7277=CARTESIAN_POINT ( 'NONE',  ( 56.42997683260104225, 32.25922681454269991, 40.00000000000003553 ) ) ;
#7280=CARTESIAN_POINT ( 'NONE',  ( 74.94097818310312675, 1.250000000000011546, 41.38025477438755928 ) ) ;
#7282=DIRECTION ( 'NONE',  ( -0.000000000000000000, -0.000000000000000000, -1.000000000000000000 ) ) ;
#7283=CARTESIAN_POINT ( 'NONE',  ( -53.60725281709914469, 37.40286400928249577, 3.125053320693569132E-16 ) ) ;
#7287=DIRECTION ( 'NONE',  ( -0.000000000000000000, -0.000000000000000000, -1.000000000000000000 ) ) ;
#7290=CARTESIAN_POINT ( 'NONE',  ( -28.32746765835430836, -69.45586423092646555, 170.0000000000000000 ) ) ;
#7297=CARTESIAN_POINT ( 'NONE',  ( -10.96274578891778084, 22.46815979931508167, 0.000000000000000000 ) ) ;
#7298=ORIENTED_EDGE ( 'NONE', *, *, #52571, .F. ) ;
#7304=CONICAL_SURFACE ( 'NONE', #54470, 65.00000000000000000, 0.7853981633974497223 ) ;
#7313=ORIENTED_EDGE ( 'NONE', *, *, #28692, .F. ) ;
#7314=ADVANCED_FACE ( 'NONE', ( #10934 ), #42153, .T. ) ;
#7315=ORIENTED_EDGE ( 'NONE', *, *, #54651, .F. ) ;
#7318=CARTESIAN_POINT ( 'NONE',  ( 21.98745393275192583, 71.71550996510526943, 133.5802547743875550 ) ) ;
#7320=PLANE ( 'NONE',  #25348 ) ;
#7321=VERTEX_POINT ( 'NONE', #49602 ) ;
#7348=VECTOR ( 'NONE', #12333, 999.9999999999998863 ) ;
#7351=VERTEX_POINT ( 'NONE', #61223 ) ;
#7353=LINE ( 'NONE', #62192, #7457 ) ;
#7367=CARTESIAN_POINT ( 'NONE',  ( -29.47687737404459085, 68.96458294135867106, 43.58025477438756212 ) ) ;
#7370=B_SPLINE_CURVE_WITH_KNOTS ( 'NONE', 3,
 ( #25011, #52423, #64010, #4245, #52749, #41871 ),
 .UNSPECIFIED., .F., .F.,
 ( 4, 2, 4 ),
 ( 0.03218935267740795358, 0.06469833035354465023, 0.09720730802968134687 ),
 .UNSPECIFIED. ) ;
#7380=DIRECTION ( 'NONE',  ( -1.000000000000000000, 0.000000000000000000, 0.000000000000000000 ) ) ;
#7383=LINE ( 'NONE', #44998, #11093 ) ;
#7391=PLANE ( 'NONE',  #13086 ) ;
#7392=LINE ( 'NONE', #60144, #13886 ) ;
#7394=EDGE_CURVE ( 'NONE', #51881, #42885, #28154, .T. ) ;
#7400=LINE ( 'NONE', #17950, #12898 ) ;
#7411=B_SPLINE_CURVE_WITH_KNOTS ( 'NONE', 3,
 ( #22498, #33760, #44992, #55195 ),
 .UNSPECIFIED., .F., .F.,
 ( 4, 4 ),
 ( 0.1259919275528359750, 0.1829744153748750768 ),
 .UNSPECIFIED. ) ;
#7418=CARTESIAN_POINT ( 'NONE',  ( 30.12852347772543027, 58.62603998952764783, 73.58025477438759765 ) ) ;
#7424=CARTESIAN_POINT ( 'NONE',  ( 0.000000000000000000, 0.000000000000000000, 40.00000000000003553 ) ) ;
#7427=CARTESIAN_POINT ( 'NONE',  ( 8.904582680624310242, -23.36040254969760355, 0.000000000000000000 ) ) ;
#7446=LINE ( 'NONE', #55976, #54640 ) ;
#7454=AXIS2_PLACEMENT_3D ( 'NONE', #27203, #32837, #54268 ) ;
#7457=VECTOR ( 'NONE', #29149, 1000.000000000000227 ) ;
#7461=VECTOR ( 'NONE', #32886, 1000.000000000000114 ) ;
#7462=VECTOR ( 'NONE', #26412, 1000.000000000000000 ) ;
#7472=EDGE_CURVE ( 'NONE', #28358, #37085, #8102, .T. ) ;
#7475=VERTEX_POINT ( 'NONE', #46418 ) ;
#7485=VERTEX_POINT ( 'NONE', #7766 ) ;
#7486=CARTESIAN_POINT ( 'NONE',  ( -56.55682276332724712, 14.31196085009922569, 27.58472369374502264 ) ) ;
#7488=DIRECTION ( 'NONE',  ( -0.000000000000000000, -0.000000000000000000, -1.000000000000000000 ) ) ;
#7494=EDGE_LOOP ( 'NONE', ( #35220, #61141, #17764, #20602 ) ) ;
#7495=DIRECTION ( 'NONE',  ( 0.6234898018587318180, 0.7818314824680311359, 0.000000000000000000 ) ) ;
#7499=CARTESIAN_POINT ( 'NONE',  ( -41.31727360890798906, 62.59299402909750398, 43.58025477438756212 ) ) ;
#7503=VECTOR ( 'NONE', #581, 1000.000000000000000 ) ;
#7510=ORIENTED_EDGE ( 'NONE', *, *, #52002, .F. ) ;
#7512=VECTOR ( 'NONE', #9429, 1000.000000000000000 ) ;
#7523=DIRECTION ( 'NONE',  ( 0.000000000000000000, 0.000000000000000000, 1.000000000000000000 ) ) ;
#7528=ORIENTED_EDGE ( 'NONE', *, *, #64229, .F. ) ;
#7538=LINE ( 'NONE', #25100, #28234 ) ;
#7540=CARTESIAN_POINT ( 'NONE',  ( -17.54261641588776754, 37.86253240666081865, 13.79046412320003689 ) ) ;
#7558=DIRECTION ( 'NONE',  ( 0.000000000000000000, 0.000000000000000000, 1.000000000000000000 ) ) ;
#7560=CIRCLE ( 'NONE', #60310, 65.00000000000000000 ) ;
#7565=DIRECTION ( 'NONE',  ( -0.3930250316539278255, 0.9195277725514487965, 0.000000000000000000 ) ) ;
#7594=ORIENTED_EDGE ( 'NONE', *, *, #39222, .T. ) ;
#7601=CIRCLE ( 'NONE', #40176, 65.36598343705435354 ) ;
#7609=DIRECTION ( 'NONE',  ( 2.998955517602045729E-18, 4.127708154724775106E-18, -1.000000000000000000 ) ) ;
#7614=CARTESIAN_POINT ( 'NONE',  ( 34.41143668122415988, 66.58502636910522199, 41.38025477438755928 ) ) ;
#7632=ORIENTED_EDGE ( 'NONE', *, *, #13053, .T. ) ;
#7640=ADVANCED_FACE ( 'NONE', ( #46950 ), #37664, .T. ) ;
#7653=CIRCLE ( 'NONE', #58191, 65.36598343705435354 ) ;
#7658=CARTESIAN_POINT ( 'NONE',  ( 0.000000000000000000, 0.000000000000000000, 41.38025477438755928 ) ) ;
#7659=DIRECTION ( 'NONE',  ( 0.3090169943749582759, -0.9510565162951499785, 0.000000000000000000 ) ) ;
#7669=AXIS2_PLACEMENT_3D ( 'NONE', #35372, #13230, #12525 ) ;
#7682=DIRECTION ( 'NONE',  ( -0.000000000000000000, -0.000000000000000000, -1.000000000000000000 ) ) ;
#7686=LINE ( 'NONE', #55872, #9265 ) ;
#7687=DIRECTION ( 'NONE',  ( 0.9839295885986295565, 0.1785568947986370392, 0.000000000000000000 ) ) ;
#7689=ADVANCED_FACE ( 'NONE', ( #9317 ), #25512, .F. ) ;
#7703=CIRCLE ( 'NONE', #64983, 65.00000000000000000 ) ;
#7711=ORIENTED_EDGE ( 'NONE', *, *, #44198, .F. ) ;
#7712=DIRECTION ( 'NONE',  ( 0.9195277725514487965, 0.3930250316539278255, 0.000000000000000000 ) ) ;
#7715=ORIENTED_EDGE ( 'NONE', *, *, #26960, .F. ) ;
#7731=DIRECTION ( 'NONE',  ( 0.2660368455666687892, 0.9639628606958550172, 0.000000000000000000 ) ) ;
#7732=B_SPLINE_CURVE_WITH_KNOTS ( 'NONE', 3,
 ( #37324, #25418, #4628, #31034 ),
 .UNSPECIFIED., .F., .F.,
 ( 4, 4 ),
 ( 0.1259919275528360860, 0.1829744153748753543 ),
 .UNSPECIFIED. ) ;
#7733=DIRECTION ( 'NONE',  ( 0.9749279121818226201, 0.2225209339563184452, 0.000000000000000000 ) ) ;
#7739=CARTESIAN_POINT ( 'NONE',  ( 73.79471914489722906, 13.39176710989777952, 43.58025477438756212 ) ) ;
#7743=ADVANCED_FACE ( 'NONE', ( #48296 ), #26532, .T. ) ;
#7747=ORIENTED_EDGE ( 'NONE', *, *, #10645, .T. ) ;
#7750=CIRCLE ( 'NONE', #69485, 65.00000000000000000 ) ;
#7756=CARTESIAN_POINT ( 'NONE',  ( 26.69682282325710787, 59.27986298182224800, 43.58025477438756923 ) ) ;
#7759=CARTESIAN_POINT ( 'NONE',  ( 0.000000000000000000, 0.000000000000000000, 40.00000000000003553 ) ) ;
#7766=CARTESIAN_POINT ( 'NONE',  ( -64.97888516016270444, -7.103257987406320417, 41.38025477438755928 ) ) ;
#7770=CARTESIAN_POINT ( 'NONE',  ( 13.02837879071828198, -36.05214194840069553, 13.32819299319723072 ) ) ;
#7787=VECTOR ( 'NONE', #19090, 999.9999999999998863 ) ;
#7793=EDGE_CURVE ( 'NONE', #20799, #36282, #3921, .T. ) ;
#7795=DIRECTION ( 'NONE',  ( -1.000000000000000000, 0.000000000000000000, 0.000000000000000000 ) ) ;
#7798=CARTESIAN_POINT ( 'NONE',  ( -6.802008071587399840, 24.18409554641266368, 3.061616997868437868E-16 ) ) ;
#7801=EDGE_CURVE ( 'NONE', #32122, #46342, #69151, .T. ) ;
#7812=CARTESIAN_POINT ( 'NONE',  ( 0.000000000000000000, 0.000000000000000000, 170.0000000000000000 ) ) ;
#7813=CARTESIAN_POINT ( 'NONE',  ( -15.76129977463437015, -63.43731725181460490, 6.377659838150115899E-18 ) ) ;
#7819=LINE ( 'NONE', #16957, #43428 ) ;
#7824=ORIENTED_EDGE ( 'NONE', *, *, #59236, .T. ) ;
#7827=VERTEX_POINT ( 'NONE', #12089 ) ;
#7831=ORIENTED_EDGE ( 'NONE', *, *, #22808, .T. ) ;
#7848=AXIS2_PLACEMENT_3D ( 'NONE', #13443, #34905, #25043 ) ;
#7854=DIRECTION ( 'NONE',  ( 1.000000000000000000, 0.000000000000000000, 0.000000000000000000 ) ) ;
#7857=EDGE_CURVE ( 'NONE', #3570, #34941, #44074, .T. ) ;
#7862=ADVANCED_FACE ( 'NONE', ( #65558 ), #24036, .F. ) ;
#7885=CARTESIAN_POINT ( 'NONE',  ( 60.74750367560205433, 24.13405452624938263, 41.38025477438755928 ) ) ;
#7886=ORIENTED_EDGE ( 'NONE', *, *, #16289, .F. ) ;
#7887=CARTESIAN_POINT ( 'NONE',  ( -24.98026281234599821, -0.9932118737290694943, 0.000000000000000000 ) ) ;
#7904=ORIENTED_EDGE ( 'NONE', *, *, #34403, .F. ) ;
#7906=CARTESIAN_POINT ( 'NONE',  ( 0.000000000000000000, 0.000000000000000000, 41.38025477438755928 ) ) ;
#7916=VECTOR ( 'NONE', #15980, 1000.000000000000114 ) ;
#7937=LINE ( 'NONE', #49785, #59100 ) ;
#7939=EDGE_CURVE ( 'NONE', #21445, #26335, #17360, .T. ) ;
#7945=FACE_OUTER_BOUND ( 'NONE', #52953, .T. ) ;
#7949=DIRECTION ( 'NONE',  ( -0.000000000000000000, -0.000000000000000000, -1.000000000000000000 ) ) ;
#7952=ORIENTED_EDGE ( 'NONE', *, *, #23621, .T. ) ;
#7953=VERTEX_POINT ( 'NONE', #23351 ) ;
#7966=VERTEX_POINT ( 'NONE', #3960 ) ;
#7979=DIRECTION ( 'NONE',  ( -0.3930250316539278255, 0.9195277725514487965, 0.000000000000000000 ) ) ;
#7995=EDGE_LOOP ( 'NONE', ( #44128, #15177, #1749, #23395, #45298, #66615, #7298, #16890, #21287 ) ) ;
#7997=LINE ( 'NONE', #14657, #63208 ) ;
#7998=VERTEX_POINT ( 'NONE', #41585 ) ;
#8009=CIRCLE ( 'NONE', #47305, 24.99999999999985434 ) ;
#8019=VERTEX_POINT ( 'NONE', #68332 ) ;
#8021=EDGE_CURVE ( 'NONE', #64121, #47461, #45830, .T. ) ;
#8022=DIRECTION ( 'NONE',  ( -0.000000000000000000, -0.000000000000000000, -1.000000000000000000 ) ) ;
#8024=CARTESIAN_POINT ( 'NONE',  ( 36.30976089643145599, -12.29214613588890437, 13.32819299319724315 ) ) ;
#8026=CARTESIAN_POINT ( 'NONE',  ( 74.62299871641495486, 5.461138973199058277, 170.0000000000000000 ) ) ;
#8037=LINE ( 'NONE', #40391, #6272 ) ;
#8046=EDGE_LOOP ( 'NONE', ( #68631, #28224, #7212, #49726 ) ) ;
#8059=ORIENTED_EDGE ( 'NONE', *, *, #60836, .F. ) ;
#8065=DIRECTION ( 'NONE',  ( 1.000000000000000000, 0.000000000000000000, 0.000000000000000000 ) ) ;
#8066=CIRCLE ( 'NONE', #51896, 65.36598343705435354 ) ;
#8067=DIRECTION ( 'NONE',  ( -0.000000000000000000, 0.000000000000000000, 1.000000000000000000 ) ) ;
#8070=ORIENTED_EDGE ( 'NONE', *, *, #18337, .F. ) ;
#8077=ORIENTED_EDGE ( 'NONE', *, *, #28923, .T. ) ;
#8082=EDGE_CURVE ( 'NONE', #34211, #69123, #37682, .T. ) ;
#8087=LINE ( 'NONE', #52633, #52708 ) ;
#8090=ORIENTED_EDGE ( 'NONE', *, *, #46995, .F. ) ;
#8102=LINE ( 'NONE', #3183, #60118 ) ;
#8117=AXIS2_PLACEMENT_3D ( 'NONE', #8779, #24950, #35146 ) ;
#8119=ORIENTED_EDGE ( 'NONE', *, *, #45679, .F. ) ;
#8121=ORIENTED_EDGE ( 'NONE', *, *, #56214, .F. ) ;
#8123=ADVANCED_FACE ( 'NONE', ( #38034 ), #43337, .T. ) ;
#8126=DIRECTION ( 'NONE',  ( -0.000000000000000000, 0.000000000000000000, -1.000000000000000000 ) ) ;
#8129=EDGE_CURVE ( 'NONE', #15646, #4543, #15755, .T. ) ;
#8138=LINE ( 'NONE', #29581, #17587 ) ;
#8147=CARTESIAN_POINT ( 'NONE',  ( 0.000000000000000000, 0.000000000000000000, 0.000000000000000000 ) ) ;
#8151=LINE ( 'NONE', #45787, #52516 ) ;
#8152=LINE ( 'NONE', #7813, #47351 ) ;
#8153=AXIS2_PLACEMENT_3D ( 'NONE', #28579, #50389, #35242 ) ;
#8154=DIRECTION ( 'NONE',  ( -0.000000000000000000, -0.000000000000000000, -1.000000000000000000 ) ) ;
#8155=CARTESIAN_POINT ( 'NONE',  ( -13.24252603915519444, -63.63674649211960599, 170.0000000000000000 ) ) ;
#8158=CARTESIAN_POINT ( 'NONE',  ( 47.91750333461326505, 19.31887485910233693, 26.66469066592268788 ) ) ;
#8165=LINE ( 'NONE', #51079, #17116 ) ;
#8172=B_SPLINE_CURVE_WITH_KNOTS ( 'NONE', 3,
 ( #31564, #53000, #68507, #35815, #52663, #4824 ),
 .UNSPECIFIED., .F., .F.,
 ( 4, 2, 4 ),
 ( 1.095770181108053550E-06, 0.03239442681617710901, 0.06478775786217311206 ),
 .UNSPECIFIED. ) ;
#8173=VECTOR ( 'NONE', #19175, 999.9999999999998863 ) ;
#8177=DIRECTION ( 'NONE',  ( -0.000000000000000000, -0.000000000000000000, 1.000000000000000000 ) ) ;
#8179=EDGE_CURVE ( 'NONE', #5941, #36461, #45398, .T. ) ;
#8181=EDGE_CURVE ( 'NONE', #22856, #15204, #57002, .T. ) ;
#8185=CARTESIAN_POINT ( 'NONE',  ( 0.000000000000000000, 0.000000000000000000, 0.000000000000000000 ) ) ;
#8189=EDGE_LOOP ( 'NONE', ( #19372, #48459, #58598, #25923 ) ) ;
#8190=ORIENTED_EDGE ( 'NONE', *, *, #56333, .F. ) ;
#8195=LINE ( 'NONE', #13473, #43487 ) ;
#8205=DIRECTION ( 'NONE',  ( 1.000000000000000000, 0.000000000000000000, 0.000000000000000000 ) ) ;
#8221=ORIENTED_EDGE ( 'NONE', *, *, #53653, .T. ) ;
#8225=CARTESIAN_POINT ( 'NONE',  ( 70.34686579112810989, 18.11777090454213379, 43.58025477438756923 ) ) ;
#8230=LINE ( 'NONE', #51495, #27766 ) ;
#8240=ORIENTED_EDGE ( 'NONE', *, *, #46920, .T. ) ;
#8241=DIRECTION ( 'NONE',  ( 0.8584487936018655452, 0.5128992774059070170, -0.000000000000000000 ) ) ;
#8246=ORIENTED_EDGE ( 'NONE', *, *, #39070, .F. ) ;
#8252=EDGE_CURVE ( 'NONE', #2052, #62563, #42200, .T. ) ;
#8256=CARTESIAN_POINT ( 'NONE',  ( -61.36325649057781817, -43.03793052543183251, 41.38025477438755928 ) ) ;
#8257=VERTEX_POINT ( 'NONE', #31638 ) ;
#8267=VECTOR ( 'NONE', #63664, 1000.000000000000114 ) ;
#8269=ORIENTED_EDGE ( 'NONE', *, *, #40967, .T. ) ;
#8270=AXIS2_PLACEMENT_3D ( 'NONE', #36099, #30470, #9359 ) ;
#8271=CARTESIAN_POINT ( 'NONE',  ( -4.164416015345870470, 64.86646004871185767, 40.00000000000003553 ) ) ;
#8274=EDGE_CURVE ( 'NONE', #38050, #8339, #26588, .T. ) ;
#8283=B_SPLINE_CURVE_WITH_KNOTS ( 'NONE', 3,
 ( #47477, #21117, #6920, #52755, #47829, #69289 ),
 .UNSPECIFIED., .F., .F.,
 ( 4, 2, 4 ),
 ( 0.03218950539619248874, 0.06469844149454670457, 0.09720737759290090652 ),
 .UNSPECIFIED. ) ;
#8291=CARTESIAN_POINT ( 'NONE',  ( -65.20298343242136241, 4.613322252417249913, 43.58025477438756212 ) ) ;
#8292=ORIENTED_EDGE ( 'NONE', *, *, #46363, .T. ) ;
#8295=CARTESIAN_POINT ( 'NONE',  ( 56.42997683260104225, 32.25922681454269991, 40.00000000000003553 ) ) ;
#8300=EDGE_CURVE ( 'NONE', #28657, #37048, #49241, .T. ) ;
#8302=EDGE_LOOP ( 'NONE', ( #16523, #9461, #42713, #42175 ) ) ;
#8304=VERTEX_POINT ( 'NONE', #47122 ) ;
#8313=AXIS2_PLACEMENT_3D ( 'NONE', #32514, #53945, #58889 ) ;
#8319=DIRECTION ( 'NONE',  ( 1.000000000000000000, 0.000000000000000000, 0.000000000000000000 ) ) ;
#8322=CARTESIAN_POINT ( 'NONE',  ( -84.49322488516129681, 0.000000000000000000, 43.58025477438756212 ) ) ;
#8330=ORIENTED_EDGE ( 'NONE', *, *, #51938, .F. ) ;
#8339=VERTEX_POINT ( 'NONE', #68586 ) ;
#8342=DIRECTION ( 'NONE',  ( -0.000000000000000000, -0.000000000000000000, -1.000000000000000000 ) ) ;
#8346=VERTEX_POINT ( 'NONE', #4905 ) ;
#8349=EDGE_CURVE ( 'NONE', #10821, #58236, #42255, .T. ) ;
#8351=DIRECTION ( 'NONE',  ( 1.000000000000000000, 0.000000000000000000, 0.000000000000000000 ) ) ;
#8353=CARTESIAN_POINT ( 'NONE',  ( 15.68296563925497900, 63.09411298019765013, 41.38025477438755928 ) ) ;
#8361=EDGE_CURVE ( 'NONE', #36820, #54048, #51201, .T. ) ;
#8364=ORIENTED_EDGE ( 'NONE', *, *, #2786, .T. ) ;
#8370=VECTOR ( 'NONE', #67571, 1000.000000000000114 ) ;
#8371=AXIS2_PLACEMENT_3D ( 'NONE', #19317, #18977, #40772 ) ;
#8376=LINE ( 'NONE', #2746, #10414 ) ;
#8378=ORIENTED_EDGE ( 'NONE', *, *, #54533, .T. ) ;
#8383=FACE_OUTER_BOUND ( 'NONE', #40334, .T. ) ;
#8403=CYLINDRICAL_SURFACE ( 'NONE', #44286, 65.00000000000000000 ) ;
#8406=PLANE ( 'NONE',  #22093 ) ;
#8411=ORIENTED_EDGE ( 'NONE', *, *, #51326, .F. ) ;
#8420=VECTOR ( 'NONE', #15399, 1000.000000000000000 ) ;
#8455=ORIENTED_EDGE ( 'NONE', *, *, #8735, .T. ) ;
#8458=EDGE_LOOP ( 'NONE', ( #31773, #35346, #60835, #17573, #27613, #66102, #6422, #6758, #46827 ) ) ;
#8465=CARTESIAN_POINT ( 'NONE',  ( 10.73115448446747244, -22.57968829347487727, 0.000000000000000000 ) ) ;
#8468=VECTOR ( 'NONE', #11523, 1000.000000000000000 ) ;
#8474=ORIENTED_EDGE ( 'NONE', *, *, #37393, .T. ) ;
#8478=DIRECTION ( 'NONE',  ( -0.9959742939952397345, 0.08963930890342655666, 0.000000000000000000 ) ) ;
#8481=FACE_OUTER_BOUND ( 'NONE', #37348, .T. ) ;
#8483=EDGE_CURVE ( 'NONE', #36461, #52626, #670, .T. ) ;
#8486=ORIENTED_EDGE ( 'NONE', *, *, #63356, .T. ) ;
#8487=VERTEX_POINT ( 'NONE', #6637 ) ;
#8492=CARTESIAN_POINT ( 'NONE',  ( 0.000000000000000000, 0.000000000000000000, 170.0000000000000000 ) ) ;
#8494=CARTESIAN_POINT ( 'NONE',  ( -52.13778968636795241, 39.42540649521991014, 41.38025477438755928 ) ) ;
#8495=ORIENTED_EDGE ( 'NONE', *, *, #14115, .F. ) ;
#8502=EDGE_CURVE ( 'NONE', #49177, #18239, #25261, .T. ) ;
#8503=CONICAL_SURFACE ( 'NONE', #62425, 65.00000000000000000, 0.7853981633974497223 ) ;
#8532=ADVANCED_FACE ( 'NONE', ( #26966 ), #4485, .T. ) ;
#8535=ORIENTED_EDGE ( 'NONE', *, *, #35179, .T. ) ;
#8555=CIRCLE ( 'NONE', #48980, 65.36598343705435354 ) ;
#8559=EDGE_LOOP ( 'NONE', ( #50087, #52557, #32077, #58326 ) ) ;
#8565=CIRCLE ( 'NONE', #41142, 65.36598343705435354 ) ;
#8566=VECTOR ( 'NONE', #37739, 1000.000000000000000 ) ;
#8575=CONICAL_SURFACE ( 'NONE', #11911, 74.95140232871122521, 0.8777644062502172329 ) ;
#8577=DIRECTION ( 'NONE',  ( 0.1342332658176667304, -0.9909497617679331460, 0.000000000000000000 ) ) ;
#8593=ADVANCED_FACE ( 'NONE', ( #26633 ), #48067, .F. ) ;
#8604=DIRECTION ( 'NONE',  ( -1.000000000000000000, 0.000000000000000000, 0.000000000000000000 ) ) ;
#8608=DIRECTION ( 'NONE',  ( -0.000000000000000000, -0.000000000000000000, -1.000000000000000000 ) ) ;
#8611=ORIENTED_EDGE ( 'NONE', *, *, #8129, .T. ) ;
#8617=EDGE_CURVE ( 'NONE', #3858, #54158, #1284, .T. ) ;
#8634=ORIENTED_EDGE ( 'NONE', *, *, #44852, .F. ) ;
#8639=CARTESIAN_POINT ( 'NONE',  ( 0.000000000000000000, 0.000000000000000000, 41.38025477438755928 ) ) ;
#8647=FACE_BOUND ( 'NONE', #61958, .T. ) ;
#8657=ADVANCED_FACE ( 'NONE', ( #18768 ), #52392, .F. ) ;
#8659=DIRECTION ( 'NONE',  ( 0.2660368455666826670, -0.9639628606958512425, 2.500042656554809847E-16 ) ) ;
#8672=CARTESIAN_POINT ( 'NONE',  ( 58.32618558115825635, 1.250000000000015099, 27.58472369367762411 ) ) ;
#8676=EDGE_CURVE ( 'NONE', #64051, #24493, #60225, .T. ) ;
#8700=DIRECTION ( 'NONE',  ( -1.000000000000000000, 0.000000000000000000, 0.000000000000000000 ) ) ;
#8702=ORIENTED_EDGE ( 'NONE', *, *, #1380, .T. ) ;
#8706=ORIENTED_EDGE ( 'NONE', *, *, #36936, .T. ) ;
#8708=VECTOR ( 'NONE', #37798, 1000.000000000000114 ) ;
#8723=CARTESIAN_POINT ( 'NONE',  ( -63.89980862959375685, 18.93195709527340043, 34.48241795236666007 ) ) ;
#8724=DIRECTION ( 'NONE',  ( 0.4738686624729966379, 0.8805955318567391110, 0.000000000000000000 ) ) ;
#8725=ORIENTED_EDGE ( 'NONE', *, *, #7939, .F. ) ;
#8735=EDGE_CURVE ( 'NONE', #26073, #476, #51813, .T. ) ;
#8746=CARTESIAN_POINT ( 'NONE',  ( 44.01696072966020523, -47.84694004974148385, 41.38025477438755928 ) ) ;
#8750=CARTESIAN_POINT ( 'NONE',  ( -64.83840629396348731, 4.580509716059292913, 40.00000000000003553 ) ) ;
#8752=EDGE_LOOP ( 'NONE', ( #59293, #45483, #44314, #27129 ) ) ;
#8756=EDGE_CURVE ( 'NONE', #9333, #4577, #44511, .T. ) ;
#8757=CARTESIAN_POINT ( 'NONE',  ( 24.39800339187929268, -60.26242556095670722, 3.061616997868437868E-16 ) ) ;
#8761=B_SPLINE_CURVE_WITH_KNOTS ( 'NONE', 3,
 ( #6158, #44504, #50480, #6868, #28317, #65983 ),
 .UNSPECIFIED., .F., .F.,
 ( 4, 2, 4 ),
 ( 0.03218936187311347702, 0.06469833704501401495, 0.09720731221691455981 ),
 .UNSPECIFIED. ) ;
#8765=VECTOR ( 'NONE', #33584, 1000.000000000000000 ) ;
#8769=VERTEX_POINT ( 'NONE', #29241 ) ;
#8774=CARTESIAN_POINT ( 'NONE',  ( 61.62594073580542897, 21.79346734965000820, 41.38025477438755928 ) ) ;
#8779=CARTESIAN_POINT ( 'NONE',  ( 0.000000000000000000, 0.000000000000000000, 170.0000000000000000 ) ) ;
#8781=DIRECTION ( 'NONE',  ( 1.807017991507195025E-16, 1.727686100818934983E-16, 1.000000000000000000 ) ) ;
#8790=VERTEX_POINT ( 'NONE', #38753 ) ;
#8814=CARTESIAN_POINT ( 'NONE',  ( 4.590321433068643486, 24.57496590315240681, 0.000000000000000000 ) ) ;
#8815=CARTESIAN_POINT ( 'NONE',  ( -16.43619359402630664, 18.99971924381106092, 0.000000000000000000 ) ) ;
#8819=DIRECTION ( 'NONE',  ( 1.000000000000000000, 0.000000000000000000, 0.000000000000000000 ) ) ;
#8830=DIRECTION ( 'NONE',  ( -0.1785568947986229116, -0.9839295885986321100, 5.102127870520020458E-18 ) ) ;
#8831=EDGE_CURVE ( 'NONE', #26680, #67396, #34872, .T. ) ;
#8846=ORIENTED_EDGE ( 'NONE', *, *, #61382, .T. ) ;
#8854=CIRCLE ( 'NONE', #68399, 65.36598343705435354 ) ;
#8864=PLANE ( 'NONE',  #51684 ) ;
#8875=DIRECTION ( 'NONE',  ( 1.000000000000000000, 0.000000000000000000, 0.000000000000000000 ) ) ;
#8876=VERTEX_POINT ( 'NONE', #49991 ) ;
#8885=ORIENTED_EDGE ( 'NONE', *, *, #56327, .F. ) ;
#8888=DIRECTION ( 'NONE',  ( -0.000000000000000000, -0.000000000000000000, -1.000000000000000000 ) ) ;
#8892=CARTESIAN_POINT ( 'NONE',  ( -59.89379335984659747, -45.06047301136921135, 41.38025477438755928 ) ) ;
#8894=EDGE_CURVE ( 'NONE', #35154, #57513, #7446, .T. ) ;
#8898=ORIENTED_EDGE ( 'NONE', *, *, #15653, .T. ) ;
#8900=ORIENTED_EDGE ( 'NONE', *, *, #31356, .F. ) ;
#8904=DIRECTION ( 'NONE',  ( 1.000000000000000000, 0.000000000000000000, 0.000000000000000000 ) ) ;
#8910=VECTOR ( 'NONE', #60487, 1000.000000000000000 ) ;
#8918=CARTESIAN_POINT ( 'NONE',  ( -55.15976438495157197, 34.41253982194030669, 170.0000000000000000 ) ) ;
#8924=ADVANCED_FACE ( 'NONE', ( #1461 ), #22916, .T. ) ;
#8926=CARTESIAN_POINT ( 'NONE',  ( 65.78600657349682024, 10.66798394579848619, 34.48241795236667429 ) ) ;
#8936=DIRECTION ( 'NONE',  ( -1.000000000000000000, 0.000000000000000000, 0.000000000000000000 ) ) ;
#8942=ORIENTED_EDGE ( 'NONE', *, *, #554, .F. ) ;
#8946=ORIENTED_EDGE ( 'NONE', *, *, #40571, .F. ) ;
#8947=CARTESIAN_POINT ( 'NONE',  ( 60.40479419793796012, -24.00543350795314979, 170.0000000000000000 ) ) ;
#8962=ORIENTED_EDGE ( 'NONE', *, *, #15500, .F. ) ;
#8972=AXIS2_PLACEMENT_3D ( 'NONE', #69350, #749, #59475 ) ;
#8978=DIRECTION ( 'NONE',  ( -0.8805955318567322276, -0.4738686624730095165, 5.102127870520022769E-18 ) ) ;
#8991=ADVANCED_FACE ( 'NONE', ( #8481 ), #3537, .T. ) ;
#8998=ORIENTED_EDGE ( 'NONE', *, *, #12701, .T. ) ;
#9000=B_SPLINE_CURVE_WITH_KNOTS ( 'NONE', 3,
 ( #64060, #68980, #26089, #15872 ),
 .UNSPECIFIED., .F., .F.,
 ( 4, 4 ),
 ( 9.900409499073836656E-07, 0.05658314289920116785 ),
 .UNSPECIFIED. ) ;
#9008=EDGE_CURVE ( 'NONE', #51470, #61262, #35530, .T. ) ;
#9016=CARTESIAN_POINT ( 'NONE',  ( 56.48035995027075273, 49.34540444547854321, 0.000000000000000000 ) ) ;
#9019=DIRECTION ( 'NONE',  ( 1.000000000000000000, 0.000000000000000000, 0.000000000000000000 ) ) ;
#9022=EDGE_LOOP ( 'NONE', ( #61019, #60838, #58387, #58725 ) ) ;
#9024=VECTOR ( 'NONE', #36147, 1000.000000000000114 ) ;
#9027=CARTESIAN_POINT ( 'NONE',  ( -40.27405704175634327, 63.28161525591265502, 43.58025477438756212 ) ) ;
#9030=ORIENTED_EDGE ( 'NONE', *, *, #32388, .F. ) ;
#9035=VERTEX_POINT ( 'NONE', #5598 ) ;
#9044=CARTESIAN_POINT ( 'NONE',  ( 5.694488383565878387, -51.35054909896783215, 26.66469104408690427 ) ) ;
#9052=PLANE ( 'NONE',  #27410 ) ;
#9054=ORIENTED_EDGE ( 'NONE', *, *, #40444, .T. ) ;
#9055=CARTESIAN_POINT ( 'NONE',  ( 48.39383208188445451, -43.94028683479019293, 6.377659838150144402E-18 ) ) ;
#9056=EDGE_CURVE ( 'NONE', #28933, #68971, #64345, .T. ) ;
#9058=CARTESIAN_POINT ( 'NONE',  ( 10.01137213834874196, 64.59476928204604462, 41.38025477438755928 ) ) ;
#9061=ORIENTED_EDGE ( 'NONE', *, *, #49882, .T. ) ;
#9064=VECTOR ( 'NONE', #16328, 1000.000000000000227 ) ;
#9069=CARTESIAN_POINT ( 'NONE',  ( -52.73319225379935205, 53.34578647582052469, 170.0000000000000000 ) ) ;
#9070=CARTESIAN_POINT ( 'NONE',  ( -49.77357484059193382, 41.82599373102802787, 170.0000000000000000 ) ) ;
#9072=DIRECTION ( 'NONE',  ( 4.691548276051942630E-18, 2.005263967813518922E-18, -1.000000000000000000 ) ) ;
#9075=ORIENTED_EDGE ( 'NONE', *, *, #10851, .F. ) ;
#9088=AXIS2_PLACEMENT_3D ( 'NONE', #64615, #16427, #5182 ) ;
#9094=PLANE ( 'NONE',  #68854 ) ;
#9100=CARTESIAN_POINT ( 'NONE',  ( 12.93264331410902379, 21.39501663729252456, 0.000000000000000000 ) ) ;
#9104=CARTESIAN_POINT ( 'NONE',  ( -24.51966494718099909, -5.470267094204724678, 0.000000000000000000 ) ) ;
#9128=ADVANCED_FACE ( 'NONE', ( #59746 ), #38661, .T. ) ;
#9137=CARTESIAN_POINT ( 'NONE',  ( 12.99074365121454910, -21.50298515537749822, 3.061616997868437868E-16 ) ) ;
#9139=DIRECTION ( 'NONE',  ( -0.9959742939952382912, -0.08963930890344089242, 0.000000000000000000 ) ) ;
#9145=ORIENTED_EDGE ( 'NONE', *, *, #44739, .F. ) ;
#9148=EDGE_CURVE ( 'NONE', #11003, #56134, #41202, .T. ) ;
#9153=CARTESIAN_POINT ( 'NONE',  ( -84.49322488516129681, 0.000000000000000000, 43.58025477438756212 ) ) ;
#9160=VERTEX_POINT ( 'NONE', #61164 ) ;
#9165=VECTOR ( 'NONE', #61009, 1000.000000000000114 ) ;
#9173=ORIENTED_EDGE ( 'NONE', *, *, #26128, .T. ) ;
#9176=AXIS2_PLACEMENT_3D ( 'NONE', #37315, #10933, #65458 ) ;
#9179=DIRECTION ( 'NONE',  ( 0.000000000000000000, 0.000000000000000000, 1.000000000000000000 ) ) ;
#9189=ORIENTED_EDGE ( 'NONE', *, *, #18185, .T. ) ;
#9196=EDGE_CURVE ( 'NONE', #33759, #48517, #23237, .T. ) ;
#9197=ORIENTED_EDGE ( 'NONE', *, *, #7793, .F. ) ;
#9207=ORIENTED_EDGE ( 'NONE', *, *, #13430, .F. ) ;
#9208=ADVANCED_FACE ( 'NONE', ( #54827 ), #12279, .F. ) ;
#9212=CARTESIAN_POINT ( 'NONE',  ( 21.96921518829188358, 71.65937688154191676, 41.38025477438755928 ) ) ;
#9223=AXIS2_PLACEMENT_3D ( 'NONE', #43882, #27361, #33710 ) ;
#9228=LINE ( 'NONE', #42610, #30904 ) ;
#9232=CARTESIAN_POINT ( 'NONE',  ( 0.000000000000000000, 0.000000000000000000, 0.000000000000000000 ) ) ;
#9242=ORIENTED_EDGE ( 'NONE', *, *, #623, .F. ) ;
#9247=CARTESIAN_POINT ( 'NONE',  ( 9.962235950565768050, -64.23203137738408941, 170.0000000000000000 ) ) ;
#9254=ORIENTED_EDGE ( 'NONE', *, *, #31048, .F. ) ;
#9259=AXIS2_PLACEMENT_3D ( 'NONE', #66754, #11872, #65345 ) ;
#9263=CARTESIAN_POINT ( 'NONE',  ( 73.95984195137785377, 12.15131637179898583, 41.38025477438755928 ) ) ;
#9265=VECTOR ( 'NONE', #66787, 1000.000000000000000 ) ;
#9269=DIRECTION ( 'NONE',  ( -0.000000000000000000, -0.000000000000000000, -1.000000000000000000 ) ) ;
#9277=DIRECTION ( 'NONE',  ( -1.000000000000000000, 0.000000000000000000, 0.000000000000000000 ) ) ;
#9278=LINE ( 'NONE', #4354, #27716 ) ;
#9279=ORIENTED_EDGE ( 'NONE', *, *, #56136, .T. ) ;
#9282=EDGE_CURVE ( 'NONE', #18239, #35316, #46068, .T. ) ;
#9285=LINE ( 'NONE', #30748, #60009 ) ;
#9288=VERTEX_POINT ( 'NONE', #45729 ) ;
#9292=ADVANCED_FACE ( 'NONE', ( #67539 ), #61893, .T. ) ;
#9307=PLANE ( 'NONE',  #59991 ) ;
#9308=ORIENTED_EDGE ( 'NONE', *, *, #56633, .T. ) ;
#9311=CIRCLE ( 'NONE', #48589, 65.00000000000000000 ) ;
#9314=FACE_OUTER_BOUND ( 'NONE', #66410, .T. ) ;
#9316=AXIS2_PLACEMENT_3D ( 'NONE', #41620, #9962, #53538 ) ;
#9317=FACE_OUTER_BOUND ( 'NONE', #39668, .T. ) ;
#9320=VECTOR ( 'NONE', #36694, 1000.000000000000000 ) ;
#9330=CARTESIAN_POINT ( 'NONE',  ( -59.09450113343241640, 27.07101652673493319, 170.0000000000000000 ) ) ;
#9333=VERTEX_POINT ( 'NONE', #19335 ) ;
#9334=ORIENTED_EDGE ( 'NONE', *, *, #16653, .T. ) ;
#9335=DIRECTION ( 'NONE',  ( -0.000000000000000000, -2.500042656554809847E-16, 1.000000000000000000 ) ) ;
#9343=EDGE_CURVE ( 'NONE', #36820, #23240, #46407, .T. ) ;
#9348=CARTESIAN_POINT ( 'NONE',  ( -17.89459634713042391, -72.78390022947110083, 41.38025477438755928 ) ) ;
#9355=VERTEX_POINT ( 'NONE', #40448 ) ;
#9356=CONICAL_SURFACE ( 'NONE', #62123, 74.95140232871122521, 0.8777644062502172329 ) ;
#9359=DIRECTION ( 'NONE',  ( -0.3090169943749446757, -0.9510565162951544194, 0.000000000000000000 ) ) ;
#9363=ORIENTED_EDGE ( 'NONE', *, *, #29015, .F. ) ;
#9369=VECTOR ( 'NONE', #31257, 999.9999999999998863 ) ;
#9373=AXIS2_PLACEMENT_3D ( 'NONE', #52520, #9269, #4346 ) ;
#9377=CARTESIAN_POINT ( 'NONE',  ( 10.01137213834873840, 64.59476928204603041, 6.377659838150142862E-18 ) ) ;
#9383=CARTESIAN_POINT ( 'NONE',  ( -67.03031041878421092, -33.66749151869542089, 170.0000000000000000 ) ) ;
#9385=DIRECTION ( 'NONE',  ( 0.8090169943749506709, -0.5877852522924686962, 0.000000000000000000 ) ) ;
#9387=ORIENTED_EDGE ( 'NONE', *, *, #41155, .F. ) ;
#9389=LINE ( 'NONE', #68804, #60559 ) ;
#9396=EDGE_CURVE ( 'NONE', #20231, #41387, #26009, .T. ) ;
#9402=LINE ( 'NONE', #10084, #56701 ) ;
#9407=ORIENTED_EDGE ( 'NONE', *, *, #34558, .T. ) ;
#9408=VERTEX_POINT ( 'NONE', #47436 ) ;
#9416=CARTESIAN_POINT ( 'NONE',  ( -52.73319225379935205, 53.34578647582052469, 170.0000000000000000 ) ) ;
#9422=CIRCLE ( 'NONE', #17287, 65.36598343705435354 ) ;
#9423=DIRECTION ( 'NONE',  ( 0.9362348706397418674, -0.3513748240813305279, 0.000000000000000000 ) ) ;
#9429=DIRECTION ( 'NONE',  ( -3.356887510711391189E-18, -3.842266915190438346E-18, -1.000000000000000000 ) ) ;
#9435=EDGE_LOOP ( 'NONE', ( #37837, #56480, #17568, #28156 ) ) ;
#9444=ADVANCED_FACE ( 'NONE', ( #4206 ), #64318, .F. ) ;
#9460=ADVANCED_FACE ( 'NONE', ( #41493 ), #52389, .F. ) ;
#9461=ORIENTED_EDGE ( 'NONE', *, *, #9148, .F. ) ;
#9465=CARTESIAN_POINT ( 'NONE',  ( -13.32397999417977630, -63.99361958670536410, 41.38025477438755928 ) ) ;
#9474=AXIS2_PLACEMENT_3D ( 'NONE', #35507, #30576, #20026 ) ;
#9477=ORIENTED_EDGE ( 'NONE', *, *, #4191, .T. ) ;
#9483=ORIENTED_EDGE ( 'NONE', *, *, #29794, .T. ) ;
#9484=EDGE_CURVE ( 'NONE', #33479, #66025, #52573, .T. ) ;
#9487=ORIENTED_EDGE ( 'NONE', *, *, #40703, .T. ) ;
#9497=LINE ( 'NONE', #36918, #5430 ) ;
#9506=ORIENTED_EDGE ( 'NONE', *, *, #24050, .F. ) ;
#9509=LINE ( 'NONE', #14445, #27139 ) ;
#9520=CIRCLE ( 'NONE', #61190, 25.12245591505646303 ) ;
#9524=CARTESIAN_POINT ( 'NONE',  ( -14.79841479960619921, -20.14961338137257840, 0.000000000000000000 ) ) ;
#9529=CARTESIAN_POINT ( 'NONE',  ( -4.610955605662443446, -74.80943656680585718, 41.38025477438755928 ) ) ;
#9535=ADVANCED_FACE ( 'NONE', ( #11190 ), #34491, .T. ) ;
#9537=ORIENTED_EDGE ( 'NONE', *, *, #30277, .T. ) ;
#9539=ORIENTED_EDGE ( 'NONE', *, *, #37765, .T. ) ;
#9540=LINE ( 'NONE', #36267, #46898 ) ;
#9543=CARTESIAN_POINT ( 'NONE',  ( 36.64089410029665572, -65.45232906116368099, 43.58025477438756923 ) ) ;
#9546=ADVANCED_FACE ( 'NONE', ( #48454 ), #33714, .T. ) ;
#9552=ORIENTED_EDGE ( 'NONE', *, *, #47627, .F. ) ;
#9553=CIRCLE ( 'NONE', #33092, 74.95140232871122521 ) ;
#9555=ORIENTED_EDGE ( 'NONE', *, *, #12386, .T. ) ;
#9557=ORIENTED_EDGE ( 'NONE', *, *, #21995, .F. ) ;
#9561=VECTOR ( 'NONE', #10952, 1000.000000000000000 ) ;
#9562=CIRCLE ( 'NONE', #38787, 65.36598343705435354 ) ;
#9573=CARTESIAN_POINT ( 'NONE',  ( 31.89651141207536256, 56.63578868294628421, 40.00000000000003553 ) ) ;
#9578=DIRECTION ( 'NONE',  ( -0.000000000000000000, -0.000000000000000000, -1.000000000000000000 ) ) ;
#9582=FACE_OUTER_BOUND ( 'NONE', #17935, .T. ) ;
#9590=CARTESIAN_POINT ( 'NONE',  ( 7.533997733928853968, 64.93035244659016314, 3.125053320693570118E-16 ) ) ;
#9592=CARTESIAN_POINT ( 'NONE',  ( 33.18066491647863359, 39.60239344302862463, 26.66469104408689006 ) ) ;
#9593=FACE_OUTER_BOUND ( 'NONE', #41307, .T. ) ;
#9603=ADVANCED_FACE ( 'NONE', ( #6968 ), #21745, .T. ) ;
#9606=AXIS2_PLACEMENT_3D ( 'NONE', #25752, #20451, #56362 ) ;
#9607=DIRECTION ( 'NONE',  ( -0.000000000000000000, -0.000000000000000000, -1.000000000000000000 ) ) ;
#9608=FACE_OUTER_BOUND ( 'NONE', #62403, .T. ) ;
#9610=EDGE_CURVE ( 'NONE', #64530, #23937, #1367, .T. ) ;
#9624=AXIS2_PLACEMENT_3D ( 'NONE', #23338, #28241, #65189 ) ;
#9625=ADVANCED_FACE ( 'NONE', ( #27720 ), #17598, .T. ) ;
#9629=LINE ( 'NONE', #52527, #42875 ) ;
#9633=LINE ( 'NONE', #68037, #53713 ) ;
#9634=CARTESIAN_POINT ( 'NONE',  ( -28.32746765835526048, 69.45586423092609607, 73.58025477438756923 ) ) ;
#9635=ORIENTED_EDGE ( 'NONE', *, *, #65097, .F. ) ;
#9639=ORIENTED_EDGE ( 'NONE', *, *, #18014, .T. ) ;
#9641=CARTESIAN_POINT ( 'NONE',  ( 0.000000000000000000, 0.000000000000000000, 0.000000000000000000 ) ) ;
#9652=AXIS2_PLACEMENT_3D ( 'NONE', #15105, #11446, #36563 ) ;
#9661=ORIENTED_EDGE ( 'NONE', *, *, #8181, .T. ) ;
#9663=VECTOR ( 'NONE', #10297, 1000.000000000000114 ) ;
#9678=CARTESIAN_POINT ( 'NONE',  ( -26.83517958587657404, 59.60356471962912650, 43.58025477438756212 ) ) ;
#9687=EDGE_CURVE ( 'NONE', #24552, #31912, #61812, .T. ) ;
#9691=DIRECTION ( 'NONE',  ( -0.000000000000000000, -0.000000000000000000, -1.000000000000000000 ) ) ;
#9693=EDGE_CURVE ( 'NONE', #14491, #37440, #37155, .T. ) ;
#9702=CARTESIAN_POINT ( 'NONE',  ( 0.000000000000000000, 0.000000000000000000, 41.38025477438755928 ) ) ;
#9706=VECTOR ( 'NONE', #65918, 999.9999999999998863 ) ;
#9707=ADVANCED_FACE ( 'NONE', ( #42092 ), #3769, .T. ) ;
#9725=B_SPLINE_CURVE_WITH_KNOTS ( 'NONE', 3,
 ( #59985, #5493, #6880, #1258 ),
 .UNSPECIFIED., .F., .F.,
 ( 4, 4 ),
 ( 9.900409499046083621E-07, 0.05658314289920115397 ),
 .UNSPECIFIED. ) ;
#9733=ORIENTED_EDGE ( 'NONE', *, *, #53016, .F. ) ;
#9741=ORIENTED_EDGE ( 'NONE', *, *, #56244, .T. ) ;
#9746=CARTESIAN_POINT ( 'NONE',  ( 73.51344971438123821, 14.61114034329559352, 41.38025477438755928 ) ) ;
#9752=LINE ( 'NONE', #36482, #19412 ) ;
#9754=VERTEX_POINT ( 'NONE', #9746 ) ;
#9755=AXIS2_PLACEMENT_3D ( 'NONE', #25964, #15745, #21029 ) ;
#9759=AXIS2_PLACEMENT_3D ( 'NONE', #52665, #61834, #13660 ) ;
#9771=AXIS2_PLACEMENT_3D ( 'NONE', #27025, #28067, #33370 ) ;
#9772=LINE ( 'NONE', #8746, #66676 ) ;
#9773=CARTESIAN_POINT ( 'NONE',  ( 62.82395662043622764, -22.24309023158800613, 34.48241823985147647 ) ) ;
#9774=DIRECTION ( 'NONE',  ( -1.000000000000000000, 0.000000000000000000, 0.000000000000000000 ) ) ;
#9782=VERTEX_POINT ( 'NONE', #33284 ) ;
#9784=CARTESIAN_POINT ( 'NONE',  ( -22.17966026246265798, -25.00691441576276475, 6.893342939543525283 ) ) ;
#9786=DIRECTION ( 'NONE',  ( 0.000000000000000000, 0.000000000000000000, 1.000000000000000000 ) ) ;
#9790=ADVANCED_FACE ( 'NONE', ( #11111 ), #54713, .T. ) ;
#9797=EDGE_CURVE ( 'NONE', #59256, #31208, #60349, .T. ) ;
#9813=CARTESIAN_POINT ( 'NONE',  ( -26.69131247781301752, 59.26697088776972322, 40.00000000000003553 ) ) ;
#9820=CIRCLE ( 'NONE', #38991, 74.95140232871122521 ) ;
#9830=EDGE_CURVE ( 'NONE', #10821, #26782, #9725, .T. ) ;
#9851=EDGE_CURVE ( 'NONE', #42925, #42894, #53670, .T. ) ;
#9855=ORIENTED_EDGE ( 'NONE', *, *, #34557, .T. ) ;
#9874=CARTESIAN_POINT ( 'NONE',  ( -53.17301597236439648, 40.17754241810537508, 34.48241795236665297 ) ) ;
#9875=VECTOR ( 'NONE', #30686, 1000.000000000000000 ) ;
#9879=EDGE_CURVE ( 'NONE', #44841, #47929, #65278, .T. ) ;
#9892=CARTESIAN_POINT ( 'NONE',  ( -9.964117946888929822, -64.24592483216726180, 170.0000000000000000 ) ) ;
#9893=CARTESIAN_POINT ( 'NONE',  ( -67.03031041878421092, -33.66749151869542089, 170.0000000000000000 ) ) ;
#9915=CARTESIAN_POINT ( 'NONE',  ( 69.77839676787897361, -27.52340539439948586, 43.58025477438756212 ) ) ;
#9917=DIRECTION ( 'NONE',  ( 1.000000000000000000, 0.000000000000000000, 0.000000000000000000 ) ) ;
#9923=LINE ( 'NONE', #31378, #51446 ) ;
#9926=CARTESIAN_POINT ( 'NONE',  ( 49.76301652092167416, 41.81676920493115546, 40.00000000000003553 ) ) ;
#9928=CARTESIAN_POINT ( 'NONE',  ( -84.49322488516129681, 0.000000000000000000, 43.58025477438756212 ) ) ;
#9929=DIRECTION ( 'NONE',  ( -0.000000000000000000, -0.000000000000000000, 1.000000000000000000 ) ) ;
#9931=DIRECTION ( 'NONE',  ( -0.2225209339563042066, -0.9749279121818259508, 0.000000000000000000 ) ) ;
#9934=VERTEX_POINT ( 'NONE', #29730 ) ;
#9940=DIRECTION ( 'NONE',  ( 1.000000000000000000, 0.000000000000000000, 0.000000000000000000 ) ) ;
#9947=PLANE ( 'NONE',  #20610 ) ;
#9950=AXIS2_PLACEMENT_3D ( 'NONE', #28749, #6938, #12221 ) ;
#9952=DIRECTION ( 'NONE',  ( -1.000000000000000000, 0.000000000000000000, 0.000000000000000000 ) ) ;
#9954=AXIS2_PLACEMENT_3D ( 'NONE', #6517, #12491, #64560 ) ;
#9957=EDGE_CURVE ( 'NONE', #67298, #12758, #18832, .T. ) ;
#9958=CIRCLE ( 'NONE', #63879, 74.95140232871122521 ) ;
#9962=DIRECTION ( 'NONE',  ( 0.000000000000000000, 0.000000000000000000, 1.000000000000000000 ) ) ;
#9981=ORIENTED_EDGE ( 'NONE', *, *, #936, .F. ) ;
#9987=CARTESIAN_POINT ( 'NONE',  ( 0.000000000000000000, 0.000000000000000000, 41.38025477438755928 ) ) ;
#9993=EDGE_CURVE ( 'NONE', #26796, #35022, #9820, .T. ) ;
#9996=EDGE_CURVE ( 'NONE', #19095, #33531, #42012, .T. ) ;
#10000=VECTOR ( 'NONE', #66938, 1000.000000000000000 ) ;
#10019=ADVANCED_FACE ( 'NONE', ( #30776 ), #69069, .F. ) ;
#10025=FACE_OUTER_BOUND ( 'NONE', #69535, .T. ) ;
#10026=CARTESIAN_POINT ( 'NONE',  ( 57.30278335769610010, -48.40406511297319980, 170.0000000000000000 ) ) ;
#10040=CARTESIAN_POINT ( 'NONE',  ( 0.000000000000000000, 0.000000000000000000, 40.00000000000003553 ) ) ;
#10041=CARTESIAN_POINT ( 'NONE',  ( -23.85457283326439182, 7.880174245944055578, 0.000000000000000000 ) ) ;
#10044=VECTOR ( 'NONE', #69152, 1000.000000000000000 ) ;
#10054=ORIENTED_EDGE ( 'NONE', *, *, #46476, .F. ) ;
#10059=ORIENTED_EDGE ( 'NONE', *, *, #9879, .F. ) ;
#10063=AXIS2_PLACEMENT_3D ( 'NONE', #42440, #21325, #58605 ) ;
#10067=LINE ( 'NONE', #47681, #47701 ) ;
#10068=EDGE_LOOP ( 'NONE', ( #22843, #39530, #33720, #46263 ) ) ;
#10069=CARTESIAN_POINT ( 'NONE',  ( 7.484861546145933353, -64.56761454192826477, 40.00000000000003553 ) ) ;
#10075=DIRECTION ( 'NONE',  ( -0.4738686624729966379, -0.8805955318567391110, 0.000000000000000000 ) ) ;
#10081=AXIS2_PLACEMENT_3D ( 'NONE', #28798, #33727, #49888 ) ;
#10084=CARTESIAN_POINT ( 'NONE',  ( 64.08056813503712590, -12.89932471814424630, 6.377659838150142091E-18 ) ) ;
#10088=ORIENTED_EDGE ( 'NONE', *, *, #2190, .F. ) ;
#10091=AXIS2_PLACEMENT_3D ( 'NONE', #19078, #25063, #20119 ) ;
#10096=B_SPLINE_CURVE_WITH_KNOTS ( 'NONE', 3,
 ( #33418, #17209, #1751, #28832, #23212, #60483 ),
 .UNSPECIFIED., .F., .F.,
 ( 4, 2, 4 ),
 ( 1.095770181117027441E-06, 0.03239442681617711595, 0.06478775786217311206 ),
 .UNSPECIFIED. ) ;
#10097=DIRECTION ( 'NONE',  ( 0.8345732537212999791, 0.5508969814521065267, 5.102127870520020458E-18 ) ) ;
#10103=ORIENTED_EDGE ( 'NONE', *, *, #20727, .F. ) ;
#10109=CARTESIAN_POINT ( 'NONE',  ( 57.30278335769610010, -48.40406511297319980, 170.0000000000000000 ) ) ;
#10111=CARTESIAN_POINT ( 'NONE',  ( -45.81425895439360829, -46.10914959592906115, 40.00000000000003553 ) ) ;
#10115=VERTEX_POINT ( 'NONE', #35712 ) ;
#10123=CARTESIAN_POINT ( 'NONE',  ( 31.89651141207536256, 56.63578868294628421, 40.00000000000003553 ) ) ;
#10130=DIRECTION ( 'NONE',  ( 0.7530714660036196273, -0.6579387259397027066, 0.000000000000000000 ) ) ;
#10146=DIRECTION ( 'NONE',  ( -0.000000000000000000, -0.000000000000000000, -1.000000000000000000 ) ) ;
#10151=LINE ( 'NONE', #53739, #48537 ) ;
#10152=CARTESIAN_POINT ( 'NONE',  ( -1.666933348991701536, -64.97862212458815634, 40.00000000000003553 ) ) ;
#10165=EDGE_CURVE ( 'NONE', #45811, #48517, #60916, .T. ) ;
#10171=CARTESIAN_POINT ( 'NONE',  ( -30.60309003827877916, -68.41902945196855512, 41.38025477438755928 ) ) ;
#10173=FACE_OUTER_BOUND ( 'NONE', #18433, .T. ) ;
#10180=LINE ( 'NONE', #35549, #65555 ) ;
#10187=ORIENTED_EDGE ( 'NONE', *, *, #56064, .T. ) ;
#10191=ORIENTED_EDGE ( 'NONE', *, *, #4290, .F. ) ;
#10197=AXIS2_PLACEMENT_3D ( 'NONE', #17463, #33320, #22050 ) ;
#10198=VERTEX_POINT ( 'NONE', #36049 ) ;
#10208=AXIS2_PLACEMENT_3D ( 'NONE', #196, #555, #65630 ) ;
#10209=LINE ( 'NONE', #53455, #45008 ) ;
#10213=LINE ( 'NONE', #31679, #44638 ) ;
#10228=ORIENTED_EDGE ( 'NONE', *, *, #54067, .F. ) ;
#10241=ADVANCED_FACE ( 'NONE', ( #69429 ), #42694, .T. ) ;
#10246=EDGE_CURVE ( 'NONE', #28008, #44519, #64280, .T. ) ;
#10248=EDGE_CURVE ( 'NONE', #36451, #3230, #48637, .T. ) ;
#10252=DIRECTION ( 'NONE',  ( -0.000000000000000000, -0.000000000000000000, -1.000000000000000000 ) ) ;
#10265=FACE_OUTER_BOUND ( 'NONE', #29897, .T. ) ;
#10274=CARTESIAN_POINT ( 'NONE',  ( -84.49322488516129681, 0.000000000000000000, 43.58025477438756212 ) ) ;
#10287=CARTESIAN_POINT ( 'NONE',  ( 14.72760828316778259, -30.00634389893561504, 6.893343212288930211 ) ) ;
#10289=CARTESIAN_POINT ( 'NONE',  ( 0.000000000000000000, 0.000000000000000000, 41.38025477438755928 ) ) ;
#10297=DIRECTION ( 'NONE',  ( 0.9839295885986321100, -0.1785568947986229116, 0.000000000000000000 ) ) ;
#10298=CARTESIAN_POINT ( 'NONE',  ( 0.000000000000000000, 0.000000000000000000, 133.5802547743875550 ) ) ;
#10301=ORIENTED_EDGE ( 'NONE', *, *, #45433, .T. ) ;
#10306=ORIENTED_EDGE ( 'NONE', *, *, #17243, .T. ) ;
#10308=VECTOR ( 'NONE', #32015, 1000.000000000000114 ) ;
#10316=PLANE ( 'NONE',  #35620 ) ;
#10317=DIRECTION ( 'NONE',  ( -0.000000000000000000, -0.000000000000000000, 1.000000000000000000 ) ) ;
#10330=LINE ( 'NONE', #37071, #38845 ) ;
#10335=ORIENTED_EDGE ( 'NONE', *, *, #43559, .T. ) ;
#10343=LINE ( 'NONE', #20910, #58937 ) ;
#10346=ORIENTED_EDGE ( 'NONE', *, *, #9196, .T. ) ;
#10352=AXIS2_PLACEMENT_3D ( 'NONE', #57064, #8177, #8875 ) ;
#10353=CARTESIAN_POINT ( 'NONE',  ( 38.07387128079424343, 34.92400860923387995, 26.66469066592269144 ) ) ;
#10357=EDGE_LOOP ( 'NONE', ( #38129, #68885, #33719, #14622 ) ) ;
#10358=ORIENTED_EDGE ( 'NONE', *, *, #48041, .F. ) ;
#10359=AXIS2_PLACEMENT_3D ( 'NONE', #14524, #47900, #4323 ) ;
#10361=CARTESIAN_POINT ( 'NONE',  ( -17.89459634713042391, -72.78390022947110083, 41.38025477438755928 ) ) ;
#10362=CIRCLE ( 'NONE', #49673, 24.99999999999985434 ) ;
#10365=ORIENTED_EDGE ( 'NONE', *, *, #38334, .F. ) ;
#10368=CARTESIAN_POINT ( 'NONE',  ( 8.171862787985018528, 51.01496593442378469, 26.66469104408689716 ) ) ;
#10369=CARTESIAN_POINT ( 'NONE',  ( 28.73969565797881387, 50.76944201751176422, 27.58472315868180402 ) ) ;
#10375=EDGE_CURVE ( 'NONE', #2402, #43402, #8195, .T. ) ;
#10379=DIRECTION ( 'NONE',  ( -0.000000000000000000, -0.000000000000000000, 1.000000000000000000 ) ) ;
#10382=DIRECTION ( 'NONE',  ( 0.000000000000000000, 0.000000000000000000, 1.000000000000000000 ) ) ;
#10383=ORIENTED_EDGE ( 'NONE', *, *, #18660, .F. ) ;
#10397=EDGE_CURVE ( 'NONE', #17506, #32477, #35624, .T. ) ;
#10401=DIRECTION ( 'NONE',  ( 0.000000000000000000, -1.000000000000000000, 0.000000000000000000 ) ) ;
#10405=EDGE_LOOP ( 'NONE', ( #57561, #43931, #57378, #57229, #9254, #57778, #38972, #63901, #23057, #68473, #58540, #23737, #49244 ) ) ;
#10414=VECTOR ( 'NONE', #18922, 1000.000000000000114 ) ;
#10418=ADVANCED_FACE ( 'NONE', ( #14842 ), #24727, .T. ) ;
#10421=DIRECTION ( 'NONE',  ( -0.000000000000000000, -0.000000000000000000, -1.000000000000000000 ) ) ;
#10424=ORIENTED_EDGE ( 'NONE', *, *, #57887, .F. ) ;
#10425=ORIENTED_EDGE ( 'NONE', *, *, #26829, .T. ) ;
#10447=CARTESIAN_POINT ( 'NONE',  ( 13.24564585880038514, 63.65041531508843065, 41.38025477438755928 ) ) ;
#10450=ORIENTED_EDGE ( 'NONE', *, *, #809, .T. ) ;
#10451=CARTESIAN_POINT ( 'NONE',  ( 19.84876894326305319, 26.89441334579538534, 6.893342937333461151 ) ) ;
#10456=EDGE_CURVE ( 'NONE', #59826, #43402, #47525, .T. ) ;
#10457=DIRECTION ( 'NONE',  ( 0.9510565162951544194, -0.3090169943749446757, -2.199760087730564624E-16 ) ) ;
#10459=ADVANCED_FACE ( 'NONE', ( #47195 ), #63035, .T. ) ;
#10464=CIRCLE ( 'NONE', #28444, 65.36598343705435354 ) ;
#10480=EDGE_LOOP ( 'NONE', ( #46112, #53786, #23789, #45716 ) ) ;
#10483=EDGE_CURVE ( 'NONE', #10617, #24043, #9923, .T. ) ;
#10485=CARTESIAN_POINT ( 'NONE',  ( 73.57152302639893549, 14.62167909564606916, 43.58025477438756923 ) ) ;
#10493=AXIS2_PLACEMENT_3D ( 'NONE', #42460, #63917, #41777 ) ;
#10497=CARTESIAN_POINT ( 'NONE',  ( 0.000000000000000000, 0.000000000000000000, 40.00000000000003553 ) ) ;
#10499=AXIS2_PLACEMENT_3D ( 'NONE', #23362, #11736, #49709 ) ;
#10500=ORIENTED_EDGE ( 'NONE', *, *, #33854, .F. ) ;
#10502=VECTOR ( 'NONE', #59714, 1000.000000000000000 ) ;
#10508=LINE ( 'NONE', #52399, #5028 ) ;
#10509=ORIENTED_EDGE ( 'NONE', *, *, #29144, .T. ) ;
#10510=EDGE_LOOP ( 'NONE', ( #62783, #688, #10606, #21869, #28775, #32569, #337, #23067, #54642 ) ) ;
#10511=CARTESIAN_POINT ( 'NONE',  ( 0.000000000000000000, 0.000000000000000000, 0.000000000000000000 ) ) ;
#10517=LINE ( 'NONE', #37248, #2496 ) ;
#10518=DIRECTION ( 'NONE',  ( 2.312964634635743450E-16, -0.000000000000000000, 1.000000000000000000 ) ) ;
#10524=FACE_OUTER_BOUND ( 'NONE', #8302, .T. ) ;
#10529=CARTESIAN_POINT ( 'NONE',  ( -45.81425895439424067, 46.10914959592843587, 170.0000000000000000 ) ) ;
#10539=CARTESIAN_POINT ( 'NONE',  ( -59.89379335984725117, 45.06047301136835870, 41.38025477438755928 ) ) ;
#10540=VECTOR ( 'NONE', #7495, 1000.000000000000114 ) ;
#10553=VECTOR ( 'NONE', #17179, 1000.000000000000114 ) ;
#10555=VECTOR ( 'NONE', #48967, 1000.000000000000227 ) ;
#10557=VECTOR ( 'NONE', #20965, 1000.000000000000227 ) ;
#10560=ORIENTED_EDGE ( 'NONE', *, *, #21984, .T. ) ;
#10561=FACE_OUTER_BOUND ( 'NONE', #20899, .T. ) ;
#10573=EDGE_LOOP ( 'NONE', ( #40343, #21052, #8898, #1185 ) ) ;
#10581=DIRECTION ( 'NONE',  ( 0.3090169943749447312, 0.9510565162951544194, -7.147453794906795954E-17 ) ) ;
#10582=DIRECTION ( 'NONE',  ( 0.000000000000000000, 0.000000000000000000, 1.000000000000000000 ) ) ;
#10593=ADVANCED_FACE ( 'NONE', ( #68327 ), #41579, .T. ) ;
#10595=CARTESIAN_POINT ( 'NONE',  ( 0.000000000000000000, 0.000000000000000000, 0.000000000000000000 ) ) ;
#10596=VECTOR ( 'NONE', #3211, 1000.000000000000000 ) ;
#10605=VECTOR ( 'NONE', #31106, 1000.000000000000000 ) ;
#10606=ORIENTED_EDGE ( 'NONE', *, *, #41471, .F. ) ;
#10609=CARTESIAN_POINT ( 'NONE',  ( 24.86543818044729193, 29.17542891737278765, 13.32819397642334103 ) ) ;
#10615=CARTESIAN_POINT ( 'NONE',  ( -26.69131247781301752, 59.26697088776972322, 170.0000000000000000 ) ) ;
#10617=VERTEX_POINT ( 'NONE', #33107 ) ;
#10622=CARTESIAN_POINT ( 'NONE',  ( 0.000000000000000000, 0.000000000000000000, 0.000000000000000000 ) ) ;
#10626=ORIENTED_EDGE ( 'NONE', *, *, #27889, .F. ) ;
#10632=DIRECTION ( 'NONE',  ( -1.000000000000000000, 0.000000000000000000, 0.000000000000000000 ) ) ;
#10639=CARTESIAN_POINT ( 'NONE',  ( 74.62299871641508275, -5.461138973197948943, 41.38025477438755928 ) ) ;
#10645=EDGE_CURVE ( 'NONE', #44574, #10732, #747, .T. ) ;
#10649=AXIS2_PLACEMENT_3D ( 'NONE', #42127, #58299, #63588 ) ;
#10654=ORIENTED_EDGE ( 'NONE', *, *, #32356, .F. ) ;
#10656=DIRECTION ( 'NONE',  ( 1.000000000000000000, 0.000000000000000000, 0.000000000000000000 ) ) ;
#10666=DIRECTION ( 'NONE',  ( 0.9195277725514489076, 0.3930250316539278810, 5.102127870520022769E-18 ) ) ;
#10672=ORIENTED_EDGE ( 'NONE', *, *, #45101, .F. ) ;
#10673=ORIENTED_EDGE ( 'NONE', *, *, #22732, .F. ) ;
#10674=ORIENTED_EDGE ( 'NONE', *, *, #39970, .T. ) ;
#10676=CARTESIAN_POINT ( 'NONE',  ( 28.03046753626767895, -26.14935100755965891, 13.32819397642332682 ) ) ;
#10681=DIRECTION ( 'NONE',  ( -0.9009688679024155933, -0.4338837391175656699, 0.000000000000000000 ) ) ;
#10682=DIRECTION ( 'NONE',  ( -0.000000000000000000, -0.000000000000000000, -1.000000000000000000 ) ) ;
#10683=EDGE_CURVE ( 'NONE', #47961, #46223, #10955, .T. ) ;
#10685=AXIS2_PLACEMENT_3D ( 'NONE', #68390, #57146, #13874 ) ;
#10690=VECTOR ( 'NONE', #41576, 1000.000000000000000 ) ;
#10696=DIRECTION ( 'NONE',  ( 0.5508969814521065267, -0.8345732537212999791, 0.000000000000000000 ) ) ;
#10698=LINE ( 'NONE', #4402, #50956 ) ;
#10704=EDGE_CURVE ( 'NONE', #43978, #16942, #54922, .T. ) ;
#10707=APPLICATION_CONTEXT ( 'automotive_design' ) ;
#10715=CARTESIAN_POINT ( 'NONE',  ( -84.49322488516129681, 0.000000000000000000, 43.58025477438756212 ) ) ;
#10722=B_SPLINE_CURVE_WITH_KNOTS ( 'NONE', 3,
 ( #36738, #20897, #42352, #26862, #48287, #14918 ),
 .UNSPECIFIED., .F., .F.,
 ( 4, 2, 4 ),
 ( 1.095770181106172926E-06, 0.03239442681617710901, 0.06478775786217311206 ),
 .UNSPECIFIED. ) ;
#10732=VERTEX_POINT ( 'NONE', #43989 ) ;
#10735=EDGE_CURVE ( 'NONE', #56044, #67138, #60533, .T. ) ;
#10738=ORIENTED_EDGE ( 'NONE', *, *, #6259, .T. ) ;
#10740=ORIENTED_EDGE ( 'NONE', *, *, #14837, .T. ) ;
#10747=LINE ( 'NONE', #4444, #22976 ) ;
#10763=CARTESIAN_POINT ( 'NONE',  ( 39.77028211725815510, -51.87520073220884598, 6.377659838150125143E-18 ) ) ;
#10768=DIRECTION ( 'NONE',  ( -0.9959742939952397345, 0.08963930890342655666, 0.000000000000000000 ) ) ;
#10769=EDGE_CURVE ( 'NONE', #48528, #2304, #13993, .T. ) ;
#10785=ORIENTED_EDGE ( 'NONE', *, *, #11877, .F. ) ;
#10789=CARTESIAN_POINT ( 'NONE',  ( -45.99287130332146489, 23.53639479597885398, 26.66469104408688295 ) ) ;
#10806=CARTESIAN_POINT ( 'NONE',  ( 70.65683382808195745, 25.18281821780106355, 43.58025477438756212 ) ) ;
#10812=LINE ( 'NONE', #33676, #42337 ) ;
#10815=ORIENTED_EDGE ( 'NONE', *, *, #62148, .F. ) ;
#10817=CARTESIAN_POINT ( 'NONE',  ( -58.00979178563853367, 29.32343869649098878, 40.00000000000003553 ) ) ;
#10821=VERTEX_POINT ( 'NONE', #52988 ) ;
#10822=DIRECTION ( 'NONE',  ( -0.9839295885986295565, -0.1785568947986370392, 0.000000000000000000 ) ) ;
#10834=ORIENTED_EDGE ( 'NONE', *, *, #63454, .T. ) ;
#10843=VERTEX_POINT ( 'NONE', #47712 ) ;
#10851=EDGE_CURVE ( 'NONE', #22589, #20231, #41764, .T. ) ;
#10853=CARTESIAN_POINT ( 'NONE',  ( 7.484861546145933353, -64.56761454192826477, 170.0000000000000000 ) ) ;
#10862=PLANE ( 'NONE',  #54875 ) ;
#10863=DIRECTION ( 'NONE',  ( 1.000000000000000000, 0.000000000000000000, 0.000000000000000000 ) ) ;
#10867=DIRECTION ( 'NONE',  ( -1.000000000000000000, 0.000000000000000000, 2.135044278125301096E-16 ) ) ;
#10869=DIRECTION ( 'NONE',  ( 0.3930250316539278255, -0.9195277725514487965, -9.090529987421286498E-17 ) ) ;
#10870=EDGE_LOOP ( 'NONE', ( #24126, #32764, #62167, #10916, #13445, #62557, #68941, #47675, #25896 ) ) ;
#10871=DIRECTION ( 'NONE',  ( -1.792759282944425749E-18, -4.776790026843733425E-18, -1.000000000000000000 ) ) ;
#10874=DIRECTION ( 'NONE',  ( 0.000000000000000000, 0.000000000000000000, 1.000000000000000000 ) ) ;
#10884=DIRECTION ( 'NONE',  ( 0.1342332658176522420, 0.9909497617679351444, 0.000000000000000000 ) ) ;
#10890=DIRECTION ( 'NONE',  ( 1.000000000000000000, 0.000000000000000000, 0.000000000000000000 ) ) ;
#10898=FACE_OUTER_BOUND ( 'NONE', #29450, .T. ) ;
#10900=CARTESIAN_POINT ( 'NONE',  ( -57.97933172774389732, 6.473286776202990644, 27.58472315868180047 ) ) ;
#10901=AXIS2_PLACEMENT_3D ( 'NONE', #35899, #8830, #51392 ) ;
#10902=LINE ( 'NONE', #48513, #42587 ) ;
#10916=ORIENTED_EDGE ( 'NONE', *, *, #22390, .T. ) ;
#10918=ORIENTED_EDGE ( 'NONE', *, *, #63068, .T. ) ;
#10920=PLANE ( 'NONE',  #14833 ) ;
#10933=DIRECTION ( 'NONE',  ( -0.000000000000000000, -0.000000000000000000, -1.000000000000000000 ) ) ;
#10934=FACE_OUTER_BOUND ( 'NONE', #53819, .T. ) ;
#10943=DIRECTION ( 'NONE',  ( 1.000000000000000000, 0.000000000000000000, -0.000000000000000000 ) ) ;
#10947=CARTESIAN_POINT ( 'NONE',  ( 0.000000000000000000, 0.000000000000000000, 0.000000000000000000 ) ) ;
#10952=DIRECTION ( 'NONE',  ( 0.9362348706397417564, -0.3513748240813305279, 0.000000000000000000 ) ) ;
#10955=CIRCLE ( 'NONE', #27833, 65.36598343705435354 ) ;
#10966=DIRECTION ( 'NONE',  ( -0.000000000000000000, -0.000000000000000000, -1.000000000000000000 ) ) ;
#10985=CARTESIAN_POINT ( 'NONE',  ( -50.92620509423088038, 55.07344309828769724, 170.0000000000000000 ) ) ;
#10993=DIRECTION ( 'NONE',  ( -0.6910626489868580968, -0.7227948638273978821, 0.000000000000000000 ) ) ;
#10994=DIRECTION ( 'NONE',  ( 1.000000000000000000, 7.993605777301127091E-15, 0.000000000000000000 ) ) ;
#10997=EDGE_CURVE ( 'NONE', #27271, #21605, #49442, .T. ) ;
#10998=EDGE_LOOP ( 'NONE', ( #64553, #57549, #21744, #31268 ) ) ;
#11003=VERTEX_POINT ( 'NONE', #928 ) ;
#11014=ORIENTED_EDGE ( 'NONE', *, *, #8349, .T. ) ;
#11015=EDGE_CURVE ( 'NONE', #32122, #29231, #579, .T. ) ;
#11020=LINE ( 'NONE', #25922, #41851 ) ;
#11036=ORIENTED_EDGE ( 'NONE', *, *, #6430, .T. ) ;
#11044=ADVANCED_FACE ( 'NONE', ( #49090 ), #6197, .T. ) ;
#11045=ADVANCED_FACE ( 'NONE', ( #16406 ), #3153, .T. ) ;
#11050=ORIENTED_EDGE ( 'NONE', *, *, #66030, .F. ) ;
#11051=ORIENTED_EDGE ( 'NONE', *, *, #39858, .T. ) ;
#11078=B_SPLINE_CURVE_WITH_KNOTS ( 'NONE', 3,
 ( #34446, #23873, #18241, #39013, #29837, #22825 ),
 .UNSPECIFIED., .F., .F.,
 ( 4, 2, 4 ),
 ( 0.03218941534092207429, 0.06469837595388627793, 0.09720733656685046076 ),
 .UNSPECIFIED. ) ;
#11079=DIRECTION ( 'NONE',  ( 0.4738686624730094610, -0.8805955318567322276, 0.000000000000000000 ) ) ;
#11093=VECTOR ( 'NONE', #11949, 999.9999999999998863 ) ;
#11095=DIRECTION ( 'NONE',  ( 0.000000000000000000, 0.000000000000000000, 1.000000000000000000 ) ) ;
#11096=EDGE_CURVE ( 'NONE', #3858, #51807, #16747, .T. ) ;
#11097=ORIENTED_EDGE ( 'NONE', *, *, #14685, .T. ) ;
#11099=ORIENTED_EDGE ( 'NONE', *, *, #68923, .T. ) ;
#11101=FACE_OUTER_BOUND ( 'NONE', #15793, .T. ) ;
#11111=FACE_OUTER_BOUND ( 'NONE', #61284, .T. ) ;
#11119=ORIENTED_EDGE ( 'NONE', *, *, #16639, .F. ) ;
#11123=DIRECTION ( 'NONE',  ( -0.000000000000000000, -0.000000000000000000, 1.000000000000000000 ) ) ;
#11125=EDGE_CURVE ( 'NONE', #45414, #51882, #31112, .T. ) ;
#11134=VERTEX_POINT ( 'NONE', #45572 ) ;
#11140=VECTOR ( 'NONE', #51084, 1000.000000000000000 ) ;
#11147=ORIENTED_EDGE ( 'NONE', *, *, #25287, .F. ) ;
#11149=DIRECTION ( 'NONE',  ( -0.000000000000000000, -0.000000000000000000, -1.000000000000000000 ) ) ;
#11155=ORIENTED_EDGE ( 'NONE', *, *, #61473, .F. ) ;
#11165=CARTESIAN_POINT ( 'NONE',  ( -10.96274578891745755, -22.46815979931523799, 0.000000000000000000 ) ) ;
#11167=DIRECTION ( 'NONE',  ( -0.000000000000000000, -0.000000000000000000, -1.000000000000000000 ) ) ;
#11168=ADVANCED_FACE ( 'NONE', ( #8647, #7945 ), #29397, .T. ) ;
#11174=VECTOR ( 'NONE', #49172, 1000.000000000000114 ) ;
#11181=CIRCLE ( 'NONE', #47144, 65.36598343705435354 ) ;
#11190=FACE_OUTER_BOUND ( 'NONE', #28622, .T. ) ;
#11191=DIRECTION ( 'NONE',  ( -0.000000000000000000, -0.000000000000000000, -1.000000000000000000 ) ) ;
#11199=EDGE_CURVE ( 'NONE', #43402, #64171, #13568, .T. ) ;
#11204=EDGE_CURVE ( 'NONE', #28933, #37212, #6545, .T. ) ;
#11207=DIRECTION ( 'NONE',  ( -4.463998536185269061E-17, -2.459865942543005358E-16, 1.000000000000000000 ) ) ;
#11211=DIRECTION ( 'NONE',  ( 0.000000000000000000, 0.000000000000000000, 1.000000000000000000 ) ) ;
#11225=EDGE_LOOP ( 'NONE', ( #35621, #9387, #63231, #16757 ) ) ;
#11226=ORIENTED_EDGE ( 'NONE', *, *, #50364, .T. ) ;
#11244=FACE_BOUND ( 'NONE', #14499, .T. ) ;
#11247=ORIENTED_EDGE ( 'NONE', *, *, #39470, .T. ) ;
#11250=DIRECTION ( 'NONE',  ( 1.000000000000000000, 0.000000000000000000, -0.000000000000000000 ) ) ;
#11252=DIRECTION ( 'NONE',  ( 0.3090169943749582759, -0.9510565162951500895, 0.000000000000000000 ) ) ;
#11254=AXIS2_PLACEMENT_3D ( 'NONE', #49886, #1710, #66096 ) ;
#11256=EDGE_CURVE ( 'NONE', #35316, #30444, #62095, .T. ) ;
#11259=CARTESIAN_POINT ( 'NONE',  ( 18.89356949897823768, 62.19351277735707839, 73.58025477438755502 ) ) ;
#11268=VERTEX_POINT ( 'NONE', #35725 ) ;
#11276=ORIENTED_EDGE ( 'NONE', *, *, #30052, .F. ) ;
#11278=DIRECTION ( 'NONE',  ( 0.000000000000000000, 0.000000000000000000, 1.000000000000000000 ) ) ;
#11282=FACE_OUTER_BOUND ( 'NONE', #5199, .T. ) ;
#11285=DIRECTION ( 'NONE',  ( -1.000000000000000000, 0.000000000000000000, 0.000000000000000000 ) ) ;
#11288=CARTESIAN_POINT ( 'NONE',  ( 0.000000000000000000, 0.000000000000000000, 41.38025477438755928 ) ) ;
#11289=CARTESIAN_POINT ( 'NONE',  ( 0.000000000000000000, 0.000000000000000000, 40.00000000000003553 ) ) ;
#11294=ORIENTED_EDGE ( 'NONE', *, *, #5550, .F. ) ;
#11295=CARTESIAN_POINT ( 'NONE',  ( 44.01696072966019102, -47.84694004974149095, 3.061616997868437868E-16 ) ) ;
#11304=CIRCLE ( 'NONE', #50635, 65.36598343705435354 ) ;
#11306=DIRECTION ( 'NONE',  ( 1.000000000000000000, 0.000000000000000000, 0.000000000000000000 ) ) ;
#11307=ORIENTED_EDGE ( 'NONE', *, *, #47001, .T. ) ;
#11308=ORIENTED_EDGE ( 'NONE', *, *, #63943, .F. ) ;
#11311=CARTESIAN_POINT ( 'NONE',  ( -59.49248125703533674, -30.03746431348988111, 34.48241823988799837 ) ) ;
#11324=CARTESIAN_POINT ( 'NONE',  ( 45.78444578631987127, 59.41672343742573759, 170.0000000000000000 ) ) ;
#11326=CARTESIAN_POINT ( 'NONE',  ( -45.81425895439360829, -46.10914959592906825, 170.0000000000000000 ) ) ;
#11327=EDGE_CURVE ( 'NONE', #31093, #11589, #48655, .T. ) ;
#11334=LINE ( 'NONE', #54234, #9663 ) ;
#11335=DIRECTION ( 'NONE',  ( -0.000000000000000000, -0.000000000000000000, -1.000000000000000000 ) ) ;
#11338=DIRECTION ( 'NONE',  ( -0.000000000000000000, -0.000000000000000000, -1.000000000000000000 ) ) ;
#11342=DIRECTION ( 'NONE',  ( -0.8090169943749506709, 0.5877852522924686962, 0.000000000000000000 ) ) ;
#11351=FACE_OUTER_BOUND ( 'NONE', #54085, .T. ) ;
#11353=LINE ( 'NONE', #47013, #68761 ) ;
#11373=DIRECTION ( 'NONE',  ( -0.000000000000000000, -0.000000000000000000, -1.000000000000000000 ) ) ;
#11374=CARTESIAN_POINT ( 'NONE',  ( 22.18075376363910323, 11.79626863379964696, 0.000000000000000000 ) ) ;
#11376=CARTESIAN_POINT ( 'NONE',  ( -23.73638277007033182, -7.847555861075553807, 0.000000000000000000 ) ) ;
#11400=CARTESIAN_POINT ( 'NONE',  ( 0.1285234777257801275, -24.99966963213046611, 0.000000000000000000 ) ) ;
#11402=DIRECTION ( 'NONE',  ( -0.000000000000000000, -0.000000000000000000, -1.000000000000000000 ) ) ;
#11414=CYLINDRICAL_SURFACE ( 'NONE', #54777, 65.36598343705435354 ) ;
#11417=VERTEX_POINT ( 'NONE', #63753 ) ;
#11420=EDGE_LOOP ( 'NONE', ( #22996, #29787, #1762, #26593 ) ) ;
#11421=EDGE_LOOP ( 'NONE', ( #7711, #36469, #60361, #60525, #30083, #55207, #49804, #8486, #2813 ) ) ;
#11423=CARTESIAN_POINT ( 'NONE',  ( -7.486743542469090684, -64.58150799671139453, 170.0000000000000000 ) ) ;
#11424=ADVANCED_FACE ( 'NONE', ( #58125 ), #68002, .T. ) ;
#11439=VERTEX_POINT ( 'NONE', #9247 ) ;
#11443=AXIS2_PLACEMENT_3D ( 'NONE', #36901, #58340, #11527 ) ;
#11446=DIRECTION ( 'NONE',  ( 1.000000000000000000, 0.000000000000000000, -1.156482317317871232E-16 ) ) ;
#11448=VECTOR ( 'NONE', #21763, 1000.000000000000000 ) ;
#11464=EDGE_CURVE ( 'NONE', #17465, #51505, #59157, .T. ) ;
#11466=CARTESIAN_POINT ( 'NONE',  ( 11.29825944729730303, 74.09495289493001735, 41.38025477438755928 ) ) ;
#11468=PLANE ( 'NONE',  #56521 ) ;
#11481=CARTESIAN_POINT ( 'NONE',  ( 45.74764628539747235, 59.37057832282332726, 41.38025477438755928 ) ) ;
#11488=LINE ( 'NONE', #249, #38980 ) ;
#11494=DIRECTION ( 'NONE',  ( 0.000000000000000000, 0.000000000000000000, 1.000000000000000000 ) ) ;
#11498=ORIENTED_EDGE ( 'NONE', *, *, #40421, .F. ) ;
#11518=LINE ( 'NONE', #54072, #31710 ) ;
#11523=DIRECTION ( 'NONE',  ( -0.000000000000000000, -0.000000000000000000, -1.000000000000000000 ) ) ;
#11527=DIRECTION ( 'NONE',  ( -1.000000000000000000, 0.000000000000000000, 0.000000000000000000 ) ) ;
#11529=CARTESIAN_POINT ( 'NONE',  ( 36.61292551086699376, -65.40035471292219427, 41.38025477438755928 ) ) ;
#11530=CARTESIAN_POINT ( 'NONE',  ( 9.962235950564874543, 64.23203137738424573, 40.00000000000003553 ) ) ;
#11536=AXIS2_PLACEMENT_3D ( 'NONE', #1455, #6728, #38388 ) ;
#11538=FACE_OUTER_BOUND ( 'NONE', #5389, .T. ) ;
#11552=PLANE ( 'NONE',  #54314 ) ;
#11560=DIRECTION ( 'NONE',  ( -0.000000000000000000, -0.000000000000000000, -1.000000000000000000 ) ) ;
#11564=ORIENTED_EDGE ( 'NONE', *, *, #49135, .T. ) ;
#11566=CARTESIAN_POINT ( 'NONE',  ( 23.81581464765709200, 7.603089679099848119, 0.000000000000000000 ) ) ;
#11568=EDGE_CURVE ( 'NONE', #28173, #29753, #58795, .T. ) ;
#11576=ADVANCED_FACE ( 'NONE', ( #44005 ), #60194, .T. ) ;
#11589=VERTEX_POINT ( 'NONE', #66891 ) ;
#11590=ORIENTED_EDGE ( 'NONE', *, *, #19522, .T. ) ;
#11591=PLANE ( 'NONE',  #23310 ) ;
#11596=EDGE_CURVE ( 'NONE', #29753, #66023, #24319, .T. ) ;
#11598=CONICAL_SURFACE ( 'NONE', #53169, 63.58578643762691485, 0.7853981633974497223 ) ;
#11601=AXIS2_PLACEMENT_3D ( 'NONE', #57347, #20390, #20743 ) ;
#11604=AXIS2_PLACEMENT_3D ( 'NONE', #1655, #7287, #59681 ) ;
#11606=ORIENTED_EDGE ( 'NONE', *, *, #45679, .T. ) ;
#11607=FACE_OUTER_BOUND ( 'NONE', #27750, .T. ) ;
#11617=DIRECTION ( 'NONE',  ( 0.000000000000000000, 0.000000000000000000, 1.000000000000000000 ) ) ;
#11622=DIRECTION ( 'NONE',  ( -0.000000000000000000, -0.000000000000000000, -1.000000000000000000 ) ) ;
#11623=APPLICATION_CONTEXT ( 'automotive_design' ) ;
#11635=CARTESIAN_POINT ( 'NONE',  ( -55.15976438495108169, -34.41253982194112382, 43.58025477438756923 ) ) ;
#11638=DIRECTION ( 'NONE',  ( 0.000000000000000000, 0.000000000000000000, 1.000000000000000000 ) ) ;
#11645=ORIENTED_EDGE ( 'NONE', *, *, #2017, .T. ) ;
#11660=EDGE_CURVE ( 'NONE', #8487, #47971, #58067, .T. ) ;
#11663=DIRECTION ( 'NONE',  ( -0.000000000000000000, 1.000000000000000000, -0.000000000000000000 ) ) ;
#11665=AXIS2_PLACEMENT_3D ( 'NONE', #59698, #43868, #61112 ) ;
#11667=ADVANCED_FACE ( 'NONE', ( #23957 ), #34869, .T. ) ;
#11669=VECTOR ( 'NONE', #50266, 1000.000000000000000 ) ;
#11680=B_SPLINE_CURVE_WITH_KNOTS ( 'NONE', 3,
 ( #28365, #55803, #49812, #50523, #12543, #51221 ),
 .UNSPECIFIED., .F., .F.,
 ( 4, 2, 4 ),
 ( 0.03218932648122787427, 0.06469831129177408546, 0.09720729610232028972 ),
 .UNSPECIFIED. ) ;
#11687=CARTESIAN_POINT ( 'NONE',  ( 64.16679220703380793, -10.37413986118096254, 40.00000000000003553 ) ) ;
#11692=EDGE_LOOP ( 'NONE', ( #15774, #5253, #25792, #8364 ) ) ;
#11699=AXIS2_PLACEMENT_3D ( 'NONE', #55002, #28272, #20157 ) ;
#11716=ORIENTED_EDGE ( 'NONE', *, *, #46142, .F. ) ;
#11718=VERTEX_POINT ( 'NONE', #29573 ) ;
#11730=EDGE_CURVE ( 'NONE', #14469, #33967, #20016, .T. ) ;
#11736=DIRECTION ( 'NONE',  ( 0.000000000000000000, 0.000000000000000000, 1.000000000000000000 ) ) ;
#11737=CARTESIAN_POINT ( 'NONE',  ( -84.49322488516129681, 0.000000000000000000, 43.58025477438756212 ) ) ;
#11738=DIRECTION ( 'NONE',  ( -0.000000000000000000, -0.000000000000000000, -1.000000000000000000 ) ) ;
#11740=VERTEX_POINT ( 'NONE', #28897 ) ;
#11748=ADVANCED_FACE ( 'NONE', ( #17641 ), #61249, .F. ) ;
#11749=EDGE_CURVE ( 'NONE', #28072, #38689, #51039, .T. ) ;
#11763=DIRECTION ( 'NONE',  ( 0.000000000000000000, 0.000000000000000000, 1.000000000000000000 ) ) ;
#11774=ORIENTED_EDGE ( 'NONE', *, *, #55986, .T. ) ;
#11777=CARTESIAN_POINT ( 'NONE',  ( 24.39800339187844003, 60.26242556095705538, 170.0000000000000000 ) ) ;
#11802=VERTEX_POINT ( 'NONE', #68925 ) ;
#11805=CARTESIAN_POINT ( 'NONE',  ( 64.98797965777978902, 1.250000000000011990, 40.00000000000003553 ) ) ;
#11807=CONICAL_SURFACE ( 'NONE', #20800, 74.95140232871122521, 0.8777644062502172329 ) ;
#11815=CARTESIAN_POINT ( 'NONE',  ( -26.28838098083469887, -20.64471174685882815, 6.893342936425401746 ) ) ;
#11818=ORIENTED_EDGE ( 'NONE', *, *, #17427, .F. ) ;
#11822=DIRECTION ( 'NONE',  ( 0.000000000000000000, 0.000000000000000000, 1.000000000000000000 ) ) ;
#11823=DIRECTION ( 'NONE',  ( -0.000000000000000000, -0.000000000000000000, -1.000000000000000000 ) ) ;
#11825=DIRECTION ( 'NONE',  ( -1.000000000000000000, 0.000000000000000000, 0.000000000000000000 ) ) ;
#11832=ORIENTED_EDGE ( 'NONE', *, *, #9610, .T. ) ;
#11833=CARTESIAN_POINT ( 'NONE',  ( -65.36598343705435354, 0.000000000000000000, 41.38025477438755928 ) ) ;
#11839=DIRECTION ( 'NONE',  ( -1.000000000000000000, 0.000000000000000000, 0.000000000000000000 ) ) ;
#11840=DIRECTION ( 'NONE',  ( -0.3930250316539278255, 0.9195277725514487965, 0.000000000000000000 ) ) ;
#11842=PLANE ( 'NONE',  #10197 ) ;
#11854=LINE ( 'NONE', #60399, #36336 ) ;
#11860=AXIS2_PLACEMENT_3D ( 'NONE', #22780, #28766, #2039 ) ;
#11866=AXIS2_PLACEMENT_3D ( 'NONE', #32228, #27277, #16725 ) ;
#11869=FACE_OUTER_BOUND ( 'NONE', #1889, .T. ) ;
#11872=DIRECTION ( 'NONE',  ( -0.000000000000000000, -0.000000000000000000, -1.000000000000000000 ) ) ;
#11874=DIRECTION ( 'NONE',  ( 0.000000000000000000, 0.000000000000000000, 1.000000000000000000 ) ) ;
#11877=EDGE_CURVE ( 'NONE', #25430, #13094, #43478, .T. ) ;
#11885=LINE ( 'NONE', #44596, #56651 ) ;
#11891=CIRCLE ( 'NONE', #13079, 65.36598343705435354 ) ;
#11904=CIRCLE ( 'NONE', #31997, 24.99999999999985434 ) ;
#11905=CARTESIAN_POINT ( 'NONE',  ( -84.49322488516129681, 0.000000000000000000, 43.58025477438756212 ) ) ;
#11911=AXIS2_PLACEMENT_3D ( 'NONE', #57071, #29989, #14155 ) ;
#11912=DIRECTION ( 'NONE',  ( 0.9362348706397369824, 0.3513748240813435175, 0.000000000000000000 ) ) ;
#11915=AXIS2_PLACEMENT_3D ( 'NONE', #58362, #5586, #64687 ) ;
#11919=ADVANCED_FACE ( 'NONE', ( #25701 ), #68593, .T. ) ;
#11933=LINE ( 'NONE', #42641, #20697 ) ;
#11934=ORIENTED_EDGE ( 'NONE', *, *, #42075, .F. ) ;
#11941=ORIENTED_EDGE ( 'NONE', *, *, #45340, .F. ) ;
#11942=CARTESIAN_POINT ( 'NONE',  ( -65.36598343705435354, 0.000000000000000000, 41.38025477438755928 ) ) ;
#11949=DIRECTION ( 'NONE',  ( -0.4738686624729966379, -0.8805955318567391110, 0.000000000000000000 ) ) ;
#11958=AXIS2_PLACEMENT_3D ( 'NONE', #13416, #34879, #56317 ) ;
#11961=DIRECTION ( 'NONE',  ( 0.9989930665413143673, 0.04486483035051862939, -2.310635633156372120E-16 ) ) ;
#11962=CIRCLE ( 'NONE', #36677, 65.36598343705435354 ) ;
#11970=EDGE_CURVE ( 'NONE', #34424, #65974, #14095, .T. ) ;
#11976=DIRECTION ( 'NONE',  ( -0.6910626489868685329, 0.7227948638273878901, 0.000000000000000000 ) ) ;
#11984=FACE_BOUND ( 'NONE', #51693, .T. ) ;
#11996=DIRECTION ( 'NONE',  ( 0.000000000000000000, 0.000000000000000000, 1.000000000000000000 ) ) ;
#11997=DIRECTION ( 'NONE',  ( 0.7530714660036099684, 0.6579387259397136978, 0.000000000000000000 ) ) ;
#12008=CARTESIAN_POINT ( 'NONE',  ( -14.86595946517991429, -20.25193917588099524, 0.000000000000000000 ) ) ;
#12010=VECTOR ( 'NONE', #48767, 1000.000000000000000 ) ;
#12012=DIRECTION ( 'NONE',  ( -0.8805955318567391110, 0.4738686624729966379, 2.500042656554809847E-16 ) ) ;
#12015=EDGE_CURVE ( 'NONE', #25148, #2042, #63692, .T. ) ;
#12026=CARTESIAN_POINT ( 'NONE',  ( -22.06416059020174103, -12.01293505575318044, 3.061616997868437868E-16 ) ) ;
#12027=AXIS2_PLACEMENT_3D ( 'NONE', #22798, #17512, #48807 ) ;
#12050=CARTESIAN_POINT ( 'NONE',  ( 0.000000000000000000, 0.000000000000000000, 0.000000000000000000 ) ) ;
#12053=ORIENTED_EDGE ( 'NONE', *, *, #58139, .T. ) ;
#12061=ORIENTED_EDGE ( 'NONE', *, *, #57323, .T. ) ;
#12069=EDGE_CURVE ( 'NONE', #41387, #22570, #36934, .T. ) ;
#12079=FACE_OUTER_BOUND ( 'NONE', #60763, .T. ) ;
#12080=ORIENTED_EDGE ( 'NONE', *, *, #37816, .F. ) ;
#12081=VERTEX_POINT ( 'NONE', #17185 ) ;
#12089=CARTESIAN_POINT ( 'NONE',  ( -4.164416015345870470, 64.86646004871185767, 73.58025477438755502 ) ) ;
#12091=CARTESIAN_POINT ( 'NONE',  ( 6.590627171038061505, 57.96611128877285779, 27.58472369369409094 ) ) ;
#12093=DIRECTION ( 'NONE',  ( 0.9959742939952397345, -0.08963930890342655666, 0.000000000000000000 ) ) ;
#12104=EDGE_CURVE ( 'NONE', #4696, #34928, #66806, .T. ) ;
#12108=VERTEX_POINT ( 'NONE', #61509 ) ;
#12111=DIRECTION ( 'NONE',  ( -0.000000000000000000, -0.000000000000000000, -1.000000000000000000 ) ) ;
#12117=DIRECTION ( 'NONE',  ( -1.000000000000000000, 0.000000000000000000, 0.000000000000000000 ) ) ;
#12118=CARTESIAN_POINT ( 'NONE',  ( -36.84489839129339828, 53.54860840895182150, 40.00000000000003553 ) ) ;
#12119=ORIENTED_EDGE ( 'NONE', *, *, #35751, .T. ) ;
#12120=CIRCLE ( 'NONE', #63789, 24.99999999999985434 ) ;
#12124=DIRECTION ( 'NONE',  ( 0.000000000000000000, 0.000000000000000000, 1.000000000000000000 ) ) ;
#12129=VECTOR ( 'NONE', #38920, 1000.000000000000000 ) ;
#12130=ORIENTED_EDGE ( 'NONE', *, *, #9343, .F. ) ;
#12134=CARTESIAN_POINT ( 'NONE',  ( 0.000000000000000000, 0.000000000000000000, 0.000000000000000000 ) ) ;
#12135=CARTESIAN_POINT ( 'NONE',  ( -19.56458807131854627, 15.75959024859389324, 0.000000000000000000 ) ) ;
#12138=ORIENTED_EDGE ( 'NONE', *, *, #17286, .T. ) ;
#12150=CARTESIAN_POINT ( 'NONE',  ( -72.62976060914745347, 18.74780984163036024, 170.0000000000000000 ) ) ;
#12155=EDGE_CURVE ( 'NONE', #9288, #3940, #6645, .T. ) ;
#12161=VECTOR ( 'NONE', #62752, 1000.000000000000000 ) ;
#12167=AXIS2_PLACEMENT_3D ( 'NONE', #7759, #65812, #33789 ) ;
#12169=LINE ( 'NONE', #17796, #15529 ) ;
#12177=DIRECTION ( 'NONE',  ( 1.000000000000000000, 0.000000000000000000, 0.000000000000000000 ) ) ;
#12178=DIRECTION ( 'NONE',  ( 0.000000000000000000, 0.000000000000000000, -1.000000000000000000 ) ) ;
#12186=DIRECTION ( 'NONE',  ( 1.000000000000000000, 0.000000000000000000, -0.000000000000000000 ) ) ;
#12191=EDGE_LOOP ( 'NONE', ( #9539, #10424, #53606, #20953 ) ) ;
#12198=LINE ( 'NONE', #49457, #14178 ) ;
#12199=FACE_OUTER_BOUND ( 'NONE', #3317, .T. ) ;
#12205=LINE ( 'NONE', #951, #39649 ) ;
#12212=ORIENTED_EDGE ( 'NONE', *, *, #20251, .F. ) ;
#12218=VECTOR ( 'NONE', #7687, 1000.000000000000227 ) ;
#12221=DIRECTION ( 'NONE',  ( -1.000000000000000000, 0.000000000000000000, 0.000000000000000000 ) ) ;
#12225=EDGE_CURVE ( 'NONE', #49213, #30161, #52668, .T. ) ;
#12256=ORIENTED_EDGE ( 'NONE', *, *, #9008, .T. ) ;
#12258=ORIENTED_EDGE ( 'NONE', *, *, #31652, .F. ) ;
#12260=CARTESIAN_POINT ( 'NONE',  ( 45.78444578632068840, -59.41672343742509810, 43.58025477438756212 ) ) ;
#12265=CARTESIAN_POINT ( 'NONE',  ( 8.828807734113986783, 74.48902371486718721, 43.58025477438756923 ) ) ;
#12279=PLANE ( 'NONE',  #68177 ) ;
#12291=FACE_OUTER_BOUND ( 'NONE', #11225, .T. ) ;
#12292=B_SPLINE_CURVE_WITH_KNOTS ( 'NONE', 3,
 ( #10539, #9874, #30985, #52082, #4582, #53444 ),
 .UNSPECIFIED., .F., .F.,
 ( 4, 2, 4 ),
 ( 1.095770181107970753E-06, 0.03239442681617710901, 0.06478775786217311206 ),
 .UNSPECIFIED. ) ;
#12307=CARTESIAN_POINT ( 'NONE',  ( 0.000000000000000000, 0.000000000000000000, 40.00000000000003553 ) ) ;
#12309=AXIS2_PLACEMENT_3D ( 'NONE', #47606, #10666, #43369 ) ;
#12316=CARTESIAN_POINT ( 'NONE',  ( 10.18313842235669320, -65.86279891076495119, 34.48241823979989107 ) ) ;
#12323=VERTEX_POINT ( 'NONE', #2951 ) ;
#12328=ORIENTED_EDGE ( 'NONE', *, *, #37731, .F. ) ;
#12329=PLANE ( 'NONE',  #6444 ) ;
#12333=DIRECTION ( 'NONE',  ( -0.9959742939952397345, 0.08963930890342655666, 0.000000000000000000 ) ) ;
#12335=PLANE ( 'NONE',  #24693 ) ;
#12338=ORIENTED_EDGE ( 'NONE', *, *, #2017, .F. ) ;
#12344=CARTESIAN_POINT ( 'NONE',  ( 17.98081503251148661, 17.36923402935782690, 0.000000000000000000 ) ) ;
#12348=CARTESIAN_POINT ( 'NONE',  ( 39.71871838048090808, 33.04133019307971608, 26.66469104408690782 ) ) ;
#12349=CARTESIAN_POINT ( 'NONE',  ( -42.32797523529043104, -61.85511477251480983, 41.38025477438755928 ) ) ;
#12350=DIRECTION ( 'NONE',  ( -0.000000000000000000, -0.000000000000000000, -1.000000000000000000 ) ) ;
#12352=CARTESIAN_POINT ( 'NONE',  ( 58.32618493680805472, -1.250000000000021982, 27.58472315868180402 ) ) ;
#12355=ORIENTED_EDGE ( 'NONE', *, *, #28194, .T. ) ;
#12365=EDGE_CURVE ( 'NONE', #11740, #53513, #1919, .T. ) ;
#12367=CARTESIAN_POINT ( 'NONE',  ( 21.98745393275290994, -71.71550996510497100, 170.0000000000000000 ) ) ;
#12371=CARTESIAN_POINT ( 'NONE',  ( -50.92620509423012720, -55.07344309828840068, 170.0000000000000000 ) ) ;
#12378=ORIENTED_EDGE ( 'NONE', *, *, #52356, .F. ) ;
#12382=CARTESIAN_POINT ( 'NONE',  ( 74.95140232871122521, 0.000000000000000000, 41.38025477438755928 ) ) ;
#12386=EDGE_CURVE ( 'NONE', #54975, #36640, #28636, .T. ) ;
#12395=EDGE_CURVE ( 'NONE', #28933, #35756, #38098, .T. ) ;
#12397=VECTOR ( 'NONE', #34260, 1000.000000000000000 ) ;
#12399=ORIENTED_EDGE ( 'NONE', *, *, #8502, .F. ) ;
#12400=CARTESIAN_POINT ( 'NONE',  ( -64.97888516016278970, 7.103257987405393159, 6.377659838150127454E-18 ) ) ;
#12402=ORIENTED_EDGE ( 'NONE', *, *, #37306, .T. ) ;
#12406=CARTESIAN_POINT ( 'NONE',  ( -61.36325649057781817, -43.03793052543183251, 41.38025477438755928 ) ) ;
#12418=DIRECTION ( 'NONE',  ( 0.000000000000000000, 0.000000000000000000, 1.000000000000000000 ) ) ;
#12428=EDGE_LOOP ( 'NONE', ( #62003, #34423, #45220, #33438 ) ) ;
#12436=CARTESIAN_POINT ( 'NONE',  ( 42.52268464718238050, 51.31691565899355822, 34.48241795236666718 ) ) ;
#12440=DIRECTION ( 'NONE',  ( 0.000000000000000000, -0.000000000000000000, -1.000000000000000000 ) ) ;
#12442=ORIENTED_EDGE ( 'NONE', *, *, #15120, .F. ) ;
#12454=EDGE_CURVE ( 'NONE', #28975, #1146, #69115, .T. ) ;
#12456=LINE ( 'NONE', #40231, #58846 ) ;
#12458=CARTESIAN_POINT ( 'NONE',  ( 47.70222499156840712, -57.81185381817577706, 41.38025477438755928 ) ) ;
#12459=DIRECTION ( 'NONE',  ( -0.000000000000000000, -0.000000000000000000, -1.000000000000000000 ) ) ;
#12461=ORIENTED_EDGE ( 'NONE', *, *, #1270, .F. ) ;
#12465=CARTESIAN_POINT ( 'NONE',  ( 41.72486082342823721, -50.31647622756196370, 43.58025477438756212 ) ) ;
#12476=VECTOR ( 'NONE', #45844, 1000.000000000000000 ) ;
#12480=ADVANCED_FACE ( 'NONE', ( #65450 ), #12329, .F. ) ;
#12491=DIRECTION ( 'NONE',  ( 0.000000000000000000, 0.000000000000000000, 1.000000000000000000 ) ) ;
#12492=VERTEX_POINT ( 'NONE', #12678 ) ;
#12498=LINE ( 'NONE', #22695, #22497 ) ;
#12503=ORIENTED_EDGE ( 'NONE', *, *, #67282, .T. ) ;
#12508=DIRECTION ( 'NONE',  ( 2.377681859532301304E-16, -7.725556675377196710E-17, 1.000000000000000000 ) ) ;
#12509=ORIENTED_EDGE ( 'NONE', *, *, #61698, .F. ) ;
#12514=CARTESIAN_POINT ( 'NONE',  ( -8.663926357539105894, 23.45072237844991747, 0.000000000000000000 ) ) ;
#12525=DIRECTION ( 'NONE',  ( 1.000000000000000000, 0.000000000000000000, -0.000000000000000000 ) ) ;
#12526=CARTESIAN_POINT ( 'NONE',  ( 0.000000000000000000, 0.000000000000000000, 0.000000000000000000 ) ) ;
#12528=AXIS2_PLACEMENT_3D ( 'NONE', #6770, #39144, #46134 ) ;
#12536=AXIS2_PLACEMENT_3D ( 'NONE', #6358, #43281, #15869 ) ;
#12539=EDGE_CURVE ( 'NONE', #6204, #67474, #22183, .T. ) ;
#12543=CARTESIAN_POINT ( 'NONE',  ( -66.47744250486724127, 4.728025645033430813, 34.48241823979542886 ) ) ;
#12552=PLANE ( 'NONE',  #13817 ) ;
#12565=ADVANCED_FACE ( 'NONE', ( #16896 ), #17605, .T. ) ;
#12566=CARTESIAN_POINT ( 'NONE',  ( -74.58602291351357394, -7.967916035252095242, 170.0000000000000000 ) ) ;
#12572=B_SPLINE_CURVE_WITH_KNOTS ( 'NONE', 3,
 ( #2516, #40833, #35564, #19728 ),
 .UNSPECIFIED., .F., .F.,
 ( 4, 4 ),
 ( 9.900409499046083621E-07, 0.05658314289920116785 ),
 .UNSPECIFIED. ) ;
#12575=ORIENTED_EDGE ( 'NONE', *, *, #35158, .T. ) ;
#12580=FACE_OUTER_BOUND ( 'NONE', #14407, .T. ) ;
#12586=ORIENTED_EDGE ( 'NONE', *, *, #58368, .T. ) ;
#12593=VERTEX_POINT ( 'NONE', #48888 ) ;
#12595=CLOSED_SHELL ( 'NONE', ( #59211, #38605, #8657, #14556, #18517, #15863, #67916, #11424, #28835, #39977, #66406, #55361, #1296, #20248, #9603, #15227, #15490, #24645, #15173, #41841, #23292, #41050, #33464, #55568, #60821, #23493, #34149, #7062, #32269, #40119, #55264, #14692, #23516, #44855, #47740, #5048, #9546, #66904, #48472, #6191, #36845, #8123, #8991, #28954, #55573, #19866, #40643, #9625, #49293, #34029, #35606, #68244, #66564, #14512, #33898, #38651, #725, #7314, #67207, #56054, #33634, #32156, #60426, #38700, #45393, #52469, #52703, #9535, #22154, #58929, #9707, #47018, #17805, #44803, #40720, #63294, #6827, #15156, #40903, #20194, #3897, #39533, #60102, #58517, #30390, #27440, #54525, #21566, #17701, #23433, #29915, #40197, #24947, #11168, #35009, #33281, #5464, #54061, #2153, #17973, #22020, #61940, #57215, #32081, #55937, #65515, #13714, #35408, #61877, #43963, #36874, #41235, #13971, #62254, #49537, #40840, #11576, #10593, #6846, #54461, #6193, #24470, #50829, #11044, #2700, #67084, #9292, #44457, #10459, #69160, #17106, #68443, #16104, #18733, #44324, #36300, #46059, #29732, #67742, #46204, #45493, #16295, #28284, #45181, #55755, #54422, #39112, #43266, #39636, #57664, #35112, #33117, #13880, #23740, #26623, #22466, #20017, #61880, #55343, #57941, #58826, #17373, #40654, #65836, #30006, #8924, #42795, #66083, #33522, #25851, #66648, #48897, #18684, #1295, #18849, #43722, #42691, #1345, #27863, #64188, #21599, #46375, #60191, #25761, #58590, #65737, #64858, #51767, #17659, #10241, #13908, #40100, #37137, #66627, #32541, #13744, #12565, #64365, #8532, #47297, #9128, #15001, #11919, #46199, #14945, #64217, #41198, #58032, #47214, #37381, #52042, #60526, #9460, #64322, #27944, #21812, #60124, #41720, #45583, #39491, #68227, #62956, #52167, #16497, #59074, #27872, #51408, #7640, #53181, #10418, #10019, #53242, #54560, #7226, #1604, #4671, #44544, #11667, #64083, #29080, #36614, #3818, #68318, #44996, #38912, #67455, #52850, #19777, #23285, #52162, #2218, #45730, #60073, #4780, #61132, #67073, #50916, #34827, #9208, #17956, #4401, #9790, #39942, #5707, #11748, #2714, #35998, #63040, #12480, #26702, #47460, #22733, #24869, #48034, #3523, #36275, #63999, #5386, #37884, #23170, #30568, #407, #49662, #52951, #8593, #16486, #775, #1127, #65295, #15408, #56467, #63218, #30732, #37064, #41299, #63638, #56698, #13518, #35588, #27206, #24056, #65434, #44938, #16504, #7862, #55503, #15870, #52038, #13344, #5826, #49483, #26181, #53594, #60500, #13683, #61929, #2719, #23441, #23594, #56934, #1693, #31210, #9444, #3560, #60360, #38104, #5148, #11045, #36558, #24073, #65744, #44747, #49121, #40569, #7689, #64402, #62492, #54361, #12646, #16203, #26522, #69319, #57185, #69124, #19683, #42556, #34085, #44567, #39950, #28991, #962, #18182, #60431, #7743 ) ) ;
#12604=EDGE_LOOP ( 'NONE', ( #14217, #30313, #39326, #17948 ) ) ;
#12613=EDGE_CURVE ( 'NONE', #16637, #60863, #54522, .T. ) ;
#12614=CARTESIAN_POINT ( 'NONE',  ( -59.94154301275507635, -45.09516516490467808, 170.0000000000000000 ) ) ;
#12616=EDGE_CURVE ( 'NONE', #25903, #6273, #27806, .T. ) ;
#12621=EDGE_CURVE ( 'NONE', #21254, #22088, #6357, .T. ) ;
#12622=FACE_OUTER_BOUND ( 'NONE', #13723, .T. ) ;
#12630=LINE ( 'NONE', #18599, #46130 ) ;
#12636=DIRECTION ( 'NONE',  ( -0.04486483035051862939, 0.9989930665413143673, 1.037707659396819425E-17 ) ) ;
#12639=ORIENTED_EDGE ( 'NONE', *, *, #42706, .F. ) ;
#12646=ADVANCED_FACE ( 'NONE', ( #378 ), #48204, .F. ) ;
#12648=AXIS2_PLACEMENT_3D ( 'NONE', #42834, #10146, #31607 ) ;
#12662=CARTESIAN_POINT ( 'NONE',  ( -60.41792053122280493, 24.01035990323433822, 43.58025477438756923 ) ) ;
#12664=CARTESIAN_POINT ( 'NONE',  ( 11.29825944729837062, -74.09495289492984682, 41.38025477438755928 ) ) ;
#12672=ORIENTED_EDGE ( 'NONE', *, *, #67075, .F. ) ;
#12674=DIRECTION ( 'NONE',  ( 0.3930250316539148359, 0.9195277725514544587, 0.000000000000000000 ) ) ;
#12678=CARTESIAN_POINT ( 'NONE',  ( -58.00979178563811445, -29.32343869649178814, 170.0000000000000000 ) ) ;
#12679=VECTOR ( 'NONE', #16689, 1000.000000000000000 ) ;
#12687=B_SPLINE_CURVE_WITH_KNOTS ( 'NONE', 3,
 ( #11466, #43131, #54374, #59316, #32593, #21682 ),
 .UNSPECIFIED., .F., .F.,
 ( 4, 2, 4 ),
 ( 1.095770181098974840E-06, 0.03239442681617710901, 0.06478775786217311206 ),
 .UNSPECIFIED. ) ;
#12691=ORIENTED_EDGE ( 'NONE', *, *, #6365, .F. ) ;
#12692=CIRCLE ( 'NONE', #1439, 74.95140232871122521 ) ;
#12701=EDGE_CURVE ( 'NONE', #26321, #28516, #37102, .T. ) ;
#12712=CARTESIAN_POINT ( 'NONE',  ( 0.000000000000000000, 0.000000000000000000, 0.000000000000000000 ) ) ;
#12717=CARTESIAN_POINT ( 'NONE',  ( 47.73902449249074920, -57.85799893277823713, 170.0000000000000000 ) ) ;
#12718=ORIENTED_EDGE ( 'NONE', *, *, #4375, .F. ) ;
#12722=DIRECTION ( 'NONE',  ( 0.9839295885986295565, 0.1785568947986370392, 0.000000000000000000 ) ) ;
#12738=CIRCLE ( 'NONE', #23984, 65.36598343705435354 ) ;
#12743=AXIS2_PLACEMENT_3D ( 'NONE', #49363, #1197, #66290 ) ;
#12755=CARTESIAN_POINT ( 'NONE',  ( 0.000000000000000000, 0.000000000000000000, 40.00000000000003553 ) ) ;
#12758=VERTEX_POINT ( 'NONE', #21484 ) ;
#12759=ORIENTED_EDGE ( 'NONE', *, *, #53426, .F. ) ;
#12767=CARTESIAN_POINT ( 'NONE',  ( 70.34686579112810989, 18.11777090454212313, 3.061616997868437868E-16 ) ) ;
#12769=VECTOR ( 'NONE', #59939, 1000.000000000000114 ) ;
#12771=DIRECTION ( 'NONE',  ( 0.4738686624729966379, 0.8805955318567391110, 0.000000000000000000 ) ) ;
#12776=ORIENTED_EDGE ( 'NONE', *, *, #2246, .F. ) ;
#12778=VECTOR ( 'NONE', #15574, 1000.000000000000227 ) ;
#12784=AXIS2_PLACEMENT_3D ( 'NONE', #26372, #49179, #54102 ) ;
#12787=AXIS2_PLACEMENT_3D ( 'NONE', #29347, #56779, #14551 ) ;
#12796=VERTEX_POINT ( 'NONE', #32743 ) ;
#12804=CARTESIAN_POINT ( 'NONE',  ( 0.000000000000000000, 0.000000000000000000, 0.000000000000000000 ) ) ;
#12809=DIRECTION ( 'NONE',  ( 0.5877852522924802425, -0.8090169943749422332, 2.500042656554809847E-16 ) ) ;
#12811=DIRECTION ( 'NONE',  ( 0.000000000000000000, 0.000000000000000000, 1.000000000000000000 ) ) ;
#12816=DIRECTION ( 'NONE',  ( -0.000000000000000000, -0.000000000000000000, -1.000000000000000000 ) ) ;
#12817=EDGE_CURVE ( 'NONE', #8346, #30965, #60372, .T. ) ;
#12821=DIRECTION ( 'NONE',  ( 0.6910626489868580968, 0.7227948638273978821, 0.000000000000000000 ) ) ;
#12830=VECTOR ( 'NONE', #65445, 1000.000000000000000 ) ;
#12837=DIRECTION ( 'NONE',  ( -0.8584487936018727616, 0.5128992774058949156, 0.000000000000000000 ) ) ;
#12841=VECTOR ( 'NONE', #23232, 1000.000000000000000 ) ;
#12843=AXIS2_PLACEMENT_3D ( 'NONE', #50297, #2117, #23567 ) ;
#12845=VERTEX_POINT ( 'NONE', #54531 ) ;
#12846=ORIENTED_EDGE ( 'NONE', *, *, #66990, .F. ) ;
#12847=CIRCLE ( 'NONE', #24040, 65.00000000000000000 ) ;
#12852=DIRECTION ( 'NONE',  ( -0.000000000000000000, -0.000000000000000000, -1.000000000000000000 ) ) ;
#12869=ORIENTED_EDGE ( 'NONE', *, *, #554, .T. ) ;
#12880=CARTESIAN_POINT ( 'NONE',  ( 0.000000000000000000, 0.000000000000000000, 43.58025477438756212 ) ) ;
#12881=ORIENTED_EDGE ( 'NONE', *, *, #65354, .F. ) ;
#12885=DIRECTION ( 'NONE',  ( -1.357354004351002108E-18, 4.918261777702510883E-18, -1.000000000000000000 ) ) ;
#12888=LINE ( 'NONE', #6557, #6793 ) ;
#12892=CARTESIAN_POINT ( 'NONE',  ( -65.36598343705435354, 0.000000000000000000, 41.38025477438755928 ) ) ;
#12893=ORIENTED_EDGE ( 'NONE', *, *, #10483, .F. ) ;
#12894=EDGE_LOOP ( 'NONE', ( #27729, #38228, #17677, #63180 ) ) ;
#12895=CIRCLE ( 'NONE', #18509, 65.00000000000000000 ) ;
#12898=VECTOR ( 'NONE', #28139, 1000.000000000000227 ) ;
#12901=CARTESIAN_POINT ( 'NONE',  ( -41.05116106442372370, -31.37049930917697083, 26.66469066592269144 ) ) ;
#12910=CARTESIAN_POINT ( 'NONE',  ( 33.53140150161104316, 18.57796495195515618, 13.32819397642333747 ) ) ;
#12911=ORIENTED_EDGE ( 'NONE', *, *, #15175, .T. ) ;
#12916=PLANE ( 'NONE',  #54578 ) ;
#12931=CARTESIAN_POINT ( 'NONE',  ( 0.000000000000000000, 0.000000000000000000, 41.38025477438755928 ) ) ;
#12946=DIRECTION ( 'NONE',  ( -0.000000000000000000, 0.000000000000000000, -1.000000000000000000 ) ) ;
#12951=ORIENTED_EDGE ( 'NONE', *, *, #31782, .F. ) ;
#12979=LINE ( 'NONE', #66803, #354 ) ;
#12981=AXIS2_PLACEMENT_3D ( 'NONE', #37255, #53428, #3885 ) ;
#12984=FACE_OUTER_BOUND ( 'NONE', #19722, .T. ) ;
#12987=CARTESIAN_POINT ( 'NONE',  ( 0.000000000000000000, 0.000000000000000000, 0.000000000000000000 ) ) ;
#12990=DIRECTION ( 'NONE',  ( -0.2225209339563184729, 0.9749279121818227312, 0.000000000000000000 ) ) ;
#13000=CIRCLE ( 'NONE', #52291, 74.95140232871122521 ) ;
#13024=ORIENTED_EDGE ( 'NONE', *, *, #61996, .F. ) ;
#13034=ORIENTED_EDGE ( 'NONE', *, *, #49141, .F. ) ;
#13053=EDGE_CURVE ( 'NONE', #41640, #4543, #15655, .T. ) ;
#13054=VERTEX_POINT ( 'NONE', #18226 ) ;
#13069=CARTESIAN_POINT ( 'NONE',  ( 0.000000000000000000, 0.000000000000000000, 170.0000000000000000 ) ) ;
#13070=CARTESIAN_POINT ( 'NONE',  ( 30.83327723550665311, -12.90705755941334942, 6.893343212288926658 ) ) ;
#13074=ORIENTED_EDGE ( 'NONE', *, *, #36033, .T. ) ;
#13077=CARTESIAN_POINT ( 'NONE',  ( -11.01093400780253084, 22.58090174195383781, 3.061616997868437868E-16 ) ) ;
#13078=DIRECTION ( 'NONE',  ( 0.9362348706397417564, -0.3513748240813305279, 0.000000000000000000 ) ) ;
#13079=AXIS2_PLACEMENT_3D ( 'NONE', #32494, #58521, #49346 ) ;
#13085=CARTESIAN_POINT ( 'NONE',  ( -29.87147652227455907, 68.79592317125366208, 73.58025477438756923 ) ) ;
#13086=AXIS2_PLACEMENT_3D ( 'NONE', #2118, #66492, #39740 ) ;
#13092=EDGE_CURVE ( 'NONE', #2204, #16163, #67659, .T. ) ;
#13094=VERTEX_POINT ( 'NONE', #23510 ) ;
#13101=EDGE_CURVE ( 'NONE', #6090, #32844, #48209, .T. ) ;
#13114=EDGE_CURVE ( 'NONE', #41523, #63790, #35444, .T. ) ;
#13115=ORIENTED_EDGE ( 'NONE', *, *, #65510, .F. ) ;
#13129=CARTESIAN_POINT ( 'NONE',  ( -67.03031041878467988, 33.66749151869449008, 43.58025477438756212 ) ) ;
#13141=CARTESIAN_POINT ( 'NONE',  ( 21.80334785612273762, 25.33568910032904142, 6.893343212288939093 ) ) ;
#13159=CARTESIAN_POINT ( 'NONE',  ( -57.97933236950880342, -6.473286833963715736, 27.58472369368490718 ) ) ;
#13160=CARTESIAN_POINT ( 'NONE',  ( -11.01093400780253084, 22.58090174195383781, 3.061616997868437868E-16 ) ) ;
#13164=EDGE_LOOP ( 'NONE', ( #18745, #61449, #6149, #59596, #62272, #44730, #29807, #17178, #42079, #44013, #63020, #53045, #10738, #24707, #6989, #29935, #11774, #59400, #25229, #9741, #14498, #18149, #35459, #37646, #66195, #26062, #56713, #46817, #33279, #10346, #52068, #44312, #33070, #33354, #47903, #12053, #45951, #65887, #63337, #36333, #39274, #38954, #8962, #11036, #1948, #20229, #49549, #4210, #40522, #11097, #41888, #39240, #26750, #18370, #18420, #8706, #30476, #51438, #11155, #65072, #19943, #57431, #11050, #16553, #44426, #27531, #44587, #61892, #9334, #1388, #10358, #214, #23208, #26556, #34415, #16509, #57033, #50809, #27374, #37339, #24263, #36596, #24600, #37930, #739, #49014, #41492, #44815, #38491, #5551, #7886, #9639, #18806, #60079, #30187, #16284, #51629, #20653, #25220, #6346, #39116, #39403, #47861, #9054, #12575, #21589, #42091, #16232, #42742, #35876, #2424, #20471, #52672, #69095, #48680, #17439, #45096, #62458, #50354, #36635, #3214, #68832, #46667, #37590, #60635, #46008, #5441, #57288, #51205, #43896, #66602, #43166, #45457, #27427, #34065, #53865, #27740, #63793, #7632, #45728, #28127 ) ) ;
#13175=DIRECTION ( 'NONE',  ( -0.000000000000000000, -0.000000000000000000, -1.000000000000000000 ) ) ;
#13190=EDGE_CURVE ( 'NONE', #4577, #23405, #57301, .T. ) ;
#13193=LINE ( 'NONE', #45533, #52142 ) ;
#13204=VERTEX_POINT ( 'NONE', #30173 ) ;
#13205=CARTESIAN_POINT ( 'NONE',  ( -11.75099048680785785, -77.43714764088365143, 73.58025477438756923 ) ) ;
#13209=DIRECTION ( 'NONE',  ( 0.8805955318567391110, -0.4738686624729966379, 5.102127870520020458E-18 ) ) ;
#13228=AXIS2_PLACEMENT_3D ( 'NONE', #59850, #23296, #28916 ) ;
#13230=DIRECTION ( 'NONE',  ( 0.000000000000000000, 0.000000000000000000, 1.000000000000000000 ) ) ;
#13233=CARTESIAN_POINT ( 'NONE',  ( 0.000000000000000000, 0.000000000000000000, 41.38025477438755928 ) ) ;
#13238=ORIENTED_EDGE ( 'NONE', *, *, #53488, .T. ) ;
#13240=ORIENTED_EDGE ( 'NONE', *, *, #55330, .F. ) ;
#13253=CARTESIAN_POINT ( 'NONE',  ( 41.26323129469689377, -6.217756351907037349, 13.79046412291064172 ) ) ;
#13257=CARTESIAN_POINT ( 'NONE',  ( 53.32245423372616244, -37.19594572654634845, 41.38025477438755928 ) ) ;
#13268=DIRECTION ( 'NONE',  ( -0.3930250316539147803, -0.9195277725514544587, 0.000000000000000000 ) ) ;
#13271=CARTESIAN_POINT ( 'NONE',  ( 64.38365952013991489, 38.46744580544303460, 43.58025477438756212 ) ) ;
#13274=VECTOR ( 'NONE', #40926, 999.9999999999998863 ) ;
#13290=ORIENTED_EDGE ( 'NONE', *, *, #57502, .T. ) ;
#13292=EDGE_CURVE ( 'NONE', #34263, #37573, #31544, .T. ) ;
#13307=CARTESIAN_POINT ( 'NONE',  ( 24.36509522348982060, 70.94296747916789059, 73.58025477438755502 ) ) ;
#13308=VERTEX_POINT ( 'NONE', #43811 ) ;
#13309=ORIENTED_EDGE ( 'NONE', *, *, #31825, .F. ) ;
#13318=ORIENTED_EDGE ( 'NONE', *, *, #41240, .F. ) ;
#13322=DIRECTION ( 'NONE',  ( -6.651034621319910312E-17, 2.409948271074229917E-16, 1.000000000000000000 ) ) ;
#13324=ORIENTED_EDGE ( 'NONE', *, *, #56385, .F. ) ;
#13327=CIRCLE ( 'NONE', #21149, 24.17157287525367693 ) ;
#13330=CARTESIAN_POINT ( 'NONE',  ( -59.42430146430427129, 27.22983999535711064, 41.38025477438755928 ) ) ;
#13331=CIRCLE ( 'NONE', #69488, 65.36598343705435354 ) ;
#13344=ADVANCED_FACE ( 'NONE', ( #35628 ), #35275, .F. ) ;
#13347=LINE ( 'NONE', #26823, #13836 ) ;
#13354=DIRECTION ( 'NONE',  ( -0.9362348706397417564, 0.3513748240813305279, 0.000000000000000000 ) ) ;
#13355=EDGE_CURVE ( 'NONE', #8019, #34646, #44528, .T. ) ;
#13358=EDGE_CURVE ( 'NONE', #39568, #32990, #26140, .T. ) ;
#13364=PLANE ( 'NONE',  #9474 ) ;
#13377=DIRECTION ( 'NONE',  ( 1.000000000000000000, 0.000000000000000000, 0.000000000000000000 ) ) ;
#13379=EDGE_CURVE ( 'NONE', #28345, #64668, #29171, .T. ) ;
#13390=ORIENTED_EDGE ( 'NONE', *, *, #31613, .T. ) ;
#13401=CARTESIAN_POINT ( 'NONE',  ( 29.69502258243432635, -57.82046033912835270, 40.00000000000003553 ) ) ;
#13406=CARTESIAN_POINT ( 'NONE',  ( 0.000000000000000000, 0.000000000000000000, 43.58025477438756212 ) ) ;
#13411=CARTESIAN_POINT ( 'NONE',  ( -24.39249304643438521, 60.24953346690454481, 73.58025477438756923 ) ) ;
#13414=EDGE_CURVE ( 'NONE', #51882, #3940, #34805, .T. ) ;
#13416=CARTESIAN_POINT ( 'NONE',  ( 26.12852347772543737, 70.00000000000000000, 77.58025477438755502 ) ) ;
#13417=CARTESIAN_POINT ( 'NONE',  ( -63.73419499958981049, -12.83646726144931449, 41.38025477438755928 ) ) ;
#13425=CARTESIAN_POINT ( 'NONE',  ( -18.89790202299209199, 62.20684691518605547, 41.38025477438755928 ) ) ;
#13430=EDGE_CURVE ( 'NONE', #18218, #50410, #17079, .T. ) ;
#13437=CARTESIAN_POINT ( 'NONE',  ( 45.82394788922798767, 46.11928342727497210, 170.0000000000000000 ) ) ;
#13440=AXIS2_PLACEMENT_3D ( 'NONE', #61485, #29467, #2743 ) ;
#13443=CARTESIAN_POINT ( 'NONE',  ( 0.000000000000000000, 0.000000000000000000, 0.000000000000000000 ) ) ;
#13445=ORIENTED_EDGE ( 'NONE', *, *, #8300, .F. ) ;
#13447=VERTEX_POINT ( 'NONE', #37330 ) ;
#13451=LINE ( 'NONE', #50727, #11140 ) ;
#13455=VECTOR ( 'NONE', #40209, 1000.000000000000000 ) ;
#13469=AXIS2_PLACEMENT_3D ( 'NONE', #16621, #22598, #33521 ) ;
#13470=ORIENTED_EDGE ( 'NONE', *, *, #9830, .F. ) ;
#13473=CARTESIAN_POINT ( 'NONE',  ( 53.32245423372616244, -37.19594572654634845, 170.0000000000000000 ) ) ;
#13478=CARTESIAN_POINT ( 'NONE',  ( 24.36509522348982060, 70.94296747916789059, 170.0000000000000000 ) ) ;
#13483=VERTEX_POINT ( 'NONE', #9926 ) ;
#13491=DIRECTION ( 'NONE',  ( 1.000000000000000000, 0.000000000000000000, 0.000000000000000000 ) ) ;
#13496=ORIENTED_EDGE ( 'NONE', *, *, #1490, .T. ) ;
#13500=CARTESIAN_POINT ( 'NONE',  ( -41.43037476669420016, -4.983853691429483312, 13.79046412286062306 ) ) ;
#13505=EDGE_CURVE ( 'NONE', #28214, #51807, #31138, .T. ) ;
#13518=ADVANCED_FACE ( 'NONE', ( #43642 ), #1447, .T. ) ;
#13529=B_SPLINE_CURVE_WITH_KNOTS ( 'NONE', 3,
 ( #59729, #34431, #44960, #17529 ),
 .UNSPECIFIED., .F., .F.,
 ( 4, 4 ),
 ( 9.900409499053008115E-07, 0.05658314289920116785 ),
 .UNSPECIFIED. ) ;
#13530=ORIENTED_EDGE ( 'NONE', *, *, #30823, .F. ) ;
#13534=CARTESIAN_POINT ( 'NONE',  ( 47.73902449248994628, 57.85799893277891215, 43.58025477438756212 ) ) ;
#13536=CARTESIAN_POINT ( 'NONE',  ( 51.04336025769664076, 7.992588086412792059, 26.66469104408688651 ) ) ;
#13551=DIRECTION ( 'NONE',  ( -1.000000000000000000, 0.000000000000000000, 0.000000000000000000 ) ) ;
#13552=CARTESIAN_POINT ( 'NONE',  ( 75.00000000000000000, 1.249999999999979350, 170.0000000000000000 ) ) ;
#13553=ORIENTED_EDGE ( 'NONE', *, *, #69261, .T. ) ;
#13556=ORIENTED_EDGE ( 'NONE', *, *, #797, .F. ) ;
#13559=DIRECTION ( 'NONE',  ( -0.000000000000000000, -0.000000000000000000, 1.000000000000000000 ) ) ;
#13560=PLANE ( 'NONE',  #58601 ) ;
#13564=CARTESIAN_POINT ( 'NONE',  ( -31.90315521289063128, -56.64813493366051489, 170.0000000000000000 ) ) ;
#13565=ORIENTED_EDGE ( 'NONE', *, *, #54238, .F. ) ;
#13568=LINE ( 'NONE', #33988, #37976 ) ;
#13583=EDGE_CURVE ( 'NONE', #2845, #64522, #19355, .T. ) ;
#13587=( GEOMETRIC_REPRESENTATION_CONTEXT ( 3 ) GLOBAL_UNCERTAINTY_ASSIGNED_CONTEXT ( ( #40235 ) ) GLOBAL_UNIT_ASSIGNED_CONTEXT ( ( #47079, #24609, #62924 ) ) REPRESENTATION_CONTEXT ( 'NONE', 'WORKASPACE' ) );
#13607=CARTESIAN_POINT ( 'NONE',  ( -46.06722295615789875, 46.37372919877054755, 41.38025477438755928 ) ) ;
#13612=CARTESIAN_POINT ( 'NONE',  ( 32.06997139192709767, 56.95813133885488355, 43.58025477438756212 ) ) ;
#13615=CARTESIAN_POINT ( 'NONE',  ( -16.43619359402603664, -18.99971924381128474, 3.061616997868437868E-16 ) ) ;
#13620=ORIENTED_EDGE ( 'NONE', *, *, #24634, .T. ) ;
#13630=AXIS2_PLACEMENT_3D ( 'NONE', #7906, #29703, #51165 ) ;
#13634=AXIS2_PLACEMENT_3D ( 'NONE', #24918, #36852, #25618 ) ;
#13643=VECTOR ( 'NONE', #61248, 1000.000000000000114 ) ;
#13653=EDGE_CURVE ( 'NONE', #39038, #68160, #26893, .T. ) ;
#13654=EDGE_LOOP ( 'NONE', ( #14823, #29626, #23861, #51943 ) ) ;
#13656=CARTESIAN_POINT ( 'NONE',  ( 55.65793654284612302, 50.28674377798304107, 170.0000000000000000 ) ) ;
#13658=DIRECTION ( 'NONE',  ( 1.000000000000000000, 0.000000000000000000, 0.000000000000000000 ) ) ;
#13660=DIRECTION ( 'NONE',  ( -0.9839295885986295565, -0.1785568947986370392, 0.000000000000000000 ) ) ;
#13669=ORIENTED_EDGE ( 'NONE', *, *, #26960, .T. ) ;
#13671=CARTESIAN_POINT ( 'NONE',  ( -39.55079474733624068, -51.59997227571039957, 170.0000000000000000 ) ) ;
#13678=EDGE_CURVE ( 'NONE', #33970, #13204, #57343, .T. ) ;
#13679=VERTEX_POINT ( 'NONE', #57000 ) ;
#13680=VECTOR ( 'NONE', #20509, 1000.000000000000000 ) ;
#13683=ADVANCED_FACE ( 'NONE', ( #20738 ), #63660, .F. ) ;
#13694=AXIS2_PLACEMENT_3D ( 'NONE', #35133, #51325, #3139 ) ;
#13705=ORIENTED_EDGE ( 'NONE', *, *, #50896, .T. ) ;
#13714=ADVANCED_FACE ( 'NONE', ( #65031 ), #64685, .T. ) ;
#13723=EDGE_LOOP ( 'NONE', ( #32213, #57682, #49015, #14936 ) ) ;
#13732=FACE_OUTER_BOUND ( 'NONE', #13654, .T. ) ;
#13737=CARTESIAN_POINT ( 'NONE',  ( -44.00727179482512241, -47.83680621839620528, 170.0000000000000000 ) ) ;
#13742=ORIENTED_EDGE ( 'NONE', *, *, #31396, .T. ) ;
#13744=ADVANCED_FACE ( 'NONE', ( #5584 ), #5919, .T. ) ;
#13759=DIRECTION ( 'NONE',  ( 1.000000000000000000, 0.000000000000000000, -0.000000000000000000 ) ) ;
#13762=EDGE_CURVE ( 'NONE', #16778, #8019, #38291, .T. ) ;
#13771=LINE ( 'NONE', #40503, #32390 ) ;
#13774=DIRECTION ( 'NONE',  ( 2.298858655265451588E-16, 9.825793442286241754E-17, 1.000000000000000000 ) ) ;
#13784=FACE_OUTER_BOUND ( 'NONE', #31737, .T. ) ;
#13790=VERTEX_POINT ( 'NONE', #27734 ) ;
#13796=DIRECTION ( 'NONE',  ( -1.000000000000000000, 0.000000000000000000, 0.000000000000000000 ) ) ;
#13797=EDGE_CURVE ( 'NONE', #53534, #37383, #27382, .T. ) ;
#13799=CARTESIAN_POINT ( 'NONE',  ( 7.484861546145031852, 64.56761454192836425, 40.00000000000003553 ) ) ;
#13802=DIRECTION ( 'NONE',  ( -0.3513748240813304724, -0.9362348706397417564, 0.000000000000000000 ) ) ;
#13816=ORIENTED_EDGE ( 'NONE', *, *, #38377, .F. ) ;
#13817=AXIS2_PLACEMENT_3D ( 'NONE', #55099, #1647, #38230 ) ;
#13824=DIRECTION ( 'NONE',  ( 0.000000000000000000, 0.000000000000000000, 1.000000000000000000 ) ) ;
#13826=DIRECTION ( 'NONE',  ( -0.000000000000000000, -0.000000000000000000, -1.000000000000000000 ) ) ;
#13834=ORIENTED_EDGE ( 'NONE', *, *, #6424, .F. ) ;
#13835=ORIENTED_EDGE ( 'NONE', *, *, #36362, .T. ) ;
#13836=VECTOR ( 'NONE', #48250, 1000.000000000000114 ) ;
#13851=CARTESIAN_POINT ( 'NONE',  ( -64.83840629396345889, -4.580509716060184644, 40.00000000000003553 ) ) ;
#13873=DIRECTION ( 'NONE',  ( -0.04486483035050447404, -0.9989930665413151445, 0.000000000000000000 ) ) ;
#13874=DIRECTION ( 'NONE',  ( 0.8584487936018655452, 0.5128992774059070170, 0.000000000000000000 ) ) ;
#13878=CARTESIAN_POINT ( 'NONE',  ( -15.47041015649555185, -73.39774458108232125, 170.0000000000000000 ) ) ;
#13880=ADVANCED_FACE ( 'NONE', ( #304 ), #59395, .T. ) ;
#13886=VECTOR ( 'NONE', #11961, 1000.000000000000114 ) ;
#13887=DIRECTION ( 'NONE',  ( 0.6234898018587318180, 0.7818314824680311359, 0.000000000000000000 ) ) ;
#13894=AXIS2_PLACEMENT_3D ( 'NONE', #1733, #54118, #27055 ) ;
#13895=ORIENTED_EDGE ( 'NONE', *, *, #17565, .T. ) ;
#13896=LINE ( 'NONE', #45210, #25641 ) ;
#13898=DIRECTION ( 'NONE',  ( 1.000000000000000000, 0.000000000000000000, 0.000000000000000000 ) ) ;
#13903=CARTESIAN_POINT ( 'NONE',  ( 39.77028211725738771, 51.87520073220943573, 3.125053320693569132E-16 ) ) ;
#13908=ADVANCED_FACE ( 'NONE', ( #29138 ), #29479, .T. ) ;
#13925=AXIS2_PLACEMENT_3D ( 'NONE', #67663, #3627, #68681 ) ;
#13931=ORIENTED_EDGE ( 'NONE', *, *, #3986, .F. ) ;
#13936=CIRCLE ( 'NONE', #50995, 74.95140232871122521 ) ;
#13939=AXIS2_PLACEMENT_3D ( 'NONE', #16626, #59877, #60588 ) ;
#13944=VECTOR ( 'NONE', #32785, 1000.000000000000000 ) ;
#13945=DIRECTION ( 'NONE',  ( -0.9009688679024218105, 0.4338837391175525693, 0.000000000000000000 ) ) ;
#13948=DIRECTION ( 'NONE',  ( 4.463998536185623432E-17, -2.459865942542999442E-16, 1.000000000000000000 ) ) ;
#13950=VERTEX_POINT ( 'NONE', #12265 ) ;
#13959=CARTESIAN_POINT ( 'NONE',  ( -18.24318075359480318, 17.27206262134385284, 3.061616997868437868E-16 ) ) ;
#13960=FACE_OUTER_BOUND ( 'NONE', #51892, .T. ) ;
#13962=CARTESIAN_POINT ( 'NONE',  ( -2.374459999240554620, 25.00999262126967437, 3.061616997868437868E-16 ) ) ;
#13963=LINE ( 'NONE', #8353, #1630 ) ;
#13967=ORIENTED_EDGE ( 'NONE', *, *, #63163, .T. ) ;
#13968=VERTEX_POINT ( 'NONE', #60789 ) ;
#13971=ADVANCED_FACE ( 'NONE', ( #8383 ), #56208, .T. ) ;
#13973=AXIS2_PLACEMENT_3D ( 'NONE', #65322, #11149, #33325 ) ;
#13981=CARTESIAN_POINT ( 'NONE',  ( 15.68296563925494702, 63.09411298019766434, 170.0000000000000000 ) ) ;
#13986=VECTOR ( 'NONE', #6693, 1000.000000000000000 ) ;
#13993=LINE ( 'NONE', #56911, #43533 ) ;
#14008=CARTESIAN_POINT ( 'NONE',  ( -52.73319225379862019, -53.34578647582125654, 170.0000000000000000 ) ) ;
#14010=DIRECTION ( 'NONE',  ( 0.4738686624729966379, 0.8805955318567391110, 0.000000000000000000 ) ) ;
#14013=CARTESIAN_POINT ( 'NONE',  ( -65.36598343705435354, 0.000000000000000000, 41.38025477438755928 ) ) ;
#14014=VERTEX_POINT ( 'NONE', #14682 ) ;
#14026=EDGE_LOOP ( 'NONE', ( #13835, #11606, #62804, #16611 ) ) ;
#14031=VECTOR ( 'NONE', #18489, 1000.000000000000000 ) ;
#14035=FACE_OUTER_BOUND ( 'NONE', #64389, .T. ) ;
#14040=AXIS2_PLACEMENT_3D ( 'NONE', #50141, #60341, #29378 ) ;
#14041=DIRECTION ( 'NONE',  ( 1.000000000000000000, 0.000000000000000000, 0.000000000000000000 ) ) ;
#14055=ORIENTED_EDGE ( 'NONE', *, *, #66030, .T. ) ;
#14061=CARTESIAN_POINT ( 'NONE',  ( -3.364862276288897558, 74.92447999059858432, 0.000000000000000000 ) ) ;
#14073=EDGE_LOOP ( 'NONE', ( #54119, #66193, #13895, #11051 ) ) ;
#14079=CIRCLE ( 'NONE', #11860, 65.00000000000000000 ) ;
#14085=CARTESIAN_POINT ( 'NONE',  ( 0.000000000000000000, 0.000000000000000000, 40.00000000000003553 ) ) ;
#14089=ORIENTED_EDGE ( 'NONE', *, *, #68529, .T. ) ;
#14091=ORIENTED_EDGE ( 'NONE', *, *, #12365, .T. ) ;
#14095=LINE ( 'NONE', #46096, #55862 ) ;
#14104=CARTESIAN_POINT ( 'NONE',  ( 55.65793654284683356, -50.28674377798225237, 170.0000000000000000 ) ) ;
#14115=EDGE_CURVE ( 'NONE', #35105, #67632, #27743, .T. ) ;
#14118=VECTOR ( 'NONE', #61047, 1000.000000000000000 ) ;
#14120=ORIENTED_EDGE ( 'NONE', *, *, #49118, .T. ) ;
#14123=AXIS2_PLACEMENT_3D ( 'NONE', #30356, #24044, #61324 ) ;
#14128=AXIS2_PLACEMENT_3D ( 'NONE', #62118, #62475, #46636 ) ;
#14135=ORIENTED_EDGE ( 'NONE', *, *, #37560, .T. ) ;
#14140=DIRECTION ( 'NONE',  ( -0.9639628606958550172, 0.2660368455666687892, 0.000000000000000000 ) ) ;
#14142=EDGE_CURVE ( 'NONE', #61903, #12845, #24711, .T. ) ;
#14143=ORIENTED_EDGE ( 'NONE', *, *, #17060, .T. ) ;
#14146=LINE ( 'NONE', #57396, #10000 ) ;
#14151=CARTESIAN_POINT ( 'NONE',  ( 4.606779575614314837, -24.69646479044436305, 3.061616997868437868E-16 ) ) ;
#14153=EDGE_CURVE ( 'NONE', #65974, #32844, #12687, .T. ) ;
#14155=DIRECTION ( 'NONE',  ( 1.000000000000000000, 0.000000000000000000, 0.000000000000000000 ) ) ;
#14164=DIRECTION ( 'NONE',  ( -0.5508969814520944253, -0.8345732537213078617, 0.000000000000000000 ) ) ;
#14172=CIRCLE ( 'NONE', #7454, 24.99999999999985434 ) ;
#14178=VECTOR ( 'NONE', #27314, 1000.000000000000114 ) ;
#14182=CIRCLE ( 'NONE', #38888, 65.36598343705435354 ) ;
#14192=B_SPLINE_CURVE_WITH_KNOTS ( 'NONE', 3,
 ( #62648, #14456, #52080, #25368 ),
 .UNSPECIFIED., .F., .F.,
 ( 4, 4 ),
 ( 0.1259919275528360583, 0.1829744153748752988 ),
 .UNSPECIFIED. ) ;
#14194=AXIS2_PLACEMENT_3D ( 'NONE', #21011, #30879, #42456 ) ;
#14195=CARTESIAN_POINT ( 'NONE',  ( -24.39249304643357519, -60.24953346690487166, 170.0000000000000000 ) ) ;
#14200=CARTESIAN_POINT ( 'NONE',  ( 34.76618902119740540, 54.93755186520760958, 43.58025477438756923 ) ) ;
#14205=CARTESIAN_POINT ( 'NONE',  ( 32.06997139192793611, -56.95813133885440038, 3.125053320693577513E-16 ) ) ;
#14208=EDGE_CURVE ( 'NONE', #47971, #67731, #33992, .T. ) ;
#14211=CARTESIAN_POINT ( 'NONE',  ( -29.87147652227455552, 100.0000000000000000, 133.5802547743875550 ) ) ;
#14216=DIRECTION ( 'NONE',  ( -0.9009688679024155933, -0.4338837391175656699, 0.000000000000000000 ) ) ;
#14217=ORIENTED_EDGE ( 'NONE', *, *, #57690, .T. ) ;
#14218=CARTESIAN_POINT ( 'NONE',  ( 0.000000000000000000, 0.000000000000000000, 0.000000000000000000 ) ) ;
#14225=CARTESIAN_POINT ( 'NONE',  ( 24.39800339187844003, 60.26242556095705538, 43.58025477438756923 ) ) ;
#14235=CARTESIAN_POINT ( 'NONE',  ( 19.40210665709608406, -63.75862921693536833, 34.48241795236665297 ) ) ;
#14240=EDGE_LOOP ( 'NONE', ( #7824, #57240, #62325, #42880 ) ) ;
#14242=AXIS2_PLACEMENT_3D ( 'NONE', #32917, #64938, #16046 ) ;
#14243=DIRECTION ( 'NONE',  ( 1.000000000000000000, 0.000000000000000000, 0.000000000000000000 ) ) ;
#14247=ORIENTED_EDGE ( 'NONE', *, *, #40703, .F. ) ;
#14261=ORIENTED_EDGE ( 'NONE', *, *, #50212, .T. ) ;
#14276=DIRECTION ( 'NONE',  ( -1.000000000000000000, 0.000000000000000000, 0.000000000000000000 ) ) ;
#14289=CARTESIAN_POINT ( 'NONE',  ( -37.04655464516766727, -53.85410457537912521, 41.38025477438755928 ) ) ;
#14294=VECTOR ( 'NONE', #31128, 1000.000000000000114 ) ;
#14296=ORIENTED_EDGE ( 'NONE', *, *, #14910, .T. ) ;
#14302=DIRECTION ( 'NONE',  ( 1.000000000000000000, 0.000000000000000000, 0.000000000000000000 ) ) ;
#14304=VERTEX_POINT ( 'NONE', #25177 ) ;
#14307=FACE_OUTER_BOUND ( 'NONE', #55309, .T. ) ;
#14311=ORIENTED_EDGE ( 'NONE', *, *, #35292, .T. ) ;
#14318=LINE ( 'NONE', #40350, #65662 ) ;
#14324=VECTOR ( 'NONE', #43839, 1000.000000000000000 ) ;
#14344=EDGE_LOOP ( 'NONE', ( #5344, #38261, #67796, #52453 ) ) ;
#14361=FACE_OUTER_BOUND ( 'NONE', #53255, .T. ) ;
#14363=CARTESIAN_POINT ( 'NONE',  ( -58.33959211651037435, 29.48226216511319464, 6.377659838150142091E-18 ) ) ;
#14371=VERTEX_POINT ( 'NONE', #9330 ) ;
#14372=CARTESIAN_POINT ( 'NONE',  ( -53.31111153860250340, -37.18770477615797176, 40.00000000000003553 ) ) ;
#14373=CARTESIAN_POINT ( 'NONE',  ( -24.40147488398712383, 5.437648709335531905, 0.000000000000000000 ) ) ;
#14376=FACE_OUTER_BOUND ( 'NONE', #2514, .T. ) ;
#14396=SURFACE_STYLE_USAGE ( .BOTH. , #56599 ) ;
#14407=EDGE_LOOP ( 'NONE', ( #51640, #26692, #12402, #5887 ) ) ;
#14421=LINE ( 'NONE', #41152, #59452 ) ;
#14435=DIRECTION ( 'NONE',  ( 0.000000000000000000, 0.000000000000000000, 1.000000000000000000 ) ) ;
#14445=CARTESIAN_POINT ( 'NONE',  ( 29.69502258243350923, 57.82046033912877903, 170.0000000000000000 ) ) ;
#14447=CARTESIAN_POINT ( 'NONE',  ( 53.32245423372562243, 37.19594572654712294, 43.58025477438756923 ) ) ;
#14456=CARTESIAN_POINT ( 'NONE',  ( -36.60035679358400529, 11.39778710981509668, 13.32819397642333392 ) ) ;
#14458=LINE ( 'NONE', #52431, #10308 ) ;
#14462=CARTESIAN_POINT ( 'NONE',  ( -51.33022649596136233, 5.874856473938592671, 26.66469104408688295 ) ) ;
#14469=VERTEX_POINT ( 'NONE', #497 ) ;
#14470=AXIS2_PLACEMENT_3D ( 'NONE', #16708, #1584, #59964 ) ;
#14475=DIRECTION ( 'NONE',  ( 0.000000000000000000, 0.000000000000000000, 1.000000000000000000 ) ) ;
#14480=DIRECTION ( 'NONE',  ( 0.000000000000000000, 0.000000000000000000, -1.000000000000000000 ) ) ;
#14486=ORIENTED_EDGE ( 'NONE', *, *, #33150, .F. ) ;
#14487=VERTEX_POINT ( 'NONE', #42373 ) ;
#14491=VERTEX_POINT ( 'NONE', #69091 ) ;
#14494=DIRECTION ( 'NONE',  ( -0.000000000000000000, -0.000000000000000000, -1.000000000000000000 ) ) ;
#14498=ORIENTED_EDGE ( 'NONE', *, *, #16820, .T. ) ;
#14499=EDGE_LOOP ( 'NONE', ( #28303, #35429 ) ) ;
#14500=DIRECTION ( 'NONE',  ( -1.000000000000000000, 0.000000000000000000, 0.000000000000000000 ) ) ;
#14505=DIRECTION ( 'NONE',  ( 0.9009688679024218105, -0.4338837391175525693, 0.000000000000000000 ) ) ;
#14512=ADVANCED_FACE ( 'NONE', ( #10025 ), #1144, .T. ) ;
#14515=ORIENTED_EDGE ( 'NONE', *, *, #36287, .F. ) ;
#14521=CARTESIAN_POINT ( 'NONE',  ( 8.942470798084380945, -23.47701018505899739, 3.061616997868437868E-16 ) ) ;
#14522=CARTESIAN_POINT ( 'NONE',  ( 65.35403040894466642, -1.250000000000021760, 41.38025477438755928 ) ) ;
#14524=CARTESIAN_POINT ( 'NONE',  ( -84.49322488516129681, 0.000000000000000000, 43.58025477438756212 ) ) ;
#14525=DIRECTION ( 'NONE',  ( 0.000000000000000000, 0.000000000000000000, 1.000000000000000000 ) ) ;
#14528=LINE ( 'NONE', #53863, #17187 ) ;
#14530=EDGE_CURVE ( 'NONE', #69123, #47461, #42711, .T. ) ;
#14535=DIRECTION ( 'NONE',  ( -0.8090169943749506709, 0.5877852522924686962, 0.000000000000000000 ) ) ;
#14551=DIRECTION ( 'NONE',  ( -1.000000000000000000, 0.000000000000000000, 0.000000000000000000 ) ) ;
#14555=DIRECTION ( 'NONE',  ( 0.000000000000000000, 0.000000000000000000, 1.000000000000000000 ) ) ;
#14556=ADVANCED_FACE ( 'NONE', ( #56056 ), #38841, .F. ) ;
#14561=CARTESIAN_POINT ( 'NONE',  ( 26.69682282325795697, -59.27986298182186431, 170.0000000000000000 ) ) ;
#14563=ORIENTED_EDGE ( 'NONE', *, *, #51628, .F. ) ;
#14564=FACE_OUTER_BOUND ( 'NONE', #16300, .T. ) ;
#14565=LINE ( 'NONE', #69047, #37760 ) ;
#14573=CARTESIAN_POINT ( 'NONE',  ( 21.96921518829288900, -71.65937688154161833, 41.38025477438755928 ) ) ;
#14608=ORIENTED_EDGE ( 'NONE', *, *, #44447, .T. ) ;
#14616=EDGE_CURVE ( 'NONE', #44628, #27271, #2591, .T. ) ;
#14622=ORIENTED_EDGE ( 'NONE', *, *, #37702, .T. ) ;
#14625=CARTESIAN_POINT ( 'NONE',  ( -34.96012151086515019, 55.23134702900888016, 6.377659838150195247E-18 ) ) ;
#14651=VECTOR ( 'NONE', #24922, 1000.000000000000000 ) ;
#14653=CARTESIAN_POINT ( 'NONE',  ( -27.41072500102445275, 43.79450017564173692, 26.66469104408688295 ) ) ;
#14654=DIRECTION ( 'NONE',  ( -0.000000000000000000, -0.000000000000000000, -1.000000000000000000 ) ) ;
#14657=CARTESIAN_POINT ( 'NONE',  ( -44.00727179482576901, 47.83680621839559421, 170.0000000000000000 ) ) ;
#14663=VERTEX_POINT ( 'NONE', #65572 ) ;
#14666=ORIENTED_EDGE ( 'NONE', *, *, #29701, .F. ) ;
#14670=DIRECTION ( 'NONE',  ( -0.000000000000000000, -0.000000000000000000, -1.000000000000000000 ) ) ;
#14673=VERTEX_POINT ( 'NONE', #1542 ) ;
#14682=CARTESIAN_POINT ( 'NONE',  ( 30.12852347772543027, 58.62603998952763362, 133.5802547743875550 ) ) ;
#14685=EDGE_CURVE ( 'NONE', #65795, #26373, #34852, .T. ) ;
#14686=ORIENTED_EDGE ( 'NONE', *, *, #13114, .F. ) ;
#14689=ORIENTED_EDGE ( 'NONE', *, *, #25375, .T. ) ;
#14692=ADVANCED_FACE ( 'NONE', ( #23366 ), #20224, .T. ) ;
#14716=FACE_OUTER_BOUND ( 'NONE', #37553, .T. ) ;
#14725=CARTESIAN_POINT ( 'NONE',  ( -67.57266509268116295, -32.54128043381741975, 43.58025477438756212 ) ) ;
#14726=EDGE_LOOP ( 'NONE', ( #44020, #2351 ) ) ;
#14732=AXIS2_PLACEMENT_3D ( 'NONE', #38682, #34111, #7380 ) ;
#14737=VECTOR ( 'NONE', #49017, 1000.000000000000114 ) ;
#14744=AXIS2_PLACEMENT_3D ( 'NONE', #51554, #67390, #3019 ) ;
#14747=CARTESIAN_POINT ( 'NONE',  ( 29.69502258243432635, -57.82046033912835270, 170.0000000000000000 ) ) ;
#14760=VERTEX_POINT ( 'NONE', #54112 ) ;
#14771=ORIENTED_EDGE ( 'NONE', *, *, #36287, .T. ) ;
#14772=CARTESIAN_POINT ( 'NONE',  ( 24.34427655538949509, 5.688250960946272805, 0.000000000000000000 ) ) ;
#14773=ORIENTED_EDGE ( 'NONE', *, *, #56797, .F. ) ;
#14784=CARTESIAN_POINT ( 'NONE',  ( -15.47041015649658391, 73.39774458108210808, 133.5802547743875550 ) ) ;
#14786=ORIENTED_EDGE ( 'NONE', *, *, #69567, .T. ) ;
#14789=CARTESIAN_POINT ( 'NONE',  ( 0.000000000000000000, 0.000000000000000000, 41.38025477438755928 ) ) ;
#14794=VECTOR ( 'NONE', #8478, 999.9999999999998863 ) ;
#14796=CARTESIAN_POINT ( 'NONE',  ( -2.116120943112232755, 74.98056102853672655, 43.58025477438756212 ) ) ;
#14797=ORIENTED_EDGE ( 'NONE', *, *, #15378, .F. ) ;
#14816=ORIENTED_EDGE ( 'NONE', *, *, #13505, .T. ) ;
#14818=ORIENTED_EDGE ( 'NONE', *, *, #20575, .T. ) ;
#14820=DIRECTION ( 'NONE',  ( -0.6579387259397028176, -0.7530714660036196273, 5.102127870520020458E-18 ) ) ;
#14823=ORIENTED_EDGE ( 'NONE', *, *, #45127, .F. ) ;
#14833=AXIS2_PLACEMENT_3D ( 'NONE', #48532, #14820, #36294 ) ;
#14837=EDGE_CURVE ( 'NONE', #3230, #19006, #4655, .T. ) ;
#14842=FACE_OUTER_BOUND ( 'NONE', #32364, .T. ) ;
#14843=DIRECTION ( 'NONE',  ( 1.000000000000000000, 0.000000000000000000, 0.000000000000000000 ) ) ;
#14856=ORIENTED_EDGE ( 'NONE', *, *, #65352, .F. ) ;
#14873=CIRCLE ( 'NONE', #32802, 65.36598343705435354 ) ;
#14876=LINE ( 'NONE', #36696, #13274 ) ;
#14878=AXIS2_PLACEMENT_3D ( 'NONE', #10511, #5244, #48134 ) ;
#14879=CARTESIAN_POINT ( 'NONE',  ( 0.000000000000000000, 0.000000000000000000, 41.38025477438755928 ) ) ;
#14882=LINE ( 'NONE', #35663, #57635 ) ;
#14886=DIRECTION ( 'NONE',  ( -5.096990367256705246E-18, 2.289061013374613071E-19, -1.000000000000000000 ) ) ;
#14888=B_SPLINE_CURVE_WITH_KNOTS ( 'NONE', 3,
 ( #43489, #21346, #10789, #64964 ),
 .UNSPECIFIED., .F., .F.,
 ( 4, 4 ),
 ( 0.1259919275528357807, 0.1829744153748745217 ),
 .UNSPECIFIED. ) ;
#14891=CARTESIAN_POINT ( 'NONE',  ( 7.484861546145031852, 64.56761454192836425, 170.0000000000000000 ) ) ;
#14894=EDGE_CURVE ( 'NONE', #8769, #20715, #32623, .T. ) ;
#14895=VERTEX_POINT ( 'NONE', #69011 ) ;
#14902=CARTESIAN_POINT ( 'NONE',  ( 55.46196446482129261, -34.59309596431295830, 41.38025477438755928 ) ) ;
#14905=DIRECTION ( 'NONE',  ( -1.000000000000000000, 0.000000000000000000, 0.000000000000000000 ) ) ;
#14907=CARTESIAN_POINT ( 'NONE',  ( 16.83496171716143408, -55.85776949775602418, 27.58472315868180402 ) ) ;
#14910=EDGE_CURVE ( 'NONE', #46954, #37858, #33741, .T. ) ;
#14918=CARTESIAN_POINT ( 'NONE',  ( 8.942470798084043437, 23.47701018505912174, 0.000000000000000000 ) ) ;
#14920=DIRECTION ( 'NONE',  ( -0.6910626489868580968, -0.7227948638273978821, 0.000000000000000000 ) ) ;
#14921=EDGE_LOOP ( 'NONE', ( #29253, #33052, #2062, #64200 ) ) ;
#14922=CIRCLE ( 'NONE', #23920, 65.00000000000000000 ) ;
#14927=CARTESIAN_POINT ( 'NONE',  ( 61.91366885787816443, -28.42865614898931881, 41.38025477438755928 ) ) ;
#14936=ORIENTED_EDGE ( 'NONE', *, *, #1490, .F. ) ;
#14938=EDGE_CURVE ( 'NONE', #57624, #60956, #12630, .T. ) ;
#14945=ADVANCED_FACE ( 'NONE', ( #44635 ), #2423, .F. ) ;
#14951=VERTEX_POINT ( 'NONE', #13330 ) ;
#14952=LINE ( 'NONE', #36416, #57759 ) ;
#14956=CARTESIAN_POINT ( 'NONE',  ( -26.69131247781221106, -59.26697088777007849, 170.0000000000000000 ) ) ;
#14962=DIRECTION ( 'NONE',  ( -0.000000000000000000, -0.000000000000000000, -1.000000000000000000 ) ) ;
#14968=ORIENTED_EDGE ( 'NONE', *, *, #13583, .F. ) ;
#14977=ORIENTED_EDGE ( 'NONE', *, *, #34495, .T. ) ;
#14982=CARTESIAN_POINT ( 'NONE',  ( -24.39249304643438521, 60.24953346690454481, 170.0000000000000000 ) ) ;
#14985=VERTEX_POINT ( 'NONE', #45325 ) ;
#14986=EDGE_CURVE ( 'NONE', #2052, #925, #18948, .T. ) ;
#14990=CARTESIAN_POINT ( 'NONE',  ( 44.98017923036987042, -25.41829121023151927, 26.66469066592268433 ) ) ;
#14994=PLANE ( 'NONE',  #56190 ) ;
#14995=DIRECTION ( 'NONE',  ( 1.000000000000000000, 0.000000000000000000, 0.000000000000000000 ) ) ;
#14997=ORIENTED_EDGE ( 'NONE', *, *, #45127, .T. ) ;
#14999=DIRECTION ( 'NONE',  ( 0.000000000000000000, 1.000000000000000000, 0.000000000000000000 ) ) ;
#15001=ADVANCED_FACE ( 'NONE', ( #12984 ), #35471, .T. ) ;
#15006=DIRECTION ( 'NONE',  ( -2.086468734323010064E-16, 1.377265952997520258E-16, 1.000000000000000000 ) ) ;
#15017=DIRECTION ( 'NONE',  ( -0.9362348706397417564, 0.3513748240813305279, 0.000000000000000000 ) ) ;
#15020=VERTEX_POINT ( 'NONE', #61163 ) ;
#15030=AXIS2_PLACEMENT_3D ( 'NONE', #30448, #9691, #14276 ) ;
#15034=EDGE_CURVE ( 'NONE', #46531, #67474, #67486, .T. ) ;
#15060=CARTESIAN_POINT ( 'NONE',  ( 18.19409201603430404, 72.94804796678661774, 73.58025477438755502 ) ) ;
#15064=ORIENTED_EDGE ( 'NONE', *, *, #62023, .F. ) ;
#15068=LINE ( 'NONE', #36525, #59287 ) ;
#15075=EDGE_CURVE ( 'NONE', #34467, #29783, #63241, .T. ) ;
#15076=AXIS2_PLACEMENT_3D ( 'NONE', #6615, #38983, #60430 ) ;
#15086=ORIENTED_EDGE ( 'NONE', *, *, #8274, .T. ) ;
#15102=DIRECTION ( 'NONE',  ( -0.000000000000000000, -0.000000000000000000, -1.000000000000000000 ) ) ;
#15104=CARTESIAN_POINT ( 'NONE',  ( 32.67633866439968671, -58.08495054655669065, 34.48241823991042310 ) ) ;
#15105=CARTESIAN_POINT ( 'NONE',  ( 30.12852347772543027, -74.98256102853682137, 73.58025477438755502 ) ) ;
#15111=ORIENTED_EDGE ( 'NONE', *, *, #53344, .F. ) ;
#15114=LINE ( 'NONE', #20733, #68796 ) ;
#15120=EDGE_CURVE ( 'NONE', #64668, #56478, #21696, .T. ) ;
#15123=CARTESIAN_POINT ( 'NONE',  ( -13.60872002018478355, 65.24114715245431739, 34.48241795236666718 ) ) ;
#15137=LINE ( 'NONE', #21437, #39752 ) ;
#15141=CIRCLE ( 'NONE', #33114, 24.99999999999985434 ) ;
#15156=ADVANCED_FACE ( 'NONE', ( #27316 ), #15798, .T. ) ;
#15173=ADVANCED_FACE ( 'NONE', ( #17461 ), #65316, .T. ) ;
#15175=EDGE_CURVE ( 'NONE', #44661, #30106, #38452, .T. ) ;
#15176=VECTOR ( 'NONE', #34068, 1000.000000000000114 ) ;
#15177=ORIENTED_EDGE ( 'NONE', *, *, #61875, .F. ) ;
#15183=CIRCLE ( 'NONE', #2835, 65.00000000000000000 ) ;
#15204=VERTEX_POINT ( 'NONE', #238 ) ;
#15208=ORIENTED_EDGE ( 'NONE', *, *, #53745, .F. ) ;
#15219=ORIENTED_EDGE ( 'NONE', *, *, #23035, .T. ) ;
#15225=AXIS2_PLACEMENT_3D ( 'NONE', #47973, #21941, #20558 ) ;
#15226=CARTESIAN_POINT ( 'NONE',  ( 69.68177367721197868, -20.52767805628086961, 3.061616997868437868E-16 ) ) ;
#15227=ADVANCED_FACE ( 'NONE', ( #6570 ), #1294, .T. ) ;
#15232=CARTESIAN_POINT ( 'NONE',  ( -4.164416015345870470, 64.86646004871185767, 170.0000000000000000 ) ) ;
#15252=ORIENTED_EDGE ( 'NONE', *, *, #34475, .F. ) ;
#15276=AXIS2_PLACEMENT_3D ( 'NONE', #47728, #58290, #37183 ) ;
#15282=ORIENTED_EDGE ( 'NONE', *, *, #48100, .F. ) ;
#15287=VECTOR ( 'NONE', #41238, 1000.000000000000114 ) ;
#15292=AXIS2_PLACEMENT_3D ( 'NONE', #11289, #9929, #32760 ) ;
#15293=CARTESIAN_POINT ( 'NONE',  ( -30.60309003827974550, 68.41902945196812880, 41.38025477438755928 ) ) ;
#15295=ORIENTED_EDGE ( 'NONE', *, *, #55834, .T. ) ;
#15314=CARTESIAN_POINT ( 'NONE',  ( 60.40479419793764038, 24.00543350795394915, 170.0000000000000000 ) ) ;
#15317=FACE_OUTER_BOUND ( 'NONE', #29296, .T. ) ;
#15321=LINE ( 'NONE', #36784, #61328 ) ;
#15324=VECTOR ( 'NONE', #27825, 1000.000000000000000 ) ;
#15325=ORIENTED_EDGE ( 'NONE', *, *, #17731, .T. ) ;
#15331=DIRECTION ( 'NONE',  ( -0.000000000000000000, -0.000000000000000000, -1.000000000000000000 ) ) ;
#15334=ORIENTED_EDGE ( 'NONE', *, *, #26061, .F. ) ;
#15338=CARTESIAN_POINT ( 'NONE',  ( 35.54014968547571129, -66.04466488925490353, 0.000000000000000000 ) ) ;
#15346=CARTESIAN_POINT ( 'NONE',  ( 0.000000000000000000, 0.000000000000000000, 40.00000000000003553 ) ) ;
#15351=CARTESIAN_POINT ( 'NONE',  ( 75.00000000000000000, 0.000000000000000000, 43.58025477438756212 ) ) ;
#15353=LINE ( 'NONE', #69145, #48548 ) ;
#15355=ORIENTED_EDGE ( 'NONE', *, *, #4297, .F. ) ;
#15370=ORIENTED_EDGE ( 'NONE', *, *, #36931, .T. ) ;
#15378=EDGE_CURVE ( 'NONE', #67017, #20457, #66721, .T. ) ;
#15392=LINE ( 'NONE', #21017, #21946 ) ;
#15398=ORIENTED_EDGE ( 'NONE', *, *, #54962, .T. ) ;
#15399=DIRECTION ( 'NONE',  ( -2.213730317917169031E-18, 4.596858371395784539E-18, -1.000000000000000000 ) ) ;
#15402=CARTESIAN_POINT ( 'NONE',  ( 0.000000000000000000, 0.000000000000000000, 170.0000000000000000 ) ) ;
#15408=ADVANCED_FACE ( 'NONE', ( #25191 ), #46973, .T. ) ;
#15410=EDGE_CURVE ( 'NONE', #3016, #67765, #57876, .T. ) ;
#15425=CARTESIAN_POINT ( 'NONE',  ( -15.47041015649555185, -73.39774458108232125, 170.0000000000000000 ) ) ;
#15447=ORIENTED_EDGE ( 'NONE', *, *, #43574, .T. ) ;
#15449=DIRECTION ( 'NONE',  ( 1.000000000000000000, 0.000000000000000000, 0.000000000000000000 ) ) ;
#15450=FACE_OUTER_BOUND ( 'NONE', #24221, .T. ) ;
#15451=ORIENTED_EDGE ( 'NONE', *, *, #17630, .F. ) ;
#15456=CARTESIAN_POINT ( 'NONE',  ( 21.27121078971613244, 61.42097029141973508, 40.00000000000003553 ) ) ;
#15466=AXIS2_PLACEMENT_3D ( 'NONE', #59966, #12852, #23745 ) ;
#15468=CARTESIAN_POINT ( 'NONE',  ( -84.49322488516129681, 0.000000000000000000, 43.58025477438756212 ) ) ;
#15473=EDGE_CURVE ( 'NONE', #36451, #30352, #42383, .T. ) ;
#15481=DIRECTION ( 'NONE',  ( 1.000000000000000000, 0.000000000000000000, 0.000000000000000000 ) ) ;
#15484=ORIENTED_EDGE ( 'NONE', *, *, #9879, .T. ) ;
#15486=CARTESIAN_POINT ( 'NONE',  ( -3.566018980795016002, -51.54211481249757298, 26.66469104408689006 ) ) ;
#15490=ADVANCED_FACE ( 'NONE', ( #31829 ), #16339, .T. ) ;
#15497=CARTESIAN_POINT ( 'NONE',  ( 0.000000000000000000, 0.000000000000000000, 41.38025477438755928 ) ) ;
#15500=EDGE_CURVE ( 'NONE', #7966, #63543, #5439, .T. ) ;
#15511=DIRECTION ( 'NONE',  ( -0.5128992774058949156, -0.8584487936018728726, 0.000000000000000000 ) ) ;
#15513=FACE_OUTER_BOUND ( 'NONE', #53265, .T. ) ;
#15517=EDGE_LOOP ( 'NONE', ( #27573, #40788, #27224, #60473 ) ) ;
#15525=ORIENTED_EDGE ( 'NONE', *, *, #56633, .F. ) ;
#15526=ORIENTED_EDGE ( 'NONE', *, *, #46454, .F. ) ;
#15529=VECTOR ( 'NONE', #17071, 1000.000000000000000 ) ;
#15535=LINE ( 'NONE', #52798, #3345 ) ;
#15537=B_SPLINE_CURVE_WITH_KNOTS ( 'NONE', 3,
 ( #52329, #51983, #57952, #47382, #9773, #4153 ),
 .UNSPECIFIED., .F., .F.,
 ( 4, 2, 4 ),
 ( 0.03218936187311347008, 0.06469833704501400107, 0.09720731221691453205 ),
 .UNSPECIFIED. ) ;
#15540=ORIENTED_EDGE ( 'NONE', *, *, #60899, .F. ) ;
#15549=EDGE_CURVE ( 'NONE', #23937, #16594, #28639, .T. ) ;
#15553=EDGE_LOOP ( 'NONE', ( #22920, #27993, #45447, #2675, #2827, #58539, #43391, #13034, #69482 ) ) ;
#15554=EDGE_CURVE ( 'NONE', #56212, #66914, #6829, .T. ) ;
#15561=DIRECTION ( 'NONE',  ( 1.000000000000000000, 0.000000000000000000, 0.000000000000000000 ) ) ;
#15567=CARTESIAN_POINT ( 'NONE',  ( -11.97857120004195330, -31.20571949911692045, 6.893342933292192498 ) ) ;
#15570=EDGE_CURVE ( 'NONE', #8876, #17506, #29318, .T. ) ;
#15574=DIRECTION ( 'NONE',  ( 0.9909497617679351444, -0.1342332658176522420, -2.292031753669949326E-16 ) ) ;
#15576=AXIS2_PLACEMENT_3D ( 'NONE', #22426, #27344, #60411 ) ;
#15583=LINE ( 'NONE', #14200, #2030 ) ;
#15597=EDGE_LOOP ( 'NONE', ( #26924, #53780, #22293, #10301 ) ) ;
#15601=VERTEX_POINT ( 'NONE', #60267 ) ;
#15611=DIRECTION ( 'NONE',  ( 0.000000000000000000, 0.000000000000000000, 1.000000000000000000 ) ) ;
#15612=FACE_OUTER_BOUND ( 'NONE', #10998, .T. ) ;
#15618=AXIS2_PLACEMENT_3D ( 'NONE', #45972, #51939, #19231 ) ;
#15628=DIRECTION ( 'NONE',  ( 1.000000000000000000, 0.000000000000000000, -0.000000000000000000 ) ) ;
#15632=CARTESIAN_POINT ( 'NONE',  ( 60.82895951008336510, 30.68107831874607072, 170.0000000000000000 ) ) ;
#15637=ORIENTED_EDGE ( 'NONE', *, *, #44198, .T. ) ;
#15646=VERTEX_POINT ( 'NONE', #40205 ) ;
#15653=EDGE_CURVE ( 'NONE', #66979, #59078, #16641, .T. ) ;
#15655=CIRCLE ( 'NONE', #39266, 25.12245591505646303 ) ;
#15657=ORIENTED_EDGE ( 'NONE', *, *, #30028, .F. ) ;
#15666=DIRECTION ( 'NONE',  ( -0.3090169943749582759, 0.9510565162951499785, 0.000000000000000000 ) ) ;
#15668=AXIS2_PLACEMENT_3D ( 'NONE', #63807, #32479, #53912 ) ;
#15672=CARTESIAN_POINT ( 'NONE',  ( 0.000000000000000000, 0.000000000000000000, 170.0000000000000000 ) ) ;
#15681=ORIENTED_EDGE ( 'NONE', *, *, #51043, .F. ) ;
#15694=ORIENTED_EDGE ( 'NONE', *, *, #53873, .T. ) ;
#15696=CARTESIAN_POINT ( 'NONE',  ( 74.62299871641508275, -5.461138973197949831, 170.0000000000000000 ) ) ;
#15709=DIRECTION ( 'NONE',  ( 0.9839295885986321100, -0.1785568947986229116, 0.000000000000000000 ) ) ;
#15714=ORIENTED_EDGE ( 'NONE', *, *, #5238, .T. ) ;
#15715=EDGE_CURVE ( 'NONE', #53047, #58120, #68650, .T. ) ;
#15725=DIRECTION ( 'NONE',  ( 1.000000000000000000, 0.000000000000000000, -0.000000000000000000 ) ) ;
#15730=CARTESIAN_POINT ( 'NONE',  ( 56.74421265833604622, -32.44697398030825042, 43.58025477438756212 ) ) ;
#15737=CIRCLE ( 'NONE', #8972, 65.00000000000000000 ) ;
#15741=ORIENTED_EDGE ( 'NONE', *, *, #29471, .F. ) ;
#15745=DIRECTION ( 'NONE',  ( -0.000000000000000000, -0.000000000000000000, -1.000000000000000000 ) ) ;
#15752=AXIS2_PLACEMENT_3D ( 'NONE', #44450, #11738, #65937 ) ;
#15755=B_SPLINE_CURVE_WITH_KNOTS ( 'NONE', 3,
 ( #65122, #49979, #12352, #33115, #22903, #39097 ),
 .UNSPECIFIED., .F., .F.,
 ( 4, 2, 4 ),
 ( 1.095770181115536239E-06, 0.03239442681617710901, 0.06478775786217311206 ),
 .UNSPECIFIED. ) ;
#15763=CARTESIAN_POINT ( 'NONE',  ( 0.000000000000000000, 0.000000000000000000, 41.38025477438755928 ) ) ;
#15770=AXIS2_PLACEMENT_3D ( 'NONE', #62506, #25224, #68794 ) ;
#15774=ORIENTED_EDGE ( 'NONE', *, *, #66795, .T. ) ;
#15779=FACE_OUTER_BOUND ( 'NONE', #52724, .T. ) ;
#15782=VECTOR ( 'NONE', #34771, 1000.000000000000000 ) ;
#15786=DIRECTION ( 'NONE',  ( -0.000000000000000000, 0.000000000000000000, -1.000000000000000000 ) ) ;
#15793=EDGE_LOOP ( 'NONE', ( #51754, #1004, #68092, #37952, #54329, #20871, #8846, #23753, #53326 ) ) ;
#15798=CONICAL_SURFACE ( 'NONE', #48355, 65.00000000000000000, 0.7853981633974497223 ) ;
#15800=DIRECTION ( 'NONE',  ( -1.000000000000000000, 0.000000000000000000, 0.000000000000000000 ) ) ;
#15805=CARTESIAN_POINT ( 'NONE',  ( 30.58844157136472575, 28.38418561969873721, 13.79046412417415191 ) ) ;
#15807=CARTESIAN_POINT ( 'NONE',  ( -50.92620509423088038, 55.07344309828769724, 170.0000000000000000 ) ) ;
#15817=EDGE_CURVE ( 'NONE', #25239, #58815, #28160, .T. ) ;
#15820=ORIENTED_EDGE ( 'NONE', *, *, #38902, .F. ) ;
#15823=ORIENTED_EDGE ( 'NONE', *, *, #23621, .F. ) ;
#15826=DIRECTION ( 'NONE',  ( 0.000000000000000000, 0.000000000000000000, 1.000000000000000000 ) ) ;
#15832=ORIENTED_EDGE ( 'NONE', *, *, #37546, .T. ) ;
#15843=ORIENTED_EDGE ( 'NONE', *, *, #5071, .T. ) ;
#15849=AXIS2_PLACEMENT_3D ( 'NONE', #21494, #11996, #10943 ) ;
#15854=ORIENTED_EDGE ( 'NONE', *, *, #19129, .F. ) ;
#15856=VERTEX_POINT ( 'NONE', #32752 ) ;
#15857=EDGE_CURVE ( 'NONE', #42885, #31341, #64412, .T. ) ;
#15863=ADVANCED_FACE ( 'NONE', ( #11282 ), #48908, .T. ) ;
#15867=CARTESIAN_POINT ( 'NONE',  ( -52.73319225379940178, 53.34578647582053179, 43.58025477438756923 ) ) ;
#15868=DIRECTION ( 'NONE',  ( 1.000000000000000000, 0.000000000000000000, -0.000000000000000000 ) ) ;
#15869=DIRECTION ( 'NONE',  ( 1.000000000000000000, 0.000000000000000000, -0.000000000000000000 ) ) ;
#15870=ADVANCED_FACE ( 'NONE', ( #54892 ), #6004, .F. ) ;
#15872=CARTESIAN_POINT ( 'NONE',  ( -4.337405327940998312, -24.62086340933521456, 0.000000000000000000 ) ) ;
#15882=FACE_OUTER_BOUND ( 'NONE', #32888, .T. ) ;
#15888=CARTESIAN_POINT ( 'NONE',  ( -17.90772993695114934, 72.84144224619130625, 133.5802547743875550 ) ) ;
#15892=ORIENTED_EDGE ( 'NONE', *, *, #16335, .T. ) ;
#15894=ORIENTED_EDGE ( 'NONE', *, *, #52263, .T. ) ;
#15897=FACE_OUTER_BOUND ( 'NONE', #37275, .T. ) ;
#15900=AXIS2_PLACEMENT_3D ( 'NONE', #41262, #26461, #68341 ) ;
#15901=EDGE_CURVE ( 'NONE', #6977, #38689, #707, .T. ) ;
#15905=LINE ( 'NONE', #18859, #18458 ) ;
#15914=VERTEX_POINT ( 'NONE', #67466 ) ;
#15939=EDGE_LOOP ( 'NONE', ( #1048, #19635, #15854, #49583 ) ) ;
#15954=DIRECTION ( 'NONE',  ( 0.6234898018587318180, 0.7818314824680311359, 0.000000000000000000 ) ) ;
#15963=ORIENTED_EDGE ( 'NONE', *, *, #45998, .F. ) ;
#15966=DIRECTION ( 'NONE',  ( 0.6234898018587431423, -0.7818314824680221431, 0.000000000000000000 ) ) ;
#15974=ORIENTED_EDGE ( 'NONE', *, *, #42075, .T. ) ;
#15980=DIRECTION ( 'NONE',  ( 0.4738686624730094610, -0.8805955318567321166, 0.000000000000000000 ) ) ;
#16000=CARTESIAN_POINT ( 'NONE',  ( 36.64089410029661309, -65.45232906116366678, 170.0000000000000000 ) ) ;
#16025=AXIS2_PLACEMENT_3D ( 'NONE', #15346, #59272, #37831 ) ;
#16029=CARTESIAN_POINT ( 'NONE',  ( -46.06722295615789875, 46.37372919877053334, 3.125053320693552861E-16 ) ) ;
#16046=DIRECTION ( 'NONE',  ( -1.000000000000000000, 0.000000000000000000, 0.000000000000000000 ) ) ;
#16056=DIRECTION ( 'NONE',  ( -0.2660368455666687892, -0.9639628606958550172, 2.500042656554809847E-16 ) ) ;
#16069=CIRCLE ( 'NONE', #13973, 65.36598343705435354 ) ;
#16078=FACE_OUTER_BOUND ( 'NONE', #65140, .T. ) ;
#16083=AXIS2_PLACEMENT_3D ( 'NONE', #1692, #32316, #1341 ) ;
#16088=VECTOR ( 'NONE', #58732, 1000.000000000000000 ) ;
#16089=ORIENTED_EDGE ( 'NONE', *, *, #47379, .T. ) ;
#16092=CARTESIAN_POINT ( 'NONE',  ( -9.964117946888961797, -64.24592483216726180, 43.58025477438756923 ) ) ;
#16104=ADVANCED_FACE ( 'NONE', ( #33985 ), #54367, .T. ) ;
#16110=EDGE_CURVE ( 'NONE', #25506, #25227, #28710, .T. ) ;
#16117=VECTOR ( 'NONE', #30728, 1000.000000000000000 ) ;
#16119=DIRECTION ( 'NONE',  ( -0.6579387259397027066, -0.7530714660036195163, 0.000000000000000000 ) ) ;
#16140=PLANE ( 'NONE',  #30203 ) ;
#16144=CARTESIAN_POINT ( 'NONE',  ( -18.89790202299119315, -62.20684691518632548, 41.38025477438755928 ) ) ;
#16156=DIRECTION ( 'NONE',  ( 1.000000000000000000, 0.000000000000000000, 0.000000000000000000 ) ) ;
#16161=CARTESIAN_POINT ( 'NONE',  ( -2.967675213622137598, -38.21895566658998433, 13.32819397642332149 ) ) ;
#16163=VERTEX_POINT ( 'NONE', #8295 ) ;
#16166=CARTESIAN_POINT ( 'NONE',  ( -24.98026281234599821, -0.9932118737290694943, 0.000000000000000000 ) ) ;
#16171=EDGE_LOOP ( 'NONE', ( #24794, #28283, #42185, #33426 ) ) ;
#16179=DIRECTION ( 'NONE',  ( -1.000000000000000000, 0.000000000000000000, 0.000000000000000000 ) ) ;
#16180=AXIS2_PLACEMENT_3D ( 'NONE', #351, #21808, #60841 ) ;
#16181=EDGE_CURVE ( 'NONE', #58719, #59923, #3697, .T. ) ;
#16184=CARTESIAN_POINT ( 'NONE',  ( 26.69682282325711142, 59.27986298182224800, 41.38025477438755928 ) ) ;
#16189=AXIS2_PLACEMENT_3D ( 'NONE', #66087, #61139, #17519 ) ;
#16197=EDGE_LOOP ( 'NONE', ( #4382, #31363, #62284, #2266 ) ) ;
#16201=ORIENTED_EDGE ( 'NONE', *, *, #18981, .F. ) ;
#16203=ADVANCED_FACE ( 'NONE', ( #67052 ), #51207, .F. ) ;
#16211=CARTESIAN_POINT ( 'NONE',  ( -62.97854483871577713, 16.08424353203677271, 170.0000000000000000 ) ) ;
#16219=CARTESIAN_POINT ( 'NONE',  ( 64.16679220703380793, -10.37413986118096254, 40.00000000000003553 ) ) ;
#16227=DIRECTION ( 'NONE',  ( -1.000000000000000000, 0.000000000000000000, 0.000000000000000000 ) ) ;
#16228=AXIS2_PLACEMENT_3D ( 'NONE', #6654, #38666, #23885 ) ;
#16232=ORIENTED_EDGE ( 'NONE', *, *, #3985, .T. ) ;
#16237=ORIENTED_EDGE ( 'NONE', *, *, #39393, .F. ) ;
#16241=DIRECTION ( 'NONE',  ( -0.9909497617679332571, -0.1342332658176667581, 5.102127870520021228E-18 ) ) ;
#16246=DIRECTION ( 'NONE',  ( 0.000000000000000000, 0.000000000000000000, 1.000000000000000000 ) ) ;
#16252=CARTESIAN_POINT ( 'NONE',  ( 44.01696072965949469, 47.84694004974210912, 41.38025477438755928 ) ) ;
#16265=DIRECTION ( 'NONE',  ( -0.000000000000000000, -0.000000000000000000, -1.000000000000000000 ) ) ;
#16266=EDGE_CURVE ( 'NONE', #44661, #14985, #54033, .T. ) ;
#16284=ORIENTED_EDGE ( 'NONE', *, *, #16266, .T. ) ;
#16285=ORIENTED_EDGE ( 'NONE', *, *, #37302, .T. ) ;
#16289=EDGE_CURVE ( 'NONE', #5114, #4283, #38120, .T. ) ;
#16295=ADVANCED_FACE ( 'NONE', ( #17728 ), #38474, .T. ) ;
#16299=DIRECTION ( 'NONE',  ( -1.000000000000000000, 0.000000000000000000, 0.000000000000000000 ) ) ;
#16300=EDGE_LOOP ( 'NONE', ( #49438, #14968, #24865, #35210 ) ) ;
#16325=CARTESIAN_POINT ( 'NONE',  ( 36.85262215550149278, -53.56030941157680303, 43.58025477438756923 ) ) ;
#16327=VECTOR ( 'NONE', #50802, 1000.000000000000114 ) ;
#16328=DIRECTION ( 'NONE',  ( 0.3090169943749446757, 0.9510565162951544194, 0.000000000000000000 ) ) ;
#16335=EDGE_CURVE ( 'NONE', #9782, #27522, #7168, .T. ) ;
#16339=PLANE ( 'NONE',  #16892 ) ;
#16346=DIRECTION ( 'NONE',  ( -0.000000000000000000, -0.000000000000000000, -1.000000000000000000 ) ) ;
#16365=CARTESIAN_POINT ( 'NONE',  ( -36.59702049363711041, -36.46867397787282528, 26.66469104408689006 ) ) ;
#16368=ORIENTED_EDGE ( 'NONE', *, *, #11596, .F. ) ;
#16369=DIRECTION ( 'NONE',  ( -0.000000000000000000, -0.000000000000000000, -1.000000000000000000 ) ) ;
#16376=EDGE_CURVE ( 'NONE', #22589, #12081, #58562, .T. ) ;
#16388=DIRECTION ( 'NONE',  ( 0.000000000000000000, 1.000000000000000000, 0.000000000000000000 ) ) ;
#16402=ORIENTED_EDGE ( 'NONE', *, *, #47134, .T. ) ;
#16406=FACE_OUTER_BOUND ( 'NONE', #14921, .T. ) ;
#16427=DIRECTION ( 'NONE',  ( -0.9909497617679352555, 0.1342332658176522697, 2.500042656554811326E-16 ) ) ;
#16432=LINE ( 'NONE', #42803, #43181 ) ;
#16439=EDGE_CURVE ( 'NONE', #57672, #37468, #62717, .T. ) ;
#16456=DIRECTION ( 'NONE',  ( -1.000000000000000000, 0.000000000000000000, 0.000000000000000000 ) ) ;
#16462=DIRECTION ( 'NONE',  ( 1.000000000000000000, 0.000000000000000000, 0.000000000000000000 ) ) ;
#16472=ORIENTED_EDGE ( 'NONE', *, *, #21285, .T. ) ;
#16486=ADVANCED_FACE ( 'NONE', ( #35978 ), #63407, .T. ) ;
#16491=DIRECTION ( 'NONE',  ( 0.8584487936018728726, -0.5128992774058949156, 0.000000000000000000 ) ) ;
#16492=DIRECTION ( 'NONE',  ( -1.000000000000000000, 0.000000000000000000, 0.000000000000000000 ) ) ;
#16497=ADVANCED_FACE ( 'NONE', ( #15897 ), #56323, .T. ) ;
#16498=ORIENTED_EDGE ( 'NONE', *, *, #33549, .F. ) ;
#16504=ADVANCED_FACE ( 'NONE', ( #9593 ), #55216, .T. ) ;
#16509=ORIENTED_EDGE ( 'NONE', *, *, #26061, .T. ) ;
#16521=VECTOR ( 'NONE', #10457, 1000.000000000000227 ) ;
#16523=ORIENTED_EDGE ( 'NONE', *, *, #65920, .T. ) ;
#16525=VERTEX_POINT ( 'NONE', #49275 ) ;
#16527=EDGE_LOOP ( 'NONE', ( #47798, #55734, #14091, #45753 ) ) ;
#16533=CARTESIAN_POINT ( 'NONE',  ( -55.15976438495108169, -34.41253982194112382, 170.0000000000000000 ) ) ;
#16537=ORIENTED_EDGE ( 'NONE', *, *, #5789, .T. ) ;
#16542=LINE ( 'NONE', #63703, #26524 ) ;
#16548=ORIENTED_EDGE ( 'NONE', *, *, #8179, .T. ) ;
#16553=ORIENTED_EDGE ( 'NONE', *, *, #34877, .T. ) ;
#16556=DIRECTION ( 'NONE',  ( -2.497525279955785470E-16, 1.121639896553560265E-17, 1.000000000000000000 ) ) ;
#16565=ORIENTED_EDGE ( 'NONE', *, *, #44150, .T. ) ;
#16570=CYLINDRICAL_SURFACE ( 'NONE', #41132, 65.00000000000000000 ) ;
#16572=CARTESIAN_POINT ( 'NONE',  ( -3.364862276288897558, 74.92447999059858432, 43.58025477438756212 ) ) ;
#16574=CARTESIAN_POINT ( 'NONE',  ( 0.000000000000000000, 0.000000000000000000, 0.000000000000000000 ) ) ;
#16594=VERTEX_POINT ( 'NONE', #18328 ) ;
#16611=ORIENTED_EDGE ( 'NONE', *, *, #14530, .T. ) ;
#16616=CARTESIAN_POINT ( 'NONE',  ( -16.35146342289110422, 18.91109843266242052, 0.000000000000000000 ) ) ;
#16621=CARTESIAN_POINT ( 'NONE',  ( 0.000000000000000000, 0.000000000000000000, 0.000000000000000000 ) ) ;
#16626=CARTESIAN_POINT ( 'NONE',  ( 0.000000000000000000, 0.000000000000000000, 40.00000000000003553 ) ) ;
#16637=VERTEX_POINT ( 'NONE', #56306 ) ;
#16639=EDGE_CURVE ( 'NONE', #29783, #35065, #49988, .T. ) ;
#16641=B_SPLINE_CURVE_WITH_KNOTS ( 'NONE', 3,
 ( #50412, #35270, #29994, #45824, #18059, #56372 ),
 .UNSPECIFIED., .F., .F.,
 ( 4, 2, 4 ),
 ( 0.03218933845493736345, 0.06469832000440858821, 0.09720730155387982685 ),
 .UNSPECIFIED. ) ;
#16644=CARTESIAN_POINT ( 'NONE',  ( 26.12852347772543737, 100.0000000000000000, 77.58025477438755502 ) ) ;
#16645=DIRECTION ( 'NONE',  ( -0.9009688679024155933, -0.4338837391175656699, 0.000000000000000000 ) ) ;
#16653=EDGE_CURVE ( 'NONE', #42599, #2074, #35202, .T. ) ;
#16660=B_SPLINE_CURVE_WITH_KNOTS ( 'NONE', 3,
 ( #10361, #55623, #28909, #17289, #33136, #37103 ),
 .UNSPECIFIED., .F., .F.,
 ( 4, 2, 4 ),
 ( 1.095770181109144105E-06, 0.03239442681617710207, 0.06478775786217309818 ),
 .UNSPECIFIED. ) ;
#16672=CARTESIAN_POINT ( 'NONE',  ( 24.36509522348982060, 70.94296747916789059, 170.0000000000000000 ) ) ;
#16675=ORIENTED_EDGE ( 'NONE', *, *, #13355, .F. ) ;
#16685=ORIENTED_EDGE ( 'NONE', *, *, #59213, .T. ) ;
#16689=DIRECTION ( 'NONE',  ( -3.687791819402489765E-18, 3.525890001671242775E-18, -1.000000000000000000 ) ) ;
#16690=CYLINDRICAL_SURFACE ( 'NONE', #563, 65.36598343705435354 ) ;
#16692=CARTESIAN_POINT ( 'NONE',  ( 24.36509522349078338, -70.94296747916756374, 170.0000000000000000 ) ) ;
#16700=CARTESIAN_POINT ( 'NONE',  ( -84.49322488516129681, 0.000000000000000000, 43.58025477438756212 ) ) ;
#16705=ORIENTED_EDGE ( 'NONE', *, *, #56859, .T. ) ;
#16708=CARTESIAN_POINT ( 'NONE',  ( 0.000000000000000000, 0.000000000000000000, 170.0000000000000000 ) ) ;
#16715=AXIS2_PLACEMENT_3D ( 'NONE', #64722, #720, #53109 ) ;
#16721=EDGE_CURVE ( 'NONE', #62736, #36820, #9509, .T. ) ;
#16725=DIRECTION ( 'NONE',  ( -1.000000000000000000, 0.000000000000000000, 0.000000000000000000 ) ) ;
#16726=ORIENTED_EDGE ( 'NONE', *, *, #57514, .T. ) ;
#16732=EDGE_CURVE ( 'NONE', #57123, #20617, #4569, .T. ) ;
#16741=ORIENTED_EDGE ( 'NONE', *, *, #37471, .T. ) ;
#16743=EDGE_CURVE ( 'NONE', #54393, #33166, #63104, .T. ) ;
#16747=LINE ( 'NONE', #17443, #12129 ) ;
#16749=DIRECTION ( 'NONE',  ( 0.3090169943749582759, -0.9510565162951499785, 0.000000000000000000 ) ) ;
#16757=ORIENTED_EDGE ( 'NONE', *, *, #32356, .T. ) ;
#16768=CARTESIAN_POINT ( 'NONE',  ( 14.66690460840479027, 20.39656099473415551, 3.061616997868437868E-16 ) ) ;
#16778=VERTEX_POINT ( 'NONE', #1026 ) ;
#16785=CARTESIAN_POINT ( 'NONE',  ( 0.000000000000000000, 0.000000000000000000, 41.38025477438755928 ) ) ;
#16786=ORIENTED_EDGE ( 'NONE', *, *, #55022, .T. ) ;
#16793=CARTESIAN_POINT ( 'NONE',  ( 30.12852347772543027, 100.0000000000000000, 73.58025477438755502 ) ) ;
#16795=LINE ( 'NONE', #54417, #56618 ) ;
#16796=VECTOR ( 'NONE', #31636, 1000.000000000000114 ) ;
#16797=PLANE ( 'NONE',  #66318 ) ;
#16812=VERTEX_POINT ( 'NONE', #49538 ) ;
#16820=EDGE_CURVE ( 'NONE', #37239, #33479, #49187, .T. ) ;
#16823=VECTOR ( 'NONE', #42945, 1000.000000000000000 ) ;
#16826=CARTESIAN_POINT ( 'NONE',  ( 0.000000000000000000, 0.000000000000000000, 41.38025477438755928 ) ) ;
#16828=CARTESIAN_POINT ( 'NONE',  ( -58.33959211650994092, -29.48226216511403308, 3.125053320693560257E-16 ) ) ;
#16840=PLANE ( 'NONE',  #54513 ) ;
#16841=CARTESIAN_POINT ( 'NONE',  ( 29.69502258243350923, 57.82046033912877903, 133.5802547743875550 ) ) ;
#16851=LINE ( 'NONE', #59752, #54425 ) ;
#16854=VERTEX_POINT ( 'NONE', #16841 ) ;
#16866=FACE_OUTER_BOUND ( 'NONE', #15939, .T. ) ;
#16875=DIRECTION ( 'NONE',  ( 0.000000000000000000, 0.000000000000000000, 1.000000000000000000 ) ) ;
#16881=VERTEX_POINT ( 'NONE', #38301 ) ;
#16888=EDGE_CURVE ( 'NONE', #17738, #11802, #18945, .T. ) ;
#16890=ORIENTED_EDGE ( 'NONE', *, *, #24481, .F. ) ;
#16892=AXIS2_PLACEMENT_3D ( 'NONE', #27233, #43749, #21272 ) ;
#16896=FACE_OUTER_BOUND ( 'NONE', #57231, .T. ) ;
#16897=CARTESIAN_POINT ( 'NONE',  ( 0.000000000000000000, 0.000000000000000000, 41.38025477438755928 ) ) ;
#16900=DIRECTION ( 'NONE',  ( -0.000000000000000000, -0.000000000000000000, 1.000000000000000000 ) ) ;
#16914=CARTESIAN_POINT ( 'NONE',  ( 34.43940527065381474, 66.63700071734669450, 43.58025477438756923 ) ) ;
#16928=DIRECTION ( 'NONE',  ( 0.1342332658176667304, -0.9909497617679331460, 0.000000000000000000 ) ) ;
#16933=CARTESIAN_POINT ( 'NONE',  ( -3.120068547127581748, 41.61225688647869703, 13.79046412284830048 ) ) ;
#16940=AXIS2_PLACEMENT_3D ( 'NONE', #60644, #12459, #12117 ) ;
#16942=VERTEX_POINT ( 'NONE', #23186 ) ;
#16957=CARTESIAN_POINT ( 'NONE',  ( 19.00668540189185407, 62.54164772954719353, 3.125053320693570118E-16 ) ) ;
#16962=ORIENTED_EDGE ( 'NONE', *, *, #25375, .F. ) ;
#16973=PLANE ( 'NONE',  #58291 ) ;
#16976=FACE_OUTER_BOUND ( 'NONE', #38309, .T. ) ;
#16999=ORIENTED_EDGE ( 'NONE', *, *, #5622, .T. ) ;
#17000=DIRECTION ( 'NONE',  ( -0.04486483035050446017, -0.9989930665413151445, 0.000000000000000000 ) ) ;
#17001=ORIENTED_EDGE ( 'NONE', *, *, #56949, .F. ) ;
#17002=ORIENTED_EDGE ( 'NONE', *, *, #3642, .F. ) ;
#17006=DIRECTION ( 'NONE',  ( 0.3090169943749582759, -0.9510565162951499785, 0.000000000000000000 ) ) ;
#17010=EDGE_LOOP ( 'NONE', ( #23143, #4788, #41545, #54607 ) ) ;
#17011=ORIENTED_EDGE ( 'NONE', *, *, #32636, .F. ) ;
#17018=CARTESIAN_POINT ( 'NONE',  ( -24.39249304643438521, 60.24953346690454481, 170.0000000000000000 ) ) ;
#17019=ORIENTED_EDGE ( 'NONE', *, *, #29254, .T. ) ;
#17029=CARTESIAN_POINT ( 'NONE',  ( 0.000000000000000000, 0.000000000000000000, 41.38025477438755928 ) ) ;
#17036=FACE_OUTER_BOUND ( 'NONE', #55740, .T. ) ;
#17043=PLANE ( 'NONE',  #54015 ) ;
#17046=ORIENTED_EDGE ( 'NONE', *, *, #62766, .T. ) ;
#17048=CARTESIAN_POINT ( 'NONE',  ( 0.000000000000000000, 0.000000000000000000, 0.000000000000000000 ) ) ;
#17057=ORIENTED_EDGE ( 'NONE', *, *, #46761, .F. ) ;
#17059=DIRECTION ( 'NONE',  ( 0.000000000000000000, -2.500042656554809847E-16, 1.000000000000000000 ) ) ;
#17060=EDGE_CURVE ( 'NONE', #43922, #58687, #3457, .T. ) ;
#17066=VECTOR ( 'NONE', #7659, 1000.000000000000114 ) ;
#17069=EDGE_LOOP ( 'NONE', ( #68928, #22191, #44318, #37748 ) ) ;
#17071=DIRECTION ( 'NONE',  ( 0.000000000000000000, 0.000000000000000000, -1.000000000000000000 ) ) ;
#17072=CARTESIAN_POINT ( 'NONE',  ( 21.27121078971695312, -61.42097029141944375, 170.0000000000000000 ) ) ;
#17073=DIRECTION ( 'NONE',  ( -0.000000000000000000, 0.000000000000000000, -1.000000000000000000 ) ) ;
#17077=CARTESIAN_POINT ( 'NONE',  ( 65.35403040894466642, 1.250000000000021982, 43.58025477438756212 ) ) ;
#17079=LINE ( 'NONE', #49787, #13455 ) ;
#17087=FACE_OUTER_BOUND ( 'NONE', #28040, .T. ) ;
#17094=CARTESIAN_POINT ( 'NONE',  ( 0.000000000000000000, 0.000000000000000000, 41.41421356237313489 ) ) ;
#17099=CARTESIAN_POINT ( 'NONE',  ( -19.46539569203812903, -15.68752276659308365, 0.000000000000000000 ) ) ;
#17102=CARTESIAN_POINT ( 'NONE',  ( 1.667562369267789890, -64.99262834925670518, 170.0000000000000000 ) ) ;
#17105=CARTESIAN_POINT ( 'NONE',  ( 64.08056813503714011, -12.89932471814424630, 41.38025477438755928 ) ) ;
#17106=ADVANCED_FACE ( 'NONE', ( #30536 ), #63581, .T. ) ;
#17114=EDGE_CURVE ( 'NONE', #12845, #19095, #20318, .T. ) ;
#17116=VECTOR ( 'NONE', #61963, 1000.000000000000000 ) ;
#17123=VERTEX_POINT ( 'NONE', #10111 ) ;
#17124=CARTESIAN_POINT ( 'NONE',  ( 45.82394788922869822, -46.11928342727429708, 170.0000000000000000 ) ) ;
#17126=CARTESIAN_POINT ( 'NONE',  ( -33.37998527947969052, -1.749200578933713279, 6.893343212288926658 ) ) ;
#17129=LINE ( 'NONE', #976, #57530 ) ;
#17131=CARTESIAN_POINT ( 'NONE',  ( 0.000000000000000000, 0.000000000000000000, 0.000000000000000000 ) ) ;
#17133=ORIENTED_EDGE ( 'NONE', *, *, #4240, .T. ) ;
#17135=LINE ( 'NONE', #1671, #17066 ) ;
#17143=ORIENTED_EDGE ( 'NONE', *, *, #49882, .F. ) ;
#17149=LINE ( 'NONE', #43191, #57535 ) ;
#17154=ORIENTED_EDGE ( 'NONE', *, *, #30555, .F. ) ;
#17155=EDGE_CURVE ( 'NONE', #16, #38237, #57955, .T. ) ;
#17158=VECTOR ( 'NONE', #66814, 1000.000000000000114 ) ;
#17170=VECTOR ( 'NONE', #5162, 1000.000000000000114 ) ;
#17176=AXIS2_PLACEMENT_3D ( 'NONE', #3994, #68363, #63773 ) ;
#17178=ORIENTED_EDGE ( 'NONE', *, *, #62319, .T. ) ;
#17179=DIRECTION ( 'NONE',  ( -0.5508969814521065267, 0.8345732537212999791, 0.000000000000000000 ) ) ;
#17181=ORIENTED_EDGE ( 'NONE', *, *, #57602, .F. ) ;
#17185=CARTESIAN_POINT ( 'NONE',  ( 45.74764628539832501, -59.37057832282265935, 41.38025477438755928 ) ) ;
#17187=VECTOR ( 'NONE', #52834, 1000.000000000000000 ) ;
#17191=CARTESIAN_POINT ( 'NONE',  ( -45.81425895439424778, 46.10914959592843587, 170.0000000000000000 ) ) ;
#17192=CARTESIAN_POINT ( 'NONE',  ( -34.79003307268509815, -38.19633032695429620, 26.66469066592268788 ) ) ;
#17203=ORIENTED_EDGE ( 'NONE', *, *, #18397, .T. ) ;
#17207=EDGE_LOOP ( 'NONE', ( #59578, #14563, #1327, #44123 ) ) ;
#17209=CARTESIAN_POINT ( 'NONE',  ( -60.57719029284778145, -27.78504199349144699, 34.48241795236666007 ) ) ;
#17216=EDGE_CURVE ( 'NONE', #1714, #1913, #28634, .T. ) ;
#17219=EDGE_CURVE ( 'NONE', #56212, #863, #39451, .T. ) ;
#17225=DIRECTION ( 'NONE',  ( -0.8584487936018727616, 0.5128992774058949156, 0.000000000000000000 ) ) ;
#17234=LINE ( 'NONE', #55221, #13986 ) ;
#17237=VERTEX_POINT ( 'NONE', #49718 ) ;
#17243=EDGE_CURVE ( 'NONE', #64171, #45918, #55001, .T. ) ;
#17245=DIRECTION ( 'NONE',  ( -0.000000000000000000, -0.000000000000000000, -1.000000000000000000 ) ) ;
#17251=CARTESIAN_POINT ( 'NONE',  ( -31.90315521289150524, 56.64813493366005304, 0.000000000000000000 ) ) ;
#17252=ORIENTED_EDGE ( 'NONE', *, *, #66000, .F. ) ;
#17254=DIRECTION ( 'NONE',  ( -0.000000000000000000, -0.000000000000000000, -1.000000000000000000 ) ) ;
#17261=FACE_OUTER_BOUND ( 'NONE', #21729, .T. ) ;
#17264=DIRECTION ( 'NONE',  ( 0.000000000000000000, 0.000000000000000000, 1.000000000000000000 ) ) ;
#17281=AXIS2_PLACEMENT_3D ( 'NONE', #24497, #8659, #51565 ) ;
#17286=EDGE_CURVE ( 'NONE', #863, #24361, #39197, .T. ) ;
#17287=AXIS2_PLACEMENT_3D ( 'NONE', #66229, #27870, #65879 ) ;
#17289=CARTESIAN_POINT ( 'NONE',  ( -10.50008294601455106, -40.38642021005834692, 13.79046340968178974 ) ) ;
#17294=CARTESIAN_POINT ( 'NONE',  ( -44.00727179482512241, -47.83680621839620528, 40.00000000000003553 ) ) ;
#17297=ORIENTED_EDGE ( 'NONE', *, *, #64380, .T. ) ;
#17303=FACE_OUTER_BOUND ( 'NONE', #65406, .T. ) ;
#17307=EDGE_CURVE ( 'NONE', #37904, #65910, #1547, .T. ) ;
#17322=CARTESIAN_POINT ( 'NONE',  ( -4.180838820195678096, -65.23214221112786504, 41.38025477438755928 ) ) ;
#17331=CONICAL_SURFACE ( 'NONE', #18456, 65.00000000000000000, 0.7853981633974497223 ) ;
#17335=CARTESIAN_POINT ( 'NONE',  ( -39.55079474733624068, -51.59997227571040668, 0.000000000000000000 ) ) ;
#17350=CARTESIAN_POINT ( 'NONE',  ( 26.98325885506551813, 31.83109204562614636, 13.79046340968179152 ) ) ;
#17354=LINE ( 'NONE', #38831, #27280 ) ;
#17360=B_SPLINE_CURVE_WITH_KNOTS ( 'NONE', 3,
 ( #1182, #12436, #49348, #17350, #13141, #17718 ),
 .UNSPECIFIED., .F., .F.,
 ( 4, 2, 4 ),
 ( 1.095770181108053550E-06, 0.03239442681617710207, 0.06478775786217309818 ),
 .UNSPECIFIED. ) ;
#17362=PLANE ( 'NONE',  #24832 ) ;
#17368=ORIENTED_EDGE ( 'NONE', *, *, #39723, .F. ) ;
#17369=VECTOR ( 'NONE', #43543, 999.9999999999998863 ) ;
#17373=ADVANCED_FACE ( 'NONE', ( #34266 ), #44459, .T. ) ;
#17376=DIRECTION ( 'NONE',  ( 0.9639628606958512425, 0.2660368455666826670, 0.000000000000000000 ) ) ;
#17388=CARTESIAN_POINT ( 'NONE',  ( -29.47687737404360675, -68.96458294135908318, 43.58025477438756212 ) ) ;
#17391=EDGE_CURVE ( 'NONE', #64034, #55870, #7538, .T. ) ;
#17399=ORIENTED_EDGE ( 'NONE', *, *, #56393, .F. ) ;
#17405=CARTESIAN_POINT ( 'NONE',  ( 0.000000000000000000, 0.000000000000000000, 0.000000000000000000 ) ) ;
#17407=CARTESIAN_POINT ( 'NONE',  ( -62.97854483871577713, 16.08424353203677271, 170.0000000000000000 ) ) ;
#17410=CARTESIAN_POINT ( 'NONE',  ( 36.85262215550067566, 53.56030941157737146, 170.0000000000000000 ) ) ;
#17411=DIRECTION ( 'NONE',  ( -1.000000000000000000, 0.000000000000000000, 2.312964634635743450E-16 ) ) ;
#17415=VECTOR ( 'NONE', #21481, 1000.000000000000000 ) ;
#17427=EDGE_CURVE ( 'NONE', #35065, #1572, #19818, .T. ) ;
#17429=FACE_OUTER_BOUND ( 'NONE', #4820, .T. ) ;
#17439=ORIENTED_EDGE ( 'NONE', *, *, #48024, .T. ) ;
#17440=ORIENTED_EDGE ( 'NONE', *, *, #38264, .F. ) ;
#17443=CARTESIAN_POINT ( 'NONE',  ( 55.14772863908673628, -34.40534879854659778, 170.0000000000000000 ) ) ;
#17446=PLANE ( 'NONE',  #53920 ) ;
#17459=CARTESIAN_POINT ( 'NONE',  ( 36.44731296966019585, -20.32014095137187581, 13.79046412351413586 ) ) ;
#17460=EDGE_CURVE ( 'NONE', #11439, #59098, #35652, .T. ) ;
#17461=FACE_OUTER_BOUND ( 'NONE', #21587, .T. ) ;
#17463=CARTESIAN_POINT ( 'NONE',  ( -41.31727360890798906, 62.59299402909750398, 0.000000000000000000 ) ) ;
#17465=VERTEX_POINT ( 'NONE', #24408 ) ;
#17469=DIRECTION ( 'NONE',  ( -0.8090169943749506709, 0.5877852522924686962, 0.000000000000000000 ) ) ;
#17483=VECTOR ( 'NONE', #17469, 1000.000000000000114 ) ;
#17485=AXIS2_PLACEMENT_3D ( 'NONE', #24691, #14475, #41550 ) ;
#17498=CARTESIAN_POINT ( 'NONE',  ( -8.663926357538780820, -23.45072237845004182, 0.000000000000000000 ) ) ;
#17499=ORIENTED_EDGE ( 'NONE', *, *, #48620, .F. ) ;
#17506=VERTEX_POINT ( 'NONE', #68011 ) ;
#17508=CYLINDRICAL_SURFACE ( 'NONE', #16083, 65.00000000000000000 ) ;
#17512=DIRECTION ( 'NONE',  ( 0.1342332658176522697, 0.9909497617679352555, 0.000000000000000000 ) ) ;
#17519=DIRECTION ( 'NONE',  ( 1.000000000000000000, 0.000000000000000000, 0.000000000000000000 ) ) ;
#17520=ORIENTED_EDGE ( 'NONE', *, *, #5526, .F. ) ;
#17523=VERTEX_POINT ( 'NONE', #68352 ) ;
#17526=VECTOR ( 'NONE', #20340, 1000.000000000000000 ) ;
#17528=DIRECTION ( 'NONE',  ( -0.1342332658176667304, 0.9909497617679331460, 0.000000000000000000 ) ) ;
#17529=CARTESIAN_POINT ( 'NONE',  ( -14.79841479960649053, 20.14961338137236524, 0.000000000000000000 ) ) ;
#17533=EDGE_CURVE ( 'NONE', #14951, #19095, #167, .T. ) ;
#17546=EDGE_CURVE ( 'NONE', #25148, #67708, #25754, .T. ) ;
#17549=CARTESIAN_POINT ( 'NONE',  ( -64.83840629396344468, -4.580509716060184644, 170.0000000000000000 ) ) ;
#17551=EDGE_CURVE ( 'NONE', #33479, #56882, #57423, .T. ) ;
#17553=CARTESIAN_POINT ( 'NONE',  ( 0.000000000000000000, 0.000000000000000000, 41.38025477438755928 ) ) ;
#17560=VERTEX_POINT ( 'NONE', #31740 ) ;
#17564=CARTESIAN_POINT ( 'NONE',  ( 0.000000000000000000, 0.000000000000000000, 170.0000000000000000 ) ) ;
#17565=EDGE_CURVE ( 'NONE', #43248, #67200, #20489, .T. ) ;
#17568=ORIENTED_EDGE ( 'NONE', *, *, #27312, .T. ) ;
#17571=EDGE_CURVE ( 'NONE', #41223, #53910, #22928, .T. ) ;
#17572=PLANE ( 'NONE',  #67174 ) ;
#17573=ORIENTED_EDGE ( 'NONE', *, *, #17607, .F. ) ;
#17587=VECTOR ( 'NONE', #2861, 1000.000000000000000 ) ;
#17592=ORIENTED_EDGE ( 'NONE', *, *, #2324, .T. ) ;
#17595=ORIENTED_EDGE ( 'NONE', *, *, #23035, .F. ) ;
#17598=CONICAL_SURFACE ( 'NONE', #21014, 65.00000000000000000, 0.7853981633974497223 ) ;
#17604=ORIENTED_EDGE ( 'NONE', *, *, #18567, .T. ) ;
#17605=PLANE ( 'NONE',  #55914 ) ;
#17607=EDGE_CURVE ( 'NONE', #34928, #25277, #34973, .T. ) ;
#17614=DIRECTION ( 'NONE',  ( -0.7530714660036196273, 0.6579387259397027066, 0.000000000000000000 ) ) ;
#17616=ORIENTED_EDGE ( 'NONE', *, *, #57350, .F. ) ;
#17618=DIRECTION ( 'NONE',  ( 0.9362348706397417564, -0.3513748240813305279, 0.000000000000000000 ) ) ;
#17630=EDGE_CURVE ( 'NONE', #20617, #14760, #51897, .T. ) ;
#17633=CONICAL_SURFACE ( 'NONE', #26609, 65.00000000000000000, 0.7853981633974497223 ) ;
#17641=FACE_OUTER_BOUND ( 'NONE', #12191, .T. ) ;
#17644=DIRECTION ( 'NONE',  ( 0.000000000000000000, -0.000000000000000000, -1.000000000000000000 ) ) ;
#17652=DIRECTION ( 'NONE',  ( -0.000000000000000000, -0.000000000000000000, -1.000000000000000000 ) ) ;
#17659=ADVANCED_FACE ( 'NONE', ( #57365 ), #26050, .T. ) ;
#17663=CARTESIAN_POINT ( 'NONE',  ( 63.74253542338308165, -39.54050679744447905, 43.58025477438756212 ) ) ;
#17670=CARTESIAN_POINT ( 'NONE',  ( 8.828807734114020533, 74.48902371486721563, 170.0000000000000000 ) ) ;
#17676=CIRCLE ( 'NONE', #49075, 65.00000000000000000 ) ;
#17677=ORIENTED_EDGE ( 'NONE', *, *, #54218, .T. ) ;
#17679=DIRECTION ( 'NONE',  ( -0.000000000000000000, -0.000000000000000000, -1.000000000000000000 ) ) ;
#17683=FACE_OUTER_BOUND ( 'NONE', #37687, .T. ) ;
#17696=PLANE ( 'NONE',  #64303 ) ;
#17698=VECTOR ( 'NONE', #27453, 1000.000000000000000 ) ;
#17700=AXIS2_PLACEMENT_3D ( 'NONE', #38029, #5659, #59473 ) ;
#17701=ADVANCED_FACE ( 'NONE', ( #63681 ), #5274, .T. ) ;
#17704=LINE ( 'NONE', #44780, #4884 ) ;
#17716=EDGE_CURVE ( 'NONE', #1146, #44628, #14458, .T. ) ;
#17718=CARTESIAN_POINT ( 'NONE',  ( 16.62148331457488837, 18.83783649008728744, 0.000000000000000000 ) ) ;
#17723=ORIENTED_EDGE ( 'NONE', *, *, #17216, .T. ) ;
#17726=EDGE_CURVE ( 'NONE', #36414, #4077, #60120, .T. ) ;
#17728=FACE_OUTER_BOUND ( 'NONE', #19222, .T. ) ;
#17730=FACE_OUTER_BOUND ( 'NONE', #10068, .T. ) ;
#17731=EDGE_CURVE ( 'NONE', #30832, #56795, #50739, .T. ) ;
#17733=LINE ( 'NONE', #59919, #23677 ) ;
#17738=VERTEX_POINT ( 'NONE', #41878 ) ;
#17758=ORIENTED_EDGE ( 'NONE', *, *, #13797, .T. ) ;
#17759=CARTESIAN_POINT ( 'NONE',  ( -56.44201257846587083, -32.26641783793643725, 43.58025477438756923 ) ) ;
#17764=ORIENTED_EDGE ( 'NONE', *, *, #28676, .T. ) ;
#17770=LINE ( 'NONE', #22342, #1576 ) ;
#17779=EDGE_CURVE ( 'NONE', #52894, #61203, #12292, .T. ) ;
#17783=ORIENTED_EDGE ( 'NONE', *, *, #50041, .T. ) ;
#17784=CIRCLE ( 'NONE', #9950, 65.36598343705435354 ) ;
#17785=CARTESIAN_POINT ( 'NONE',  ( 21.38432669263065833, -61.76910524360950916, 43.58025477438756212 ) ) ;
#17792=VERTEX_POINT ( 'NONE', #16166 ) ;
#17796=CARTESIAN_POINT ( 'NONE',  ( 26.12852347772543737, 70.00000000000000000, 129.5802547743875550 ) ) ;
#17801=LINE ( 'NONE', #7243, #14031 ) ;
#17805=ADVANCED_FACE ( 'NONE', ( #12291 ), #27063, .T. ) ;
#17817=DIRECTION ( 'NONE',  ( -0.000000000000000000, 0.000000000000000000, -1.000000000000000000 ) ) ;
#17820=DIRECTION ( 'NONE',  ( 1.000000000000000000, 0.000000000000000000, 0.000000000000000000 ) ) ;
#17824=CARTESIAN_POINT ( 'NONE',  ( -15.45727656667689409, 73.34020256436167529, 41.38025477438755928 ) ) ;
#17826=DIRECTION ( 'NONE',  ( 2.241020959626597081E-17, 2.489978219820159838E-16, 1.000000000000000000 ) ) ;
#17829=LINE ( 'NONE', #60729, #44345 ) ;
#17830=ORIENTED_EDGE ( 'NONE', *, *, #22083, .F. ) ;
#17831=CARTESIAN_POINT ( 'NONE',  ( 0.000000000000000000, 0.000000000000000000, 0.000000000000000000 ) ) ;
#17837=AXIS2_PLACEMENT_3D ( 'NONE', #23048, #1953, #38166 ) ;
#17840=DIRECTION ( 'NONE',  ( 0.000000000000000000, 0.000000000000000000, 1.000000000000000000 ) ) ;
#17845=CARTESIAN_POINT ( 'NONE',  ( -21.27554331372911989, -61.43430442924893953, 3.061616997868437868E-16 ) ) ;
#17855=DIRECTION ( 'NONE',  ( -4.974206872490789458E-18, 1.135330258912604340E-18, -1.000000000000000000 ) ) ;
#17859=DIRECTION ( 'NONE',  ( -0.000000000000000000, -0.000000000000000000, -1.000000000000000000 ) ) ;
#17869=EDGE_CURVE ( 'NONE', #52056, #41640, #43996, .T. ) ;
#17894=ORIENTED_EDGE ( 'NONE', *, *, #31767, .F. ) ;
#17907=DIRECTION ( 'NONE',  ( -1.000000000000000000, 0.000000000000000000, 0.000000000000000000 ) ) ;
#17914=PLANE ( 'NONE',  #53266 ) ;
#17921=ORIENTED_EDGE ( 'NONE', *, *, #26267, .T. ) ;
#17923=FACE_OUTER_BOUND ( 'NONE', #38591, .T. ) ;
#17935=EDGE_LOOP ( 'NONE', ( #14977, #42204, #58935, #65359 ) ) ;
#17938=FACE_OUTER_BOUND ( 'NONE', #8458, .T. ) ;
#17948=ORIENTED_EDGE ( 'NONE', *, *, #4289, .T. ) ;
#17950=CARTESIAN_POINT ( 'NONE',  ( 74.62299871641495486, 5.461138973199058277, 170.0000000000000000 ) ) ;
#17956=ADVANCED_FACE ( 'NONE', ( #25119 ), #45111, .T. ) ;
#17957=LINE ( 'NONE', #39066, #49661 ) ;
#17958=ORIENTED_EDGE ( 'NONE', *, *, #57887, .T. ) ;
#17971=AXIS2_PLACEMENT_3D ( 'NONE', #1360, #16491, #22815 ) ;
#17973=ADVANCED_FACE ( 'NONE', ( #11244, #705 ), #26746, .T. ) ;
#17975=CARTESIAN_POINT ( 'NONE',  ( -26.83517958587572494, -59.60356471962950309, 43.58025477438756212 ) ) ;
#17979=CARTESIAN_POINT ( 'NONE',  ( 41.72486082342750535, 50.31647622756258187, 41.38025477438755928 ) ) ;
#17982=DIRECTION ( 'NONE',  ( 0.1342332658176522420, 0.9909497617679351444, 0.000000000000000000 ) ) ;
#17990=CARTESIAN_POINT ( 'NONE',  ( -24.53636015449704644, -60.58612729876431047, 43.58025477438756212 ) ) ;
#17993=DIRECTION ( 'NONE',  ( 1.000000000000000000, 1.243449787580175325E-14, 0.000000000000000000 ) ) ;
#17997=ORIENTED_EDGE ( 'NONE', *, *, #11256, .T. ) ;
#18001=PLANE ( 'NONE',  #41285 ) ;
#18002=DIRECTION ( 'NONE',  ( 1.000000000000000000, 0.000000000000000000, 0.000000000000000000 ) ) ;
#18004=AXIS2_PLACEMENT_3D ( 'NONE', #38558, #60003, #11825 ) ;
#18005=CARTESIAN_POINT ( 'NONE',  ( 74.01791526339553684, 12.16185512414947034, 43.58025477438756212 ) ) ;
#18012=EDGE_CURVE ( 'NONE', #17792, #42599, #48442, .T. ) ;
#18014=EDGE_CURVE ( 'NONE', #5114, #308, #63096, .T. ) ;
#18016=CARTESIAN_POINT ( 'NONE',  ( -62.31345272479885011, -18.49415068377726712, 170.0000000000000000 ) ) ;
#18019=LINE ( 'NONE', #22593, #45555 ) ;
#18051=ORIENTED_EDGE ( 'NONE', *, *, #22900, .F. ) ;
#18054=EDGE_CURVE ( 'NONE', #11417, #1085, #10209, .T. ) ;
#18056=ORIENTED_EDGE ( 'NONE', *, *, #49135, .F. ) ;
#18059=CARTESIAN_POINT ( 'NONE',  ( -13.60872009721716935, -65.24114748995962998, 34.48241823981439325 ) ) ;
#18062=EDGE_CURVE ( 'NONE', #15601, #22641, #32373, .T. ) ;
#18070=PLANE ( 'NONE',  #65463 ) ;
#18076=VECTOR ( 'NONE', #20236, 1000.000000000000000 ) ;
#18101=ORIENTED_EDGE ( 'NONE', *, *, #64138, .T. ) ;
#18105=LINE ( 'NONE', #56424, #61526 ) ;
#18114=AXIS2_PLACEMENT_3D ( 'NONE', #47557, #30716, #69016 ) ;
#18115=ORIENTED_EDGE ( 'NONE', *, *, #9996, .F. ) ;
#18119=FACE_OUTER_BOUND ( 'NONE', #69094, .T. ) ;
#18125=VECTOR ( 'NONE', #926, 1000.000000000000000 ) ;
#18149=ORIENTED_EDGE ( 'NONE', *, *, #17551, .T. ) ;
#18151=AXIS2_PLACEMENT_3D ( 'NONE', #47319, #25553, #48006 ) ;
#18166=AXIS2_PLACEMENT_3D ( 'NONE', #37635, #4942, #59085 ) ;
#18169=DIRECTION ( 'NONE',  ( -0.8805955318567321166, -0.4738686624730094055, 0.000000000000000000 ) ) ;
#18182=ADVANCED_FACE ( 'NONE', ( #60135 ), #39732, .F. ) ;
#18185=EDGE_CURVE ( 'NONE', #19578, #55116, #61191, .T. ) ;
#18193=ORIENTED_EDGE ( 'NONE', *, *, #45326, .F. ) ;
#18207=ORIENTED_EDGE ( 'NONE', *, *, #41309, .F. ) ;
#18218=VERTEX_POINT ( 'NONE', #33423 ) ;
#18226=CARTESIAN_POINT ( 'NONE',  ( -24.53636015449705354, -60.58612729876431047, 41.38025477438755928 ) ) ;
#18239=VERTEX_POINT ( 'NONE', #28123 ) ;
#18241=CARTESIAN_POINT ( 'NONE',  ( 35.16506477614511539, 22.46626293537709529, 13.79046412351414475 ) ) ;
#18244=DIRECTION ( 'NONE',  ( -0.000000000000000000, -0.000000000000000000, -1.000000000000000000 ) ) ;
#18253=LINE ( 'NONE', #47302, #47562 ) ;
#18255=CARTESIAN_POINT ( 'NONE',  ( 51.85299110299440173, 39.21848821248450179, 0.000000000000000000 ) ) ;
#18258=ORIENTED_EDGE ( 'NONE', *, *, #30823, .T. ) ;
#18268=MANIFOLD_SOLID_BREP ( 'Cut-Extrude3', #12595 ) ;
#18272=ORIENTED_EDGE ( 'NONE', *, *, #35809, .F. ) ;
#18274=DIRECTION ( 'NONE',  ( -0.000000000000000000, -0.000000000000000000, -1.000000000000000000 ) ) ;
#18292=AXIS2_PLACEMENT_3D ( 'NONE', #48383, #16056, #220 ) ;
#18297=AXIS2_PLACEMENT_3D ( 'NONE', #41682, #35373, #19181 ) ;
#18302=LINE ( 'NONE', #61216, #7348 ) ;
#18310=DIRECTION ( 'NONE',  ( 1.000000000000000000, 0.000000000000000000, 0.000000000000000000 ) ) ;
#18311=VERTEX_POINT ( 'NONE', #3830 ) ;
#18319=DIRECTION ( 'NONE',  ( -0.000000000000000000, -0.000000000000000000, -1.000000000000000000 ) ) ;
#18324=CARTESIAN_POINT ( 'NONE',  ( -40.24154210098803475, 63.23235722614447951, 41.38025477438755928 ) ) ;
#18325=ORIENTED_EDGE ( 'NONE', *, *, #27485, .F. ) ;
#18328=CARTESIAN_POINT ( 'NONE',  ( -62.66631205405160188, -18.59153367093452047, 41.38025477438755928 ) ) ;
#18337=EDGE_CURVE ( 'NONE', #30965, #8346, #38434, .T. ) ;
#18338=CARTESIAN_POINT ( 'NONE',  ( 0.000000000000000000, 0.000000000000000000, 40.00000000000003553 ) ) ;
#18341=VECTOR ( 'NONE', #54932, 1000.000000000000000 ) ;
#18350=DIRECTION ( 'NONE',  ( -0.000000000000000000, -0.000000000000000000, -1.000000000000000000 ) ) ;
#18351=CARTESIAN_POINT ( 'NONE',  ( -59.09450113343241640, 27.07101652673493319, 40.00000000000003553 ) ) ;
#18353=VECTOR ( 'NONE', #2846, 1000.000000000000000 ) ;
#18358=FACE_OUTER_BOUND ( 'NONE', #34983, .T. ) ;
#18366=B_SPLINE_CURVE_WITH_KNOTS ( 'NONE', 3,
 ( #40486, #61934, #46107, #32014 ),
 .UNSPECIFIED., .F., .F.,
 ( 4, 4 ),
 ( 0.1259919275528360583, 0.1829744153748752433 ),
 .UNSPECIFIED. ) ;
#18370=ORIENTED_EDGE ( 'NONE', *, *, #42418, .T. ) ;
#18371=CARTESIAN_POINT ( 'NONE',  ( -72.57286576968809300, 18.73210786364346703, 41.38025477438755928 ) ) ;
#18397=EDGE_CURVE ( 'NONE', #67683, #36964, #11304, .T. ) ;
#18400=VECTOR ( 'NONE', #13322, 1000.000000000000000 ) ;
#18403=DIRECTION ( 'NONE',  ( -0.000000000000000000, -0.000000000000000000, -1.000000000000000000 ) ) ;
#18408=AXIS2_PLACEMENT_3D ( 'NONE', #30223, #51674, #18622 ) ;
#18410=ORIENTED_EDGE ( 'NONE', *, *, #29227, .F. ) ;
#18411=ORIENTED_EDGE ( 'NONE', *, *, #43333, .F. ) ;
#18418=DIRECTION ( 'NONE',  ( -0.000000000000000000, -0.000000000000000000, 1.000000000000000000 ) ) ;
#18420=ORIENTED_EDGE ( 'NONE', *, *, #56136, .F. ) ;
#18423=EDGE_CURVE ( 'NONE', #16594, #13447, #49507, .T. ) ;
#18433=EDGE_LOOP ( 'NONE', ( #64907, #54509, #37131, #39710 ) ) ;
#18443=LINE ( 'NONE', #17388, #27619 ) ;
#18455=EDGE_CURVE ( 'NONE', #38758, #12492, #17129, .T. ) ;
#18456=AXIS2_PLACEMENT_3D ( 'NONE', #57201, #57546, #9019 ) ;
#18458=VECTOR ( 'NONE', #51216, 1000.000000000000000 ) ;
#18461=PLANE ( 'NONE',  #20354 ) ;
#18463=VERTEX_POINT ( 'NONE', #39995 ) ;
#18474=ORIENTED_EDGE ( 'NONE', *, *, #13190, .T. ) ;
#18475=B_SPLINE_CURVE_WITH_KNOTS ( 'NONE', 3,
 ( #55619, #49635, #16933, #7087, #54913, #6737 ),
 .UNSPECIFIED., .F., .F.,
 ( 4, 2, 4 ),
 ( 0.03218932480516799310, 0.06469831007220608332, 0.09720729533924417354 ),
 .UNSPECIFIED. ) ;
#18481=ORIENTED_EDGE ( 'NONE', *, *, #9993, .F. ) ;
#18482=CARTESIAN_POINT ( 'NONE',  ( -20.06363827490053708, -32.66413954409357245, 13.32819299319723427 ) ) ;
#18489=DIRECTION ( 'NONE',  ( -1.282270072030875824E-16, -2.146158602472697874E-16, 1.000000000000000000 ) ) ;
#18497=CARTESIAN_POINT ( 'NONE',  ( 0.000000000000000000, 0.000000000000000000, 40.00000000000003553 ) ) ;
#18500=CARTESIAN_POINT ( 'NONE',  ( -42.36049017605873956, -61.90437280228297112, 170.0000000000000000 ) ) ;
#18501=DIRECTION ( 'NONE',  ( 0.5877852522924685852, 0.8090169943749507819, -0.000000000000000000 ) ) ;
#18509=AXIS2_PLACEMENT_3D ( 'NONE', #3757, #34743, #19584 ) ;
#18517=ADVANCED_FACE ( 'NONE', ( #14307 ), #68459, .T. ) ;
#18518=CARTESIAN_POINT ( 'NONE',  ( 57.84269266929310049, -33.10328523389011934, 34.48241823993598842 ) ) ;
#18524=CARTESIAN_POINT ( 'NONE',  ( 24.36509522349081536, -70.94296747916753532, 43.58025477438756923 ) ) ;
#18525=CARTESIAN_POINT ( 'NONE',  ( 0.000000000000000000, 0.000000000000000000, 73.58025477438756923 ) ) ;
#18528=FACE_OUTER_BOUND ( 'NONE', #8559, .T. ) ;
#18543=AXIS2_PLACEMENT_3D ( 'NONE', #38467, #5420, #43035 ) ;
#18544=CARTESIAN_POINT ( 'NONE',  ( 18.89356949897907967, -62.19351277735683681, 40.00000000000003553 ) ) ;
#18553=CARTESIAN_POINT ( 'NONE',  ( -26.69131247781301752, 59.26697088776972322, 170.0000000000000000 ) ) ;
#18554=VECTOR ( 'NONE', #50047, 1000.000000000000000 ) ;
#18567=EDGE_CURVE ( 'NONE', #34081, #41081, #46649, .T. ) ;
#18573=ORIENTED_EDGE ( 'NONE', *, *, #11327, .F. ) ;
#18576=DIRECTION ( 'NONE',  ( -1.000000000000000000, 0.000000000000000000, 0.000000000000000000 ) ) ;
#18586=ORIENTED_EDGE ( 'NONE', *, *, #54298, .T. ) ;
#18599=CARTESIAN_POINT ( 'NONE',  ( 60.82895951008336510, 30.68107831874607072, 41.38025477438755928 ) ) ;
#18602=ORIENTED_EDGE ( 'NONE', *, *, #12454, .T. ) ;
#18622=DIRECTION ( 'NONE',  ( -1.000000000000000000, 0.000000000000000000, 0.000000000000000000 ) ) ;
#18628=DIRECTION ( 'NONE',  ( 0.000000000000000000, 0.000000000000000000, 1.000000000000000000 ) ) ;
#18629=DIRECTION ( 'NONE',  ( 1.000000000000000000, 0.000000000000000000, 0.000000000000000000 ) ) ;
#18632=CARTESIAN_POINT ( 'NONE',  ( 1.667562369267757916, -64.99262834925670518, 41.38025477438755928 ) ) ;
#18644=CARTESIAN_POINT ( 'NONE',  ( -26.83517958587572494, -59.60356471962950309, 6.377659838150123602E-18 ) ) ;
#18645=CARTESIAN_POINT ( 'NONE',  ( 51.85299110299440173, 39.21848821248450179, 43.58025477438756923 ) ) ;
#18648=AXIS2_PLACEMENT_3D ( 'NONE', #23723, #11763, #22323 ) ;
#18650=EDGE_CURVE ( 'NONE', #2615, #17123, #40022, .T. ) ;
#18660=EDGE_CURVE ( 'NONE', #54950, #43717, #31605, .T. ) ;
#18682=EDGE_CURVE ( 'NONE', #65787, #9934, #55142, .T. ) ;
#18684=ADVANCED_FACE ( 'NONE', ( #43777 ), #17043, .T. ) ;
#18691=ORIENTED_EDGE ( 'NONE', *, *, #64559, .F. ) ;
#18694=CARTESIAN_POINT ( 'NONE',  ( -45.81425895439424067, 46.10914959592843587, 40.00000000000003553 ) ) ;
#18698=CARTESIAN_POINT ( 'NONE',  ( -28.32746765835526048, 69.45586423092609607, 170.0000000000000000 ) ) ;
#18701=VERTEX_POINT ( 'NONE', #6512 ) ;
#18702=LINE ( 'NONE', #30298, #63729 ) ;
#18726=ORIENTED_EDGE ( 'NONE', *, *, #26052, .F. ) ;
#18731=ORIENTED_EDGE ( 'NONE', *, *, #33758, .T. ) ;
#18733=ADVANCED_FACE ( 'NONE', ( #27959 ), #18461, .T. ) ;
#18742=ORIENTED_EDGE ( 'NONE', *, *, #26426, .F. ) ;
#18743=EDGE_CURVE ( 'NONE', #33925, #28657, #24836, .T. ) ;
#18744=VECTOR ( 'NONE', #1240, 1000.000000000000114 ) ;
#18745=ORIENTED_EDGE ( 'NONE', *, *, #67407, .T. ) ;
#18755=CARTESIAN_POINT ( 'NONE',  ( -47.92160691800343386, 33.27200046441025449, 27.58472369410210945 ) ) ;
#18757=DIRECTION ( 'NONE',  ( 1.000000000000000000, 0.000000000000000000, 0.000000000000000000 ) ) ;
#18768=FACE_OUTER_BOUND ( 'NONE', #63805, .T. ) ;
#18779=EDGE_LOOP ( 'NONE', ( #4748, #51066, #19117, #26551 ) ) ;
#18784=LINE ( 'NONE', #67674, #7049 ) ;
#18790=ORIENTED_EDGE ( 'NONE', *, *, #10456, .T. ) ;
#18806=ORIENTED_EDGE ( 'NONE', *, *, #53038, .T. ) ;
#18807=CARTESIAN_POINT ( 'NONE',  ( 0.000000000000000000, 0.000000000000000000, 0.000000000000000000 ) ) ;
#18827=FACE_OUTER_BOUND ( 'NONE', #41459, .T. ) ;
#18832=LINE ( 'NONE', #40289, #26636 ) ;
#18833=DIRECTION ( 'NONE',  ( 0.3090169943749446757, 0.9510565162951544194, 0.000000000000000000 ) ) ;
#18843=ORIENTED_EDGE ( 'NONE', *, *, #60485, .T. ) ;
#18849=ADVANCED_FACE ( 'NONE', ( #34654 ), #56090, .T. ) ;
#18859=CARTESIAN_POINT ( 'NONE',  ( 21.27121078971612889, 61.42097029141972087, 170.0000000000000000 ) ) ;
#18864=CARTESIAN_POINT ( 'NONE',  ( -64.61430802170492882, 7.070445451047392638, 40.00000000000003553 ) ) ;
#18872=CARTESIAN_POINT ( 'NONE',  ( -68.11501976657856972, 31.41506934893843805, 170.0000000000000000 ) ) ;
#18880=FACE_OUTER_BOUND ( 'NONE', #40775, .T. ) ;
#18885=CARTESIAN_POINT ( 'NONE',  ( -15.67984581960975632, -63.08044415722883969, 40.00000000000003553 ) ) ;
#18886=EDGE_CURVE ( 'NONE', #9754, #18311, #48387, .T. ) ;
#18893=EDGE_LOOP ( 'NONE', ( #63149, #58895, #41301, #56367 ) ) ;
#18899=VECTOR ( 'NONE', #32739, 1000.000000000000114 ) ;
#18900=DIRECTION ( 'NONE',  ( 0.3090169943749446757, 0.9510565162951544194, 0.000000000000000000 ) ) ;
#18901=CARTESIAN_POINT ( 'NONE',  ( 8.942470798084043437, 23.47701018505912174, 0.000000000000000000 ) ) ;
#18913=EDGE_LOOP ( 'NONE', ( #22387, #10672, #6363, #25179 ) ) ;
#18917=ORIENTED_EDGE ( 'NONE', *, *, #23269, .F. ) ;
#18922=DIRECTION ( 'NONE',  ( 0.9749279121818226201, 0.2225209339563184452, -2.254973782195817056E-16 ) ) ;
#18924=ORIENTED_EDGE ( 'NONE', *, *, #32183, .F. ) ;
#18930=CARTESIAN_POINT ( 'NONE',  ( -7.486743542470046364, 64.58150799671128084, 41.38025477438755928 ) ) ;
#18935=EDGE_LOOP ( 'NONE', ( #24739, #32010, #62953, #47248 ) ) ;
#18945=LINE ( 'NONE', #34448, #61783 ) ;
#18948=LINE ( 'NONE', #67487, #44976 ) ;
#18953=CARTESIAN_POINT ( 'NONE',  ( -65.36598343705435354, 0.000000000000000000, 41.38025477438755928 ) ) ;
#18956=ORIENTED_EDGE ( 'NONE', *, *, #59924, .F. ) ;
#18957=CARTESIAN_POINT ( 'NONE',  ( 32.64241790427570322, -7.194141594814827734, 6.893343212288940869 ) ) ;
#18977=DIRECTION ( 'NONE',  ( -0.000000000000000000, -0.000000000000000000, -1.000000000000000000 ) ) ;
#18981=EDGE_CURVE ( 'NONE', #61455, #7485, #69402, .T. ) ;
#18983=VERTEX_POINT ( 'NONE', #32120 ) ;
#18987=CIRCLE ( 'NONE', #15618, 65.36598343705435354 ) ;
#18992=CARTESIAN_POINT ( 'NONE',  ( -40.27405704175546930, -63.28161525591320924, 170.0000000000000000 ) ) ;
#18998=DIRECTION ( 'NONE',  ( -1.000000000000000000, 0.000000000000000000, 0.000000000000000000 ) ) ;
#19006=VERTEX_POINT ( 'NONE', #1148 ) ;
#19012=DIRECTION ( 'NONE',  ( -0.9959742939952397345, 0.08963930890342654279, 0.000000000000000000 ) ) ;
#19014=CARTESIAN_POINT ( 'NONE',  ( -26.69131247781221106, -59.26697088777007849, 170.0000000000000000 ) ) ;
#19029=ORIENTED_EDGE ( 'NONE', *, *, #31987, .F. ) ;
#19030=ORIENTED_EDGE ( 'NONE', *, *, #58743, .T. ) ;
#19032=DIRECTION ( 'NONE',  ( -0.000000000000000000, -0.000000000000000000, -1.000000000000000000 ) ) ;
#19036=AXIS2_PLACEMENT_3D ( 'NONE', #905, #43793, #17059 ) ;
#19039=CIRCLE ( 'NONE', #44900, 65.00000000000000000 ) ;
#19040=DIRECTION ( 'NONE',  ( -1.000000000000000000, 0.000000000000000000, 0.000000000000000000 ) ) ;
#19047=EDGE_CURVE ( 'NONE', #47961, #58719, #7120, .T. ) ;
#19051=DIRECTION ( 'NONE',  ( 0.8584487936018655452, 0.5128992774059070170, 0.000000000000000000 ) ) ;
#19053=LINE ( 'NONE', #13437, #1527 ) ;
#19056=VECTOR ( 'NONE', #10421, 1000.000000000000000 ) ;
#19062=CARTESIAN_POINT ( 'NONE',  ( 0.000000000000000000, 0.000000000000000000, 40.82842712474622004 ) ) ;
#19078=CARTESIAN_POINT ( 'NONE',  ( 0.000000000000000000, 0.000000000000000000, 41.38025477438755928 ) ) ;
#19085=CARTESIAN_POINT ( 'NONE',  ( -16.04603987767271533, 64.68484515506864341, 34.48241823981440746 ) ) ;
#19088=FACE_OUTER_BOUND ( 'NONE', #38833, .T. ) ;
#19090=DIRECTION ( 'NONE',  ( 0.1342332658176522420, 0.9909497617679352555, -0.000000000000000000 ) ) ;
#19095=VERTEX_POINT ( 'NONE', #60583 ) ;
#19114=CARTESIAN_POINT ( 'NONE',  ( 51.85299110299497016, -39.21848821248376993, 3.061616997868437868E-16 ) ) ;
#19117=ORIENTED_EDGE ( 'NONE', *, *, #68368, .T. ) ;
#19128=EDGE_CURVE ( 'NONE', #28008, #45254, #8009, .T. ) ;
#19129=EDGE_CURVE ( 'NONE', #24552, #1734, #56311, .T. ) ;
#19131=ORIENTED_EDGE ( 'NONE', *, *, #57502, .F. ) ;
#19140=ORIENTED_EDGE ( 'NONE', *, *, #25181, .T. ) ;
#19141=DIRECTION ( 'NONE',  ( 1.000000000000000000, 0.000000000000000000, 0.000000000000000000 ) ) ;
#19142=CARTESIAN_POINT ( 'NONE',  ( -16.68907004672281502, -73.11959341363693454, 0.000000000000000000 ) ) ;
#19153=VECTOR ( 'NONE', #18501, 1000.000000000000000 ) ;
#19163=DIRECTION ( 'NONE',  ( 0.000000000000000000, -1.000000000000000000, 0.000000000000000000 ) ) ;
#19175=DIRECTION ( 'NONE',  ( 0.4738686624729966379, 0.8805955318567391110, 0.000000000000000000 ) ) ;
#19178=LINE ( 'NONE', #23165, #15176 ) ;
#19180=DIRECTION ( 'NONE',  ( -0.000000000000000000, -0.000000000000000000, 1.000000000000000000 ) ) ;
#19181=DIRECTION ( 'NONE',  ( 0.000000000000000000, 0.000000000000000000, -1.000000000000000000 ) ) ;
#19188=ORIENTED_EDGE ( 'NONE', *, *, #11204, .T. ) ;
#19192=CARTESIAN_POINT ( 'NONE',  ( 23.93060502292675196, 7.646171227524815706, 0.000000000000000000 ) ) ;
#19198=AXIS2_PLACEMENT_3D ( 'NONE', #15763, #11167, #16456 ) ;
#19206=DIRECTION ( 'NONE',  ( 0.000000000000000000, 0.000000000000000000, 1.000000000000000000 ) ) ;
#19210=ORIENTED_EDGE ( 'NONE', *, *, #1044, .F. ) ;
#19213=VECTOR ( 'NONE', #8888, 1000.000000000000000 ) ;
#19216=LINE ( 'NONE', #62127, #49140 ) ;
#19222=EDGE_LOOP ( 'NONE', ( #48524, #50912, #18790, #60327 ) ) ;
#19231=DIRECTION ( 'NONE',  ( -1.000000000000000000, 0.000000000000000000, 0.000000000000000000 ) ) ;
#19243=ORIENTED_EDGE ( 'NONE', *, *, #44037, .F. ) ;
#19245=CIRCLE ( 'NONE', #14732, 65.36598343705435354 ) ;
#19251=VECTOR ( 'NONE', #14010, 999.9999999999998863 ) ;
#19255=CARTESIAN_POINT ( 'NONE',  ( -29.70166638324878150, -57.83280658984300970, 170.0000000000000000 ) ) ;
#19260=CARTESIAN_POINT ( 'NONE',  ( -48.12872802574198516, -43.70867239603780519, 170.0000000000000000 ) ) ;
#19265=CARTESIAN_POINT ( 'NONE',  ( -59.49248094505429663, 30.03746416324668900, 34.48241795236666718 ) ) ;
#19277=CARTESIAN_POINT ( 'NONE',  ( 64.38365952013991489, 38.46744580544303460, 0.000000000000000000 ) ) ;
#19285=ORIENTED_EDGE ( 'NONE', *, *, #25760, .T. ) ;
#19289=ORIENTED_EDGE ( 'NONE', *, *, #43529, .F. ) ;
#19291=DIRECTION ( 'NONE',  ( -0.9362348706397369824, -0.3513748240813435175, 0.000000000000000000 ) ) ;
#19302=VERTEX_POINT ( 'NONE', #29800 ) ;
#19308=VECTOR ( 'NONE', #58439, 1000.000000000000000 ) ;
#19312=EDGE_CURVE ( 'NONE', #25377, #69123, #61798, .T. ) ;
#19314=EDGE_LOOP ( 'NONE', ( #37356, #35762, #36812, #9506 ) ) ;
#19317=CARTESIAN_POINT ( 'NONE',  ( 0.000000000000000000, 0.000000000000000000, 41.38025477438755928 ) ) ;
#19321=EDGE_CURVE ( 'NONE', #36739, #65910, #39495, .T. ) ;
#19326=ORIENTED_EDGE ( 'NONE', *, *, #26758, .F. ) ;
#19334=ORIENTED_EDGE ( 'NONE', *, *, #53426, .T. ) ;
#19335=CARTESIAN_POINT ( 'NONE',  ( -72.57286576968809300, 18.73210786364346703, 41.38025477438755928 ) ) ;
#19340=FACE_OUTER_BOUND ( 'NONE', #51925, .T. ) ;
#19355=LINE ( 'NONE', #19014, #53835 ) ;
#19359=ORIENTED_EDGE ( 'NONE', *, *, #33892, .T. ) ;
#19361=CARTESIAN_POINT ( 'NONE',  ( 1.667562369266825550, 64.99262834925669097, 0.000000000000000000 ) ) ;
#19363=DIRECTION ( 'NONE',  ( -1.000000000000000000, 0.000000000000000000, 0.000000000000000000 ) ) ;
#19372=ORIENTED_EDGE ( 'NONE', *, *, #17571, .F. ) ;
#19373=ORIENTED_EDGE ( 'NONE', *, *, #24972, .T. ) ;
#19381=EDGE_CURVE ( 'NONE', #4738, #7351, #23780, .T. ) ;
#19391=VERTEX_POINT ( 'NONE', #13962 ) ;
#19393=LINE ( 'NONE', #46822, #31648 ) ;
#19395=DIRECTION ( 'NONE',  ( 0.000000000000000000, 0.000000000000000000, 1.000000000000000000 ) ) ;
#19402=CARTESIAN_POINT ( 'NONE',  ( 34.41143668122415988, 66.58502636910522199, 41.38025477438755928 ) ) ;
#19407=EDGE_LOOP ( 'NONE', ( #26407, #55770, #17783, #43299 ) ) ;
#19411=ORIENTED_EDGE ( 'NONE', *, *, #33057, .T. ) ;
#19412=VECTOR ( 'NONE', #31215, 1000.000000000000000 ) ;
#19414=LINE ( 'NONE', #66937, #65596 ) ;
#19415=DIRECTION ( 'NONE',  ( -0.000000000000000000, -0.000000000000000000, -1.000000000000000000 ) ) ;
#19441=EDGE_LOOP ( 'NONE', ( #64915, #32629, #11645, #58789 ) ) ;
#19445=AXIS2_PLACEMENT_3D ( 'NONE', #40135, #51725, #19363 ) ;
#19454=EDGE_LOOP ( 'NONE', ( #17019, #23571, #10383, #17440 ) ) ;
#19460=CARTESIAN_POINT ( 'NONE',  ( -35.06172898939804838, 15.49744344258353479, 13.32819299319722539 ) ) ;
#19462=EDGE_CURVE ( 'NONE', #5114, #17560, #35665, .T. ) ;
#19490=LINE ( 'NONE', #14225, #2938 ) ;
#19503=ORIENTED_EDGE ( 'NONE', *, *, #41443, .F. ) ;
#19506=CIRCLE ( 'NONE', #61093, 65.00000000000000000 ) ;
#19520=DIRECTION ( 'NONE',  ( -0.000000000000000000, -0.000000000000000000, -1.000000000000000000 ) ) ;
#19521=DIRECTION ( 'NONE',  ( -0.000000000000000000, -0.000000000000000000, -1.000000000000000000 ) ) ;
#19522=EDGE_CURVE ( 'NONE', #25277, #242, #547, .T. ) ;
#19539=ORIENTED_EDGE ( 'NONE', *, *, #61323, .F. ) ;
#19542=AXIS2_PLACEMENT_3D ( 'NONE', #24340, #66223, #67258 ) ;
#19546=CARTESIAN_POINT ( 'NONE',  ( 51.65020416916155455, -1.250000000000021760, 26.66469104408689006 ) ) ;
#19547=DIRECTION ( 'NONE',  ( 0.9959742939952397345, -0.08963930890342655666, 0.000000000000000000 ) ) ;
#19559=AXIS2_PLACEMENT_3D ( 'NONE', #11833, #34357, #60013 ) ;
#19576=EDGE_LOOP ( 'NONE', ( #52961, #51215, #7528, #12119, #40259, #37087, #26916, #15681, #20765 ) ) ;
#19578=VERTEX_POINT ( 'NONE', #47337 ) ;
#19580=DIRECTION ( 'NONE',  ( 0.000000000000000000, 0.000000000000000000, 1.000000000000000000 ) ) ;
#19584=DIRECTION ( 'NONE',  ( 1.000000000000000000, 0.000000000000000000, 0.000000000000000000 ) ) ;
#19599=EDGE_LOOP ( 'NONE', ( #59973, #54842, #54178, #10059 ) ) ;
#19602=VECTOR ( 'NONE', #61461, 1000.000000000000000 ) ;
#19619=DIRECTION ( 'NONE',  ( -1.000000000000000000, 0.000000000000000000, 0.000000000000000000 ) ) ;
#19625=CARTESIAN_POINT ( 'NONE',  ( 22.18075376363927020, -11.79626863379931656, 3.061616997868437868E-16 ) ) ;
#19629=LINE ( 'NONE', #47050, #55807 ) ;
#19631=CARTESIAN_POINT ( 'NONE',  ( -15.47041015649658391, 73.39774458108210808, 170.0000000000000000 ) ) ;
#19633=CARTESIAN_POINT ( 'NONE',  ( -51.55432439150845170, 3.384920705045805001, 26.66469066592269144 ) ) ;
#19635=ORIENTED_EDGE ( 'NONE', *, *, #61493, .F. ) ;
#19638=CARTESIAN_POINT ( 'NONE',  ( -31.73109799811232890, -21.50890718406003188, 13.32819397642332326 ) ) ;
#19641=ORIENTED_EDGE ( 'NONE', *, *, #23180, .T. ) ;
#19651=DIRECTION ( 'NONE',  ( -1.000000000000000000, 0.000000000000000000, 0.000000000000000000 ) ) ;
#19661=CARTESIAN_POINT ( 'NONE',  ( 0.000000000000000000, 0.000000000000000000, 2.000000000000001776 ) ) ;
#19662=ORIENTED_EDGE ( 'NONE', *, *, #17869, .F. ) ;
#19669=EDGE_CURVE ( 'NONE', #50834, #28566, #8761, .T. ) ;
#19676=ORIENTED_EDGE ( 'NONE', *, *, #53199, .F. ) ;
#19683=ADVANCED_FACE ( 'NONE', ( #39580 ), #44851, .T. ) ;
#19685=FACE_OUTER_BOUND ( 'NONE', #28952, .T. ) ;
#19716=DIRECTION ( 'NONE',  ( -0.000000000000000000, -0.000000000000000000, 1.000000000000000000 ) ) ;
#19722=EDGE_LOOP ( 'NONE', ( #51427, #5587, #31709, #28222 ) ) ;
#19725=EDGE_LOOP ( 'NONE', ( #15694, #62988, #52, #41722 ) ) ;
#19728=CARTESIAN_POINT ( 'NONE',  ( 16.54503815046451010, -18.74197728628616844, 0.000000000000000000 ) ) ;
#19731=ORIENTED_EDGE ( 'NONE', *, *, #3187, .F. ) ;
#19739=CIRCLE ( 'NONE', #2873, 74.95140232871122521 ) ;
#19749=CIRCLE ( 'NONE', #18648, 65.00000000000000000 ) ;
#19753=CYLINDRICAL_SURFACE ( 'NONE', #7848, 65.36598343705435354 ) ;
#19760=VECTOR ( 'NONE', #11912, 999.9999999999998863 ) ;
#19763=VERTEX_POINT ( 'NONE', #53908 ) ;
#19777=ADVANCED_FACE ( 'NONE', ( #64134 ), #45107, .T. ) ;
#19779=CARTESIAN_POINT ( 'NONE',  ( 45.82394788922869822, -46.11928342727429708, 0.000000000000000000 ) ) ;
#19793=VECTOR ( 'NONE', #14164, 1000.000000000000227 ) ;
#19802=DIRECTION ( 'NONE',  ( 0.000000000000000000, 1.000000000000000000, 0.000000000000000000 ) ) ;
#19810=CARTESIAN_POINT ( 'NONE',  ( 63.74253542338254164, 39.54050679744534591, 170.0000000000000000 ) ) ;
#19816=ORIENTED_EDGE ( 'NONE', *, *, #43225, .F. ) ;
#19818=LINE ( 'NONE', #40919, #64191 ) ;
#19819=LINE ( 'NONE', #14195, #62223 ) ;
#19828=CARTESIAN_POINT ( 'NONE',  ( 65.35403040894466642, -1.250000000000021982, 43.58025477438756212 ) ) ;
#19831=CARTESIAN_POINT ( 'NONE',  ( 65.02478361689730946, 37.39438481344068776, 170.0000000000000000 ) ) ;
#19835=CARTESIAN_POINT ( 'NONE',  ( -0.2498518584877217619, -33.42485110444322771, 6.893342931471429402 ) ) ;
#19844=VERTEX_POINT ( 'NONE', #38089 ) ;
#19851=CONICAL_SURFACE ( 'NONE', #20944, 65.00000000000000000, 0.7853981633974497223 ) ;
#19855=CARTESIAN_POINT ( 'NONE',  ( 50.03867889673311709, 42.05760816978183669, 43.58025477438756212 ) ) ;
#19858=CARTESIAN_POINT ( 'NONE',  ( -30.62628708973294422, -68.47330165179167238, 170.0000000000000000 ) ) ;
#19866=ADVANCED_FACE ( 'NONE', ( #51092 ), #50787, .T. ) ;
#19896=ORIENTED_EDGE ( 'NONE', *, *, #20532, .T. ) ;
#19905=DIRECTION ( 'NONE',  ( 0.9009688679024155933, 0.4338837391175656699, -0.000000000000000000 ) ) ;
#19910=VECTOR ( 'NONE', #44818, 1000.000000000000114 ) ;
#19918=VECTOR ( 'NONE', #38108, 1000.000000000000114 ) ;
#19936=ORIENTED_EDGE ( 'NONE', *, *, #9610, .F. ) ;
#19938=DIRECTION ( 'NONE',  ( -0.000000000000000000, -0.000000000000000000, -1.000000000000000000 ) ) ;
#19943=ORIENTED_EDGE ( 'NONE', *, *, #63021, .T. ) ;
#19947=EDGE_LOOP ( 'NONE', ( #47444, #64728, #55279, #37389 ) ) ;
#19949=AXIS2_PLACEMENT_3D ( 'NONE', #38572, #61077, #11839 ) ;
#19951=EDGE_CURVE ( 'NONE', #39418, #33970, #22880, .T. ) ;
#19953=AXIS2_PLACEMENT_3D ( 'NONE', #54843, #54134, #28829 ) ;
#19954=EDGE_CURVE ( 'NONE', #14760, #48854, #17957, .T. ) ;
#19966=CARTESIAN_POINT ( 'NONE',  ( -31.86613124579579903, 10.09122387767404838, 6.893343212288924882 ) ) ;
#19993=PLANE ( 'NONE',  #10649 ) ;
#20016=CIRCLE ( 'NONE', #68314, 65.36598343705435354 ) ;
#20017=ADVANCED_FACE ( 'NONE', ( #369 ), #5987, .T. ) ;
#20026=DIRECTION ( 'NONE',  ( 1.000000000000000000, 0.000000000000000000, -0.000000000000000000 ) ) ;
#20027=VERTEX_POINT ( 'NONE', #33786 ) ;
#20029=ORIENTED_EDGE ( 'NONE', *, *, #50041, .F. ) ;
#20042=ORIENTED_EDGE ( 'NONE', *, *, #11660, .T. ) ;
#20046=CARTESIAN_POINT ( 'NONE',  ( 0.000000000000000000, 0.000000000000000000, 40.00000000000003553 ) ) ;
#20047=ORIENTED_EDGE ( 'NONE', *, *, #8483, .T. ) ;
#20054=CARTESIAN_POINT ( 'NONE',  ( 30.12852347772543737, 100.0000000000000000, 133.5802547743875550 ) ) ;
#20061=DIRECTION ( 'NONE',  ( -0.000000000000000000, -0.000000000000000000, -1.000000000000000000 ) ) ;
#20070=ORIENTED_EDGE ( 'NONE', *, *, #62583, .F. ) ;
#20074=ORIENTED_EDGE ( 'NONE', *, *, #41613, .F. ) ;
#20078=CARTESIAN_POINT ( 'NONE',  ( 48.11816970607238630, 43.69944786994017960, 170.0000000000000000 ) ) ;
#20079=DIRECTION ( 'NONE',  ( 0.7818314824680221431, 0.6234898018587432533, 2.500042656554810340E-16 ) ) ;
#20082=CARTESIAN_POINT ( 'NONE',  ( -38.04732747637867618, 4.679373924310576527, 13.32819397642332326 ) ) ;
#20083=ORIENTED_EDGE ( 'NONE', *, *, #39070, .T. ) ;
#20091=CIRCLE ( 'NONE', #32441, 25.12245591505646303 ) ;
#20092=ORIENTED_EDGE ( 'NONE', *, *, #43084, .F. ) ;
#20111=CARTESIAN_POINT ( 'NONE',  ( 69.68177367721139603, 20.52767805628179332, 170.0000000000000000 ) ) ;
#20119=DIRECTION ( 'NONE',  ( -1.000000000000000000, 0.000000000000000000, 0.000000000000000000 ) ) ;
#20123=EDGE_LOOP ( 'NONE', ( #60111, #9552, #12672, #68997, #58996, #47267, #65608, #9635, #8455 ) ) ;
#20138=DIRECTION ( 'NONE',  ( 1.000000000000000000, 0.000000000000000000, 0.000000000000000000 ) ) ;
#20140=CIRCLE ( 'NONE', #36963, 65.36598343705435354 ) ;
#20144=CARTESIAN_POINT ( 'NONE',  ( 21.77974805481932918, -62.98608706026495696, 34.48241823983692456 ) ) ;
#20149=EDGE_CURVE ( 'NONE', #51034, #10115, #23835, .T. ) ;
#20151=DIRECTION ( 'NONE',  ( 0.000000000000000000, 0.000000000000000000, 1.000000000000000000 ) ) ;
#20156=CARTESIAN_POINT ( 'NONE',  ( 70.65683382808231272, -25.18281821780013274, 170.0000000000000000 ) ) ;
#20157=DIRECTION ( 'NONE',  ( -1.000000000000000000, 0.000000000000000000, 0.000000000000000000 ) ) ;
#20162=CARTESIAN_POINT ( 'NONE',  ( 33.08881014127219089, 4.734317623318680113, 6.893343212288931099 ) ) ;
#20165=CARTESIAN_POINT ( 'NONE',  ( -40.27405704175544088, -63.28161525591325187, 43.58025477438756923 ) ) ;
#20167=DIRECTION ( 'NONE',  ( 0.000000000000000000, 0.000000000000000000, 1.000000000000000000 ) ) ;
#20173=CARTESIAN_POINT ( 'NONE',  ( -9.744241498306646321, -37.07486245478190057, 13.32819397642333392 ) ) ;
#20174=CARTESIAN_POINT ( 'NONE',  ( 0.000000000000000000, 0.000000000000000000, 0.000000000000000000 ) ) ;
#20177=CARTESIAN_POINT ( 'NONE',  ( 0.000000000000000000, 0.000000000000000000, 41.38025477438755928 ) ) ;
#20180=ORIENTED_EDGE ( 'NONE', *, *, #38441, .T. ) ;
#20187=ORIENTED_EDGE ( 'NONE', *, *, #2155, .F. ) ;
#20190=CARTESIAN_POINT ( 'NONE',  ( -52.73319225379862019, -53.34578647582125654, 43.58025477438756212 ) ) ;
#20192=EDGE_CURVE ( 'NONE', #27636, #52661, #61560, .T. ) ;
#20194=ADVANCED_FACE ( 'NONE', ( #50650 ), #53031, .T. ) ;
#20206=VERTEX_POINT ( 'NONE', #63971 ) ;
#20209=AXIS2_PLACEMENT_3D ( 'NONE', #10947, #55246, #1097 ) ;
#20212=CARTESIAN_POINT ( 'NONE',  ( 2.129405171194437063, -25.03204795498853841, 0.000000000000000000 ) ) ;
#20215=DIRECTION ( 'NONE',  ( 0.000000000000000000, 0.000000000000000000, 1.000000000000000000 ) ) ;
#20224=CONICAL_SURFACE ( 'NONE', #32571, 65.00000000000000000, 0.7853981633974497223 ) ;
#20226=CARTESIAN_POINT ( 'NONE',  ( -19.46539569203835640, 15.68752276659279943, 0.000000000000000000 ) ) ;
#20229=ORIENTED_EDGE ( 'NONE', *, *, #59719, .T. ) ;
#20231=VERTEX_POINT ( 'NONE', #42174 ) ;
#20236=DIRECTION ( 'NONE',  ( 0.000000000000000000, 0.000000000000000000, 1.000000000000000000 ) ) ;
#20238=CIRCLE ( 'NONE', #15770, 25.12245591505646303 ) ;
#20244=CARTESIAN_POINT ( 'NONE',  ( 20.86596583059835552, 36.13760021380633702, 13.79046340968177908 ) ) ;
#20248=ADVANCED_FACE ( 'NONE', ( #15450 ), #58012, .T. ) ;
#20251=EDGE_CURVE ( 'NONE', #7998, #12593, #63143, .T. ) ;
#20254=VERTEX_POINT ( 'NONE', #21400 ) ;
#20259=CARTESIAN_POINT ( 'NONE',  ( -21.93488243476846478, -35.49895327440580672, 13.79046412364926333 ) ) ;
#20265=CARTESIAN_POINT ( 'NONE',  ( -68.11501976657856972, 31.41506934893843805, 170.0000000000000000 ) ) ;
#20271=B_SPLINE_CURVE_WITH_KNOTS ( 'NONE', 3,
 ( #20934, #58551, #10368, #31834 ),
 .UNSPECIFIED., .F., .F.,
 ( 4, 4 ),
 ( 0.1259919275528363081, 0.1829744153748759372 ),
 .UNSPECIFIED. ) ;
#20273=VECTOR ( 'NONE', #49190, 1000.000000000000000 ) ;
#20296=EDGE_LOOP ( 'NONE', ( #45452, #35267, #18193, #39783 ) ) ;
#20310=ORIENTED_EDGE ( 'NONE', *, *, #43551, .T. ) ;
#20313=EDGE_CURVE ( 'NONE', #17237, #67632, #68888, .T. ) ;
#20315=CARTESIAN_POINT ( 'NONE',  ( 0.000000000000000000, 0.000000000000000000, 170.0000000000000000 ) ) ;
#20318=LINE ( 'NONE', #14363, #24893 ) ;
#20334=EDGE_CURVE ( 'NONE', #54975, #64346, #46310, .T. ) ;
#20339=CARTESIAN_POINT ( 'NONE',  ( 64.98797965777978902, 1.249999999999979350, 170.0000000000000000 ) ) ;
#20340=DIRECTION ( 'NONE',  ( 0.8584487936018727616, -0.5128992774058949156, 0.000000000000000000 ) ) ;
#20354=AXIS2_PLACEMENT_3D ( 'NONE', #14561, #56428, #61705 ) ;
#20357=CIRCLE ( 'NONE', #1286, 24.99999999999985434 ) ;
#20363=ORIENTED_EDGE ( 'NONE', *, *, #41155, .T. ) ;
#20367=DIRECTION ( 'NONE',  ( 0.9909497617679352555, -0.1342332658176522697, 5.102127870520022769E-18 ) ) ;
#20384=PLANE ( 'NONE',  #53870 ) ;
#20390=DIRECTION ( 'NONE',  ( -0.6910626489868685329, 0.7227948638273878901, 0.000000000000000000 ) ) ;
#20406=ORIENTED_EDGE ( 'NONE', *, *, #29864, .F. ) ;
#20411=AXIS2_PLACEMENT_3D ( 'NONE', #45171, #7558, #46201 ) ;
#20412=CARTESIAN_POINT ( 'NONE',  ( -22.15007195153847164, -31.28689791206514670, 13.32819397642333037 ) ) ;
#20416=VERTEX_POINT ( 'NONE', #32654 ) ;
#20422=CARTESIAN_POINT ( 'NONE',  ( -74.52723870109949189, 7.962625360374199879, 41.38025477438755928 ) ) ;
#20424=EDGE_LOOP ( 'NONE', ( #29848, #3306, #37004, #50191 ) ) ;
#20431=ORIENTED_EDGE ( 'NONE', *, *, #48100, .T. ) ;
#20434=EDGE_LOOP ( 'NONE', ( #3517, #59421, #50911, #42790 ) ) ;
#20436=VERTEX_POINT ( 'NONE', #65015 ) ;
#20439=VECTOR ( 'NONE', #1061, 1000.000000000000000 ) ;
#20444=AXIS2_PLACEMENT_3D ( 'NONE', #2472, #40106, #13377 ) ;
#20451=DIRECTION ( 'NONE',  ( -0.000000000000000000, -0.000000000000000000, -1.000000000000000000 ) ) ;
#20457=VERTEX_POINT ( 'NONE', #6965 ) ;
#20458=VECTOR ( 'NONE', #22087, 1000.000000000000000 ) ;
#20471=ORIENTED_EDGE ( 'NONE', *, *, #67850, .T. ) ;
#20475=DIRECTION ( 'NONE',  ( -0.000000000000000000, -0.000000000000000000, 1.000000000000000000 ) ) ;
#20476=ORIENTED_EDGE ( 'NONE', *, *, #6664, .T. ) ;
#20486=LINE ( 'NONE', #48236, #52102 ) ;
#20489=LINE ( 'NONE', #20156, #34987 ) ;
#20494=CONICAL_SURFACE ( 'NONE', #28381, 74.95140232871122521, 0.8777644062502172329 ) ;
#20496=DIRECTION ( 'NONE',  ( -1.000000000000000000, 0.000000000000000000, 0.000000000000000000 ) ) ;
#20509=DIRECTION ( 'NONE',  ( -0.8090169943749422332, -0.5877852522924802425, 0.000000000000000000 ) ) ;
#20511=CARTESIAN_POINT ( 'NONE',  ( 0.1230226671131348926, -25.12215469714591976, 3.061616997868437868E-16 ) ) ;
#20515=DIRECTION ( 'NONE',  ( -0.5508969814521065267, 0.8345732537212999791, 0.000000000000000000 ) ) ;
#20516=CARTESIAN_POINT ( 'NONE',  ( 74.62299871641495486, 5.461138973199026303, 41.38025477438755928 ) ) ;
#20532=EDGE_CURVE ( 'NONE', #45386, #20826, #60068, .T. ) ;
#20537=DIRECTION ( 'NONE',  ( -1.000000000000000000, 0.000000000000000000, 0.000000000000000000 ) ) ;
#20542=AXIS2_PLACEMENT_3D ( 'NONE', #57252, #67467, #40715 ) ;
#20547=CARTESIAN_POINT ( 'NONE',  ( -14.86595946518020739, 20.25193917588078563, 3.061616997868437868E-16 ) ) ;
#20548=AXIS2_PLACEMENT_3D ( 'NONE', #42129, #42805, #53011 ) ;
#20551=FACE_OUTER_BOUND ( 'NONE', #33044, .T. ) ;
#20556=ORIENTED_EDGE ( 'NONE', *, *, #35558, .F. ) ;
#20558=DIRECTION ( 'NONE',  ( 1.000000000000000000, 0.000000000000000000, 0.000000000000000000 ) ) ;
#20567=ORIENTED_EDGE ( 'NONE', *, *, #61583, .T. ) ;
#20575=EDGE_CURVE ( 'NONE', #66330, #15601, #4783, .T. ) ;
#20577=EDGE_CURVE ( 'NONE', #12758, #56665, #62865, .T. ) ;
#20588=EDGE_LOOP ( 'NONE', ( #8378, #56058, #30527, #59030 ) ) ;
#20589=AXIS2_PLACEMENT_3D ( 'NONE', #35462, #28806, #67827 ) ;
#20599=LINE ( 'NONE', #37823, #53809 ) ;
#20600=CIRCLE ( 'NONE', #17176, 65.00000000000000000 ) ;
#20602=ORIENTED_EDGE ( 'NONE', *, *, #211, .T. ) ;
#20603=VECTOR ( 'NONE', #17225, 1000.000000000000000 ) ;
#20605=ORIENTED_EDGE ( 'NONE', *, *, #17546, .F. ) ;
#20608=B_SPLINE_CURVE_WITH_KNOTS ( 'NONE', 3,
 ( #53012, #9784, #4501, #36861, #69539, #58302 ),
 .UNSPECIFIED., .F., .F.,
 ( 4, 2, 4 ),
 ( 0.03218953612796877223, 0.06469846386257063764, 0.09720739159717248223 ),
 .UNSPECIFIED. ) ;
#20609=DIRECTION ( 'NONE',  ( -0.000000000000000000, 1.000000000000000000, -0.000000000000000000 ) ) ;
#20610=AXIS2_PLACEMENT_3D ( 'NONE', #10274, #16246, #32086 ) ;
#20615=CARTESIAN_POINT ( 'NONE',  ( -15.67984581961064450, 63.08044415722863363, 73.58025477438756923 ) ) ;
#20617=VERTEX_POINT ( 'NONE', #42089 ) ;
#20620=PLANE ( 'NONE',  #43711 ) ;
#20634=CARTESIAN_POINT ( 'NONE',  ( -64.18058723658654685, 10.37664328995176888, 0.000000000000000000 ) ) ;
#20639=EDGE_CURVE ( 'NONE', #8876, #42865, #11020, .T. ) ;
#20653=ORIENTED_EDGE ( 'NONE', *, *, #45268, .T. ) ;
#20660=DIRECTION ( 'NONE',  ( -0.000000000000000000, -0.000000000000000000, -1.000000000000000000 ) ) ;
#20665=CARTESIAN_POINT ( 'NONE',  ( -48.12872802574267439, 43.70867239603707333, 170.0000000000000000 ) ) ;
#20667=CARTESIAN_POINT ( 'NONE',  ( 0.000000000000000000, 0.000000000000000000, 43.58025477438756212 ) ) ;
#20669=EDGE_LOOP ( 'NONE', ( #15832, #41567, #61041, #19896 ) ) ;
#20677=LINE ( 'NONE', #15060, #16521 ) ;
#20679=DIRECTION ( 'NONE',  ( -0.000000000000000000, -0.000000000000000000, 1.000000000000000000 ) ) ;
#20697=VECTOR ( 'NONE', #42304, 1000.000000000000000 ) ;
#20701=B_SPLINE_CURVE_WITH_KNOTS ( 'NONE', 3,
 ( #25187, #67400, #19546, #21193 ),
 .UNSPECIFIED., .F., .F.,
 ( 4, 4 ),
 ( 0.1259919275528358362, 0.1829744153748746882 ),
 .UNSPECIFIED. ) ;
#20703=ORIENTED_EDGE ( 'NONE', *, *, #288, .F. ) ;
#20704=CIRCLE ( 'NONE', #60005, 25.12245591505646303 ) ;
#20712=VECTOR ( 'NONE', #47007, 1000.000000000000000 ) ;
#20714=DIRECTION ( 'NONE',  ( -0.6910626489868685329, 0.7227948638273878901, 0.000000000000000000 ) ) ;
#20715=VERTEX_POINT ( 'NONE', #3871 ) ;
#20727=EDGE_CURVE ( 'NONE', #25681, #40373, #15114, .T. ) ;
#20733=CARTESIAN_POINT ( 'NONE',  ( 35.54014968547571129, -66.04466488925490353, 43.58025477438756212 ) ) ;
#20738=FACE_OUTER_BOUND ( 'NONE', #31244, .T. ) ;
#20741=ORIENTED_EDGE ( 'NONE', *, *, #54438, .F. ) ;
#20743=DIRECTION ( 'NONE',  ( -0.000000000000000000, 0.000000000000000000, -1.000000000000000000 ) ) ;
#20759=DIRECTION ( 'NONE',  ( -1.000000000000000000, 0.000000000000000000, 0.000000000000000000 ) ) ;
#20763=VECTOR ( 'NONE', #3049, 1000.000000000000114 ) ;
#20765=ORIENTED_EDGE ( 'NONE', *, *, #17307, .F. ) ;
#20773=ORIENTED_EDGE ( 'NONE', *, *, #35345, .T. ) ;
#20789=EDGE_CURVE ( 'NONE', #21469, #63543, #55567, .T. ) ;
#20790=ORIENTED_EDGE ( 'NONE', *, *, #5904, .T. ) ;
#20799=VERTEX_POINT ( 'NONE', #47799 ) ;
#20800=AXIS2_PLACEMENT_3D ( 'NONE', #31615, #44940, #2386 ) ;
#20802=DIRECTION ( 'NONE',  ( -0.5508969814520944253, -0.8345732537213078617, 0.000000000000000000 ) ) ;
#20811=CARTESIAN_POINT ( 'NONE',  ( 24.79066879238609644, 3.228426989449657114, 0.000000000000000000 ) ) ;
#20826=VERTEX_POINT ( 'NONE', #4896 ) ;
#20848=VECTOR ( 'NONE', #10993, 1000.000000000000000 ) ;
#20852=LINE ( 'NONE', #42312, #16117 ) ;
#20854=CARTESIAN_POINT ( 'NONE',  ( 11.30618213853385967, 74.15344055032308290, 170.0000000000000000 ) ) ;
#20855=DIRECTION ( 'NONE',  ( -0.000000000000000000, -0.000000000000000000, -1.000000000000000000 ) ) ;
#20858=VECTOR ( 'NONE', #12508, 1000.000000000000000 ) ;
#20859=AXIS2_PLACEMENT_3D ( 'NONE', #58700, #10518, #10867 ) ;
#20871=ORIENTED_EDGE ( 'NONE', *, *, #44553, .F. ) ;
#20893=EDGE_CURVE ( 'NONE', #17738, #53526, #21600, .T. ) ;
#20897=CARTESIAN_POINT ( 'NONE',  ( 21.77974794783310486, 62.98608673099827371, 34.48241795236666007 ) ) ;
#20899=EDGE_LOOP ( 'NONE', ( #32470, #43497, #34862, #15714 ) ) ;
#20909=CARTESIAN_POINT ( 'NONE',  ( -52.13778968636795241, 39.42540649521991014, 6.377659838150125914E-18 ) ) ;
#20910=CARTESIAN_POINT ( 'NONE',  ( 70.34686579112866411, -18.11777090454118877, 43.58025477438756923 ) ) ;
#20919=CARTESIAN_POINT ( 'NONE',  ( 28.03046679490049797, 26.14935035984741774, 13.32819299319723960 ) ) ;
#20925=DIRECTION ( 'NONE',  ( -0.2225209339563184452, 0.9749279121818226201, 0.000000000000000000 ) ) ;
#20930=EDGE_LOOP ( 'NONE', ( #20180, #1452, #59956, #47111 ) ) ;
#20934=CARTESIAN_POINT ( 'NONE',  ( 4.590321433068643486, 24.57496590315240681, 0.000000000000000000 ) ) ;
#20939=FACE_OUTER_BOUND ( 'NONE', #39388, .T. ) ;
#20944=AXIS2_PLACEMENT_3D ( 'NONE', #18338, #39801, #61257 ) ;
#20953=ORIENTED_EDGE ( 'NONE', *, *, #18423, .T. ) ;
#20954=EDGE_LOOP ( 'NONE', ( #62874, #66371, #11247, #2377 ) ) ;
#20965=DIRECTION ( 'NONE',  ( -0.5508969814520944253, -0.8345732537213078617, 0.000000000000000000 ) ) ;
#20969=FACE_OUTER_BOUND ( 'NONE', #19725, .T. ) ;
#20971=CARTESIAN_POINT ( 'NONE',  ( -62.97854483871577713, 16.08424353203677271, 40.00000000000003553 ) ) ;
#20976=EDGE_CURVE ( 'NONE', #11268, #61262, #7686, .T. ) ;
#20985=B_SPLINE_CURVE_WITH_KNOTS ( 'NONE', 3,
 ( #58796, #47899, #5350, #64087 ),
 .UNSPECIFIED., .F., .F.,
 ( 4, 4 ),
 ( 9.900409499072286585E-07, 0.05658314289920114010 ),
 .UNSPECIFIED. ) ;
#21005=ORIENTED_EDGE ( 'NONE', *, *, #31784, .T. ) ;
#21006=VECTOR ( 'NONE', #35469, 1000.000000000000000 ) ;
#21011=CARTESIAN_POINT ( 'NONE',  ( -65.36598343705435354, 0.000000000000000000, 41.38025477438755928 ) ) ;
#21014=AXIS2_PLACEMENT_3D ( 'NONE', #998, #44602, #66082 ) ;
#21017=CARTESIAN_POINT ( 'NONE',  ( 56.42997683260104225, 32.25922681454270702, 170.0000000000000000 ) ) ;
#21024=EDGE_CURVE ( 'NONE', #28566, #26321, #26133, .T. ) ;
#21029=DIRECTION ( 'NONE',  ( -1.000000000000000000, 0.000000000000000000, 0.000000000000000000 ) ) ;
#21034=VERTEX_POINT ( 'NONE', #12260 ) ;
#21040=LINE ( 'NONE', #36526, #17526 ) ;
#21041=ORIENTED_EDGE ( 'NONE', *, *, #35296, .T. ) ;
#21044=VECTOR ( 'NONE', #59014, 1000.000000000000000 ) ;
#21049=AXIS2_PLACEMENT_3D ( 'NONE', #52923, #69106, #52253 ) ;
#21052=ORIENTED_EDGE ( 'NONE', *, *, #51856, .F. ) ;
#21058=AXIS2_PLACEMENT_3D ( 'NONE', #194, #22701, #21654 ) ;
#21063=ORIENTED_EDGE ( 'NONE', *, *, #17155, .T. ) ;
#21077=CARTESIAN_POINT ( 'NONE',  ( -65.36598343705435354, 0.000000000000000000, 41.38025477438755928 ) ) ;
#21084=ORIENTED_EDGE ( 'NONE', *, *, #48041, .T. ) ;
#21108=CIRCLE ( 'NONE', #42434, 74.95140232871122521 ) ;
#21117=CARTESIAN_POINT ( 'NONE',  ( 25.97682081077775251, -21.03539584665513829, 6.893342938366318506 ) ) ;
#21119=AXIS2_PLACEMENT_3D ( 'NONE', #52480, #58105, #25766 ) ;
#21127=DIRECTION ( 'NONE',  ( -0.000000000000000000, -0.000000000000000000, -1.000000000000000000 ) ) ;
#21131=DIRECTION ( 'NONE',  ( 0.8584487936018655452, 0.5128992774059070170, 0.000000000000000000 ) ) ;
#21149=AXIS2_PLACEMENT_3D ( 'NONE', #19661, #41121, #66838 ) ;
#21156=EDGE_CURVE ( 'NONE', #40373, #63617, #35801, .T. ) ;
#21163=ORIENTED_EDGE ( 'NONE', *, *, #25181, .F. ) ;
#21179=LINE ( 'NONE', #9590, #63285 ) ;
#21189=ORIENTED_EDGE ( 'NONE', *, *, #48017, .F. ) ;
#21193=CARTESIAN_POINT ( 'NONE',  ( 64.98797965777978902, -1.250000000000021760, 40.00000000000003553 ) ) ;
#21212=EDGE_CURVE ( 'NONE', #27636, #26875, #64329, .T. ) ;
#21216=LINE ( 'NONE', #21891, #20848 ) ;
#21221=CARTESIAN_POINT ( 'NONE',  ( 57.30278335769541087, 48.40406511297401693, 170.0000000000000000 ) ) ;
#21226=LINE ( 'NONE', #37387, #58941 ) ;
#21234=ORIENTED_EDGE ( 'NONE', *, *, #15473, .F. ) ;
#21235=DIRECTION ( 'NONE',  ( -0.000000000000000000, -0.000000000000000000, -1.000000000000000000 ) ) ;
#21243=ORIENTED_EDGE ( 'NONE', *, *, #31936, .T. ) ;
#21253=VERTEX_POINT ( 'NONE', #41074 ) ;
#21254=VERTEX_POINT ( 'NONE', #51968 ) ;
#21255=CARTESIAN_POINT ( 'NONE',  ( 64.08056813503695537, 12.89932471814515225, 41.38025477438755928 ) ) ;
#21261=DIRECTION ( 'NONE',  ( -0.000000000000000000, -0.000000000000000000, 1.000000000000000000 ) ) ;
#21264=ORIENTED_EDGE ( 'NONE', *, *, #6364, .T. ) ;
#21270=B_SPLINE_CURVE_WITH_KNOTS ( 'NONE', 3,
 ( #47454, #30962, #58361, #4226, #47121, #52735 ),
 .UNSPECIFIED., .F., .F.,
 ( 4, 2, 4 ),
 ( 0.03218947840871067695, 0.06469842185262320022, 0.09720736529653573044 ),
 .UNSPECIFIED. ) ;
#21272=DIRECTION ( 'NONE',  ( -0.04486483035051862939, 0.9989930665413143673, 0.000000000000000000 ) ) ;
#21285=EDGE_CURVE ( 'NONE', #62629, #53534, #48059, .T. ) ;
#21287=ORIENTED_EDGE ( 'NONE', *, *, #9693, .F. ) ;
#21295=ORIENTED_EDGE ( 'NONE', *, *, #53514, .F. ) ;
#21299=ORIENTED_EDGE ( 'NONE', *, *, #14837, .F. ) ;
#21325=DIRECTION ( 'NONE',  ( -0.000000000000000000, -0.000000000000000000, -1.000000000000000000 ) ) ;
#21329=VERTEX_POINT ( 'NONE', #58615 ) ;
#21331=CARTESIAN_POINT ( 'NONE',  ( 69.77839676787858991, 27.52340539440040956, 170.0000000000000000 ) ) ;
#21344=ORIENTED_EDGE ( 'NONE', *, *, #40258, .F. ) ;
#21346=CARTESIAN_POINT ( 'NONE',  ( -33.97702052856965338, 17.74986603947969144, 13.32819397642332504 ) ) ;
#21356=CARTESIAN_POINT ( 'NONE',  ( 35.38849253846352383, 46.38061039241811301, 27.58472369417912162 ) ) ;
#21358=LINE ( 'NONE', #4500, #25046 ) ;
#21365=EDGE_CURVE ( 'NONE', #66442, #42365, #55394, .T. ) ;
#21376=VERTEX_POINT ( 'NONE', #69172 ) ;
#21377=LINE ( 'NONE', #59687, #31146 ) ;
#21381=LINE ( 'NONE', #64296, #25682 ) ;
#21391=CARTESIAN_POINT ( 'NONE',  ( 56.42997683260146857, -32.25922681454192542, 170.0000000000000000 ) ) ;
#21399=DIRECTION ( 'NONE',  ( -0.000000000000000000, -0.000000000000000000, -1.000000000000000000 ) ) ;
#21400=CARTESIAN_POINT ( 'NONE',  ( 55.46196446482127840, -34.59309596431295120, 43.58025477438756212 ) ) ;
#21401=ORIENTED_EDGE ( 'NONE', *, *, #26599, .F. ) ;
#21405=EDGE_CURVE ( 'NONE', #68305, #68932, #31899, .T. ) ;
#21406=LINE ( 'NONE', #64319, #34265 ) ;
#21415=DIRECTION ( 'NONE',  ( -0.000000000000000000, -0.000000000000000000, -1.000000000000000000 ) ) ;
#21418=DIRECTION ( 'NONE',  ( -0.000000000000000000, -0.000000000000000000, -1.000000000000000000 ) ) ;
#21419=EDGE_CURVE ( 'NONE', #19763, #31093, #21679, .T. ) ;
#21433=EDGE_CURVE ( 'NONE', #3016, #60863, #53120, .T. ) ;
#21437=CARTESIAN_POINT ( 'NONE',  ( 45.82394788922869822, -46.11928342727429708, 41.38025477438755928 ) ) ;
#21438=ORIENTED_EDGE ( 'NONE', *, *, #14115, .T. ) ;
#21445=VERTEX_POINT ( 'NONE', #66703 ) ;
#21450=EDGE_CURVE ( 'NONE', #22781, #23405, #60976, .T. ) ;
#21451=LINE ( 'NONE', #64357, #42382 ) ;
#21459=DIRECTION ( 'NONE',  ( 1.000000000000000000, 0.000000000000000000, 0.000000000000000000 ) ) ;
#21460=EDGE_LOOP ( 'NONE', ( #15282, #53884, #62575, #61572, #1954, #40214, #43773, #53919, #22993 ) ) ;
#21469=VERTEX_POINT ( 'NONE', #56128 ) ;
#21481=DIRECTION ( 'NONE',  ( 0.8584487936018727616, -0.5128992774058949156, 0.000000000000000000 ) ) ;
#21483=DIRECTION ( 'NONE',  ( 1.000000000000000000, 0.000000000000000000, 0.000000000000000000 ) ) ;
#21484=CARTESIAN_POINT ( 'NONE',  ( -28.32746765835430836, -69.45586423092646555, 170.0000000000000000 ) ) ;
#21489=VECTOR ( 'NONE', #32532, 1000.000000000000000 ) ;
#21494=CARTESIAN_POINT ( 'NONE',  ( -84.49322488516129681, 0.000000000000000000, 43.58025477438756212 ) ) ;
#21496=CARTESIAN_POINT ( 'NONE',  ( -64.83840629396348731, 4.580509716059292913, 40.00000000000003553 ) ) ;
#21497=CARTESIAN_POINT ( 'NONE',  ( 6.526941389886052214, 24.13294503563511029, 0.000000000000000000 ) ) ;
#21522=EDGE_LOOP ( 'NONE', ( #4725, #15252, #36070, #43614 ) ) ;
#21529=EDGE_CURVE ( 'NONE', #68932, #4035, #51481, .T. ) ;
#21538=LINE ( 'NONE', #10985, #64735 ) ;
#21542=AXIS2_PLACEMENT_3D ( 'NONE', #45788, #55639, #67266 ) ;
#21548=ORIENTED_EDGE ( 'NONE', *, *, #5009, .T. ) ;
#21552=CIRCLE ( 'NONE', #30565, 65.00000000000000000 ) ;
#21553=AXIS2_PLACEMENT_3D ( 'NONE', #53097, #9179, #4925 ) ;
#21555=DIRECTION ( 'NONE',  ( -0.9009688679024218105, 0.4338837391175526248, 0.000000000000000000 ) ) ;
#21565=CARTESIAN_POINT ( 'NONE',  ( 34.76618902119821541, -54.93755186520709799, 43.58025477438756923 ) ) ;
#21566=ADVANCED_FACE ( 'NONE', ( #17087 ), #49761, .T. ) ;
#21572=LINE ( 'NONE', #1168, #58505 ) ;
#21587=EDGE_LOOP ( 'NONE', ( #11226, #23255, #14120, #11818 ) ) ;
#21589=ORIENTED_EDGE ( 'NONE', *, *, #13101, .T. ) ;
#21593=EDGE_CURVE ( 'NONE', #47929, #17237, #9311, .T. ) ;
#21594=FACE_OUTER_BOUND ( 'NONE', #64207, .T. ) ;
#21595=VECTOR ( 'NONE', #48867, 999.9999999999998863 ) ;
#21599=ADVANCED_FACE ( 'NONE', ( #62798 ), #45573, .T. ) ;
#21600=CIRCLE ( 'NONE', #14878, 24.99999999999985434 ) ;
#21604=VERTEX_POINT ( 'NONE', #35726 ) ;
#21605=VERTEX_POINT ( 'NONE', #40300 ) ;
#21616=SHAPE_REPRESENTATION_RELATIONSHIP ( 'NONE' , 'NONE' ,  #55473, #60914 ) ;
#21619=CARTESIAN_POINT ( 'NONE',  ( 56.74421265833604622, -32.44697398030825752, 41.38025477438755928 ) ) ;
#21648=AXIS2_PLACEMENT_3D ( 'NONE', #60000, #61059, #49443 ) ;
#21654=DIRECTION ( 'NONE',  ( -1.000000000000000000, 0.000000000000000000, 0.000000000000000000 ) ) ;
#21679=LINE ( 'NONE', #26621, #3683 ) ;
#21682=CARTESIAN_POINT ( 'NONE',  ( 4.606779575613957789, 24.69646479044443765, 0.000000000000000000 ) ) ;
#21685=EDGE_LOOP ( 'NONE', ( #42353, #32502, #15540, #29956 ) ) ;
#21687=ORIENTED_EDGE ( 'NONE', *, *, #67594, .T. ) ;
#21696=LINE ( 'NONE', #58981, #25908 ) ;
#21703=CARTESIAN_POINT ( 'NONE',  ( 18.89356949897823768, 62.19351277735707839, 133.5802547743875550 ) ) ;
#21711=ORIENTED_EDGE ( 'NONE', *, *, #56949, .T. ) ;
#21728=DIRECTION ( 'NONE',  ( -1.000000000000000000, -1.509903313490212895E-14, 2.135044278125301096E-16 ) ) ;
#21729=EDGE_LOOP ( 'NONE', ( #30399, #15741, #9242, #9197, #68879, #61829, #55271, #28270, #38481 ) ) ;
#21734=CIRCLE ( 'NONE', #2627, 65.00000000000000000 ) ;
#21737=CARTESIAN_POINT ( 'NONE',  ( -61.34830047412111043, 62.92641549729705019, 133.5802547743875550 ) ) ;
#21744=ORIENTED_EDGE ( 'NONE', *, *, #17716, .T. ) ;
#21745=PLANE ( 'NONE',  #12027 ) ;
#21748=DIRECTION ( 'NONE',  ( -0.000000000000000000, -0.000000000000000000, -1.000000000000000000 ) ) ;
#21753=ORIENTED_EDGE ( 'NONE', *, *, #28085, .F. ) ;
#21754=ORIENTED_EDGE ( 'NONE', *, *, #30028, .T. ) ;
#21758=CARTESIAN_POINT ( 'NONE',  ( 24.96873044429757726, 1.250000000000021982, 0.000000000000000000 ) ) ;
#21763=DIRECTION ( 'NONE',  ( 0.3090169943749447312, 0.9510565162951544194, 0.000000000000000000 ) ) ;
#21766=VERTEX_POINT ( 'NONE', #1908 ) ;
#21769=CARTESIAN_POINT ( 'NONE',  ( -29.87147652227455552, -74.98256102853682137, 133.5802547743875550 ) ) ;
#21771=DIRECTION ( 'NONE',  ( -0.000000000000000000, -0.000000000000000000, -1.000000000000000000 ) ) ;
#21778=FACE_OUTER_BOUND ( 'NONE', #36393, .T. ) ;
#21780=ORIENTED_EDGE ( 'NONE', *, *, #13762, .T. ) ;
#21781=ORIENTED_EDGE ( 'NONE', *, *, #42084, .T. ) ;
#21788=VERTEX_POINT ( 'NONE', #60631 ) ;
#21792=ORIENTED_EDGE ( 'NONE', *, *, #6424, .T. ) ;
#21801=EDGE_CURVE ( 'NONE', #38858, #27926, #54287, .T. ) ;
#21802=AXIS2_PLACEMENT_3D ( 'NONE', #3160, #35153, #24961 ) ;
#21808=DIRECTION ( 'NONE',  ( -0.000000000000000000, -0.000000000000000000, -1.000000000000000000 ) ) ;
#21812=ADVANCED_FACE ( 'NONE', ( #17730 ), #46461, .T. ) ;
#21818=EDGE_LOOP ( 'NONE', ( #24784, #22468, #5976, #57845 ) ) ;
#21827=AXIS2_PLACEMENT_3D ( 'NONE', #56813, #66688, #49776 ) ;
#21828=CARTESIAN_POINT ( 'NONE',  ( 23.81581464765709200, 7.603089679099848119, 0.000000000000000000 ) ) ;
#21829=DIRECTION ( 'NONE',  ( -0.000000000000000000, -0.000000000000000000, -1.000000000000000000 ) ) ;
#21830=CARTESIAN_POINT ( 'NONE',  ( -84.49322488516129681, 0.000000000000000000, 43.58025477438756212 ) ) ;
#21856=CIRCLE ( 'NONE', #28601, 24.99999999999985434 ) ;
#21869=ORIENTED_EDGE ( 'NONE', *, *, #13358, .F. ) ;
#21879=CARTESIAN_POINT ( 'NONE',  ( -58.33959211650994092, -29.48226216511403308, 43.58025477438756212 ) ) ;
#21881=CARTESIAN_POINT ( 'NONE',  ( 0.000000000000000000, 0.000000000000000000, 0.000000000000000000 ) ) ;
#21891=CARTESIAN_POINT ( 'NONE',  ( 45.82394788922800899, 46.11928342727495078, 43.58025477438756923 ) ) ;
#21897=DIRECTION ( 'NONE',  ( -2.998955517602105048E-18, 4.127708154724731195E-18, -1.000000000000000000 ) ) ;
#21905=DIRECTION ( 'NONE',  ( -0.3513748240813435175, 0.9362348706397369824, 2.500042656554809354E-16 ) ) ;
#21917=DIRECTION ( 'NONE',  ( -0.5508969814520946473, -0.8345732537213079727, 0.000000000000000000 ) ) ;
#21922=EDGE_LOOP ( 'NONE', ( #9145, #1230, #54736, #6772 ) ) ;
#21925=EDGE_CURVE ( 'NONE', #53544, #6513, #11078, .T. ) ;
#21930=CARTESIAN_POINT ( 'NONE',  ( -84.49322488516129681, 0.000000000000000000, 43.58025477438756212 ) ) ;
#21937=AXIS2_PLACEMENT_3D ( 'NONE', #57326, #67541, #41149 ) ;
#21941=DIRECTION ( 'NONE',  ( 0.000000000000000000, 0.000000000000000000, 1.000000000000000000 ) ) ;
#21946=VECTOR ( 'NONE', #53346, 1000.000000000000000 ) ;
#21961=VERTEX_POINT ( 'NONE', #29488 ) ;
#21968=CARTESIAN_POINT ( 'NONE',  ( 0.000000000000000000, 0.000000000000000000, 40.00000000000003553 ) ) ;
#21972=ORIENTED_EDGE ( 'NONE', *, *, #16110, .T. ) ;
#21976=CYLINDRICAL_SURFACE ( 'NONE', #39934, 65.00000000000000000 ) ;
#21978=CARTESIAN_POINT ( 'NONE',  ( -59.42430146430388049, -27.22983999535795618, 43.58025477438756212 ) ) ;
#21984=EDGE_CURVE ( 'NONE', #18463, #20826, #12979, .T. ) ;
#21987=AXIS2_PLACEMENT_3D ( 'NONE', #23431, #45912, #34330 ) ;
#21989=FACE_OUTER_BOUND ( 'NONE', #14026, .T. ) ;
#21991=CARTESIAN_POINT ( 'NONE',  ( -74.58602291351357394, -7.967916035252095242, 170.0000000000000000 ) ) ;
#21995=EDGE_CURVE ( 'NONE', #863, #56212, #3737, .T. ) ;
#22001=VECTOR ( 'NONE', #59253, 1000.000000000000000 ) ;
#22019=DIRECTION ( 'NONE',  ( -1.000000000000000000, 0.000000000000000000, 0.000000000000000000 ) ) ;
#22020=ADVANCED_FACE ( 'NONE', ( #34086 ), #11598, .F. ) ;
#22025=DIRECTION ( 'NONE',  ( -1.000000000000000000, 0.000000000000000000, 0.000000000000000000 ) ) ;
#22033=CARTESIAN_POINT ( 'NONE',  ( -84.49322488516129681, 0.000000000000000000, 43.58025477438756212 ) ) ;
#22039=ORIENTED_EDGE ( 'NONE', *, *, #41921, .F. ) ;
#22043=CARTESIAN_POINT ( 'NONE',  ( 36.64089410029661309, -65.45232906116366678, 170.0000000000000000 ) ) ;
#22050=DIRECTION ( 'NONE',  ( -0.000000000000000000, 0.000000000000000000, -1.000000000000000000 ) ) ;
#22065=ORIENTED_EDGE ( 'NONE', *, *, #55850, .T. ) ;
#22080=ORIENTED_EDGE ( 'NONE', *, *, #44321, .F. ) ;
#22083=EDGE_CURVE ( 'NONE', #58443, #64743, #9772, .T. ) ;
#22087=DIRECTION ( 'NONE',  ( 2.086468734322990096E-16, 1.377265952997550087E-16, 1.000000000000000000 ) ) ;
#22088=VERTEX_POINT ( 'NONE', #47049 ) ;
#22093=AXIS2_PLACEMENT_3D ( 'NONE', #35129, #45691, #61173 ) ;
#22101=AXIS2_PLACEMENT_3D ( 'NONE', #52827, #41596, #3971 ) ;
#22102=CARTESIAN_POINT ( 'NONE',  ( -23.85457283326427813, -7.880174245944393974, 3.061616997868437868E-16 ) ) ;
#22107=ORIENTED_EDGE ( 'NONE', *, *, #65920, .F. ) ;
#22116=CARTESIAN_POINT ( 'NONE',  ( -13.24252603915608617, 63.63674649211943546, 40.00000000000003553 ) ) ;
#22117=CARTESIAN_POINT ( 'NONE',  ( -61.29635759142584561, -21.66977272663583776, 170.0000000000000000 ) ) ;
#22125=DIRECTION ( 'NONE',  ( 0.4738686624730094610, -0.8805955318567321166, 0.000000000000000000 ) ) ;
#22130=DIRECTION ( 'NONE',  ( 0.000000000000000000, 0.000000000000000000, 1.000000000000000000 ) ) ;
#22131=VERTEX_POINT ( 'NONE', #68836 ) ;
#22141=CIRCLE ( 'NONE', #34524, 65.00000000000000000 ) ;
#22142=DIRECTION ( 'NONE',  ( -1.000000000000000000, 0.000000000000000000, 0.000000000000000000 ) ) ;
#22149=PLANE ( 'NONE',  #19953 ) ;
#22150=VECTOR ( 'NONE', #49756, 1000.000000000000000 ) ;
#22154=ADVANCED_FACE ( 'NONE', ( #57615 ), #68508, .T. ) ;
#22164=ORIENTED_EDGE ( 'NONE', *, *, #32388, .T. ) ;
#22167=CARTESIAN_POINT ( 'NONE',  ( 18.07314801315378006, 17.44990292519104003, 3.061616997868437868E-16 ) ) ;
#22183=LINE ( 'NONE', #43969, #28953 ) ;
#22185=VECTOR ( 'NONE', #51902, 1000.000000000000114 ) ;
#22188=CARTESIAN_POINT ( 'NONE',  ( 0.000000000000000000, 0.000000000000000000, 40.00000000000003553 ) ) ;
#22191=ORIENTED_EDGE ( 'NONE', *, *, #21024, .F. ) ;
#22223=ORIENTED_EDGE ( 'NONE', *, *, #7394, .F. ) ;
#22224=ORIENTED_EDGE ( 'NONE', *, *, #6174, .T. ) ;
#22229=CARTESIAN_POINT ( 'NONE',  ( 0.000000000000000000, 0.000000000000000000, 41.38025477438755928 ) ) ;
#22239=DIRECTION ( 'NONE',  ( -0.000000000000000000, -0.000000000000000000, -1.000000000000000000 ) ) ;
#22254=CONICAL_SURFACE ( 'NONE', #61578, 74.95140232871122521, 0.8777644062502172329 ) ;
#22259=AXIS2_PLACEMENT_3D ( 'NONE', #18497, #19180, #44882 ) ;
#22279=ORIENTED_EDGE ( 'NONE', *, *, #17286, .F. ) ;
#22288=CARTESIAN_POINT ( 'NONE',  ( 0.000000000000000000, 0.000000000000000000, 40.00000000000003553 ) ) ;
#22293=ORIENTED_EDGE ( 'NONE', *, *, #11568, .F. ) ;
#22294=EDGE_LOOP ( 'NONE', ( #22774, #33524, #57961, #19936, #51433, #26105, #62640, #48526, #65525 ) ) ;
#22305=EDGE_CURVE ( 'NONE', #60309, #44366, #591, .T. ) ;
#22308=EDGE_CURVE ( 'NONE', #28214, #14673, #50172, .T. ) ;
#22309=DIRECTION ( 'NONE',  ( 0.8090169943749506709, -0.5877852522924686962, 0.000000000000000000 ) ) ;
#22323=DIRECTION ( 'NONE',  ( 1.000000000000000000, 0.000000000000000000, 0.000000000000000000 ) ) ;
#22325=ORIENTED_EDGE ( 'NONE', *, *, #28250, .T. ) ;
#22326=LINE ( 'NONE', #64897, #49555 ) ;
#22339=DIRECTION ( 'NONE',  ( 0.000000000000000000, 0.000000000000000000, 1.000000000000000000 ) ) ;
#22341=VERTEX_POINT ( 'NONE', #39279 ) ;
#22342=CARTESIAN_POINT ( 'NONE',  ( 41.49663191311417165, -50.03028622612021792, 170.0000000000000000 ) ) ;
#22345=LINE ( 'NONE', #54694, #68294 ) ;
#22346=VECTOR ( 'NONE', #49753, 1000.000000000000114 ) ;
#22350=CARTESIAN_POINT ( 'NONE',  ( -44.00727179482577611, 47.83680621839560132, 40.00000000000003553 ) ) ;
#22354=ORIENTED_EDGE ( 'NONE', *, *, #61698, .T. ) ;
#22369=DIRECTION ( 'NONE',  ( -0.000000000000000000, 0.000000000000000000, -1.000000000000000000 ) ) ;
#22377=CARTESIAN_POINT ( 'NONE',  ( 10.06749493632391967, 74.32123213259514216, 0.000000000000000000 ) ) ;
#22378=CARTESIAN_POINT ( 'NONE',  ( -15.24379664668640899, 38.84509419542018094, 13.79046340968178441 ) ) ;
#22379=CARTESIAN_POINT ( 'NONE',  ( -49.77357484059128012, -41.82599373102878104, 170.0000000000000000 ) ) ;
#22385=ORIENTED_EDGE ( 'NONE', *, *, #55416, .T. ) ;
#22387=ORIENTED_EDGE ( 'NONE', *, *, #40258, .T. ) ;
#22390=EDGE_CURVE ( 'NONE', #64497, #37048, #1290, .T. ) ;
#22400=DIRECTION ( 'NONE',  ( -0.000000000000000000, -0.000000000000000000, -1.000000000000000000 ) ) ;
#22407=CARTESIAN_POINT ( 'NONE',  ( -24.39249304643438521, 60.24953346690454481, 40.00000000000003553 ) ) ;
#22422=EDGE_CURVE ( 'NONE', #37971, #35286, #35268, .T. ) ;
#22426=CARTESIAN_POINT ( 'NONE',  ( -63.73419499958981049, -12.83646726144931449, 170.0000000000000000 ) ) ;
#22437=VERTEX_POINT ( 'NONE', #46620 ) ;
#22443=FACE_OUTER_BOUND ( 'NONE', #66536, .T. ) ;
#22456=EDGE_LOOP ( 'NONE', ( #3155, #54342, #1046, #58446, #44332, #19503, #16705, #23206, #47895 ) ) ;
#22457=VERTEX_POINT ( 'NONE', #57532 ) ;
#22458=CIRCLE ( 'NONE', #20209, 24.99999999999985434 ) ;
#22466=ADVANCED_FACE ( 'NONE', ( #30799 ), #52247, .T. ) ;
#22468=ORIENTED_EDGE ( 'NONE', *, *, #67454, .F. ) ;
#22469=DIRECTION ( 'NONE',  ( -1.000000000000000000, 0.000000000000000000, 0.000000000000000000 ) ) ;
#22476=CARTESIAN_POINT ( 'NONE',  ( -29.70166638324963415, 57.83280658984260469, 3.061616997868437868E-16 ) ) ;
#22497=VECTOR ( 'NONE', #65261, 1000.000000000000114 ) ;
#22498=CARTESIAN_POINT ( 'NONE',  ( -19.46539569203835640, 15.68752276659279943, 0.000000000000000000 ) ) ;
#22501=CARTESIAN_POINT ( 'NONE',  ( -49.77357484059128012, -41.82599373102878104, 170.0000000000000000 ) ) ;
#22504=CARTESIAN_POINT ( 'NONE',  ( 0.000000000000000000, 0.000000000000000000, 0.000000000000000000 ) ) ;
#22510=CARTESIAN_POINT ( 'NONE',  ( -84.49322488516129681, 0.000000000000000000, 43.58025477438756212 ) ) ;
#22512=DIRECTION ( 'NONE',  ( -1.000000000000000000, 0.000000000000000000, 0.000000000000000000 ) ) ;
#22524=VECTOR ( 'NONE', #59238, 1000.000000000000000 ) ;
#22537=DIRECTION ( 'NONE',  ( 1.000000000000000000, 0.000000000000000000, 0.000000000000000000 ) ) ;
#22547=CARTESIAN_POINT ( 'NONE',  ( 20.79325243092002751, 13.87950479462545772, 0.000000000000000000 ) ) ;
#22549=CARTESIAN_POINT ( 'NONE',  ( 29.69502258243350923, 57.82046033912877903, 40.00000000000003553 ) ) ;
#22550=CARTESIAN_POINT ( 'NONE',  ( 32.24915330809657377, -20.72408693595937734, 13.32819397642332326 ) ) ;
#22564=AXIS2_PLACEMENT_3D ( 'NONE', #58143, #56766, #57797 ) ;
#22570=VERTEX_POINT ( 'NONE', #28637 ) ;
#22574=B_SPLINE_CURVE_WITH_KNOTS ( 'NONE', 3,
 ( #49545, #17192, #65760, #65051 ),
 .UNSPECIFIED., .F., .F.,
 ( 4, 4 ),
 ( 9.900409499083079903E-07, 0.05658314289920115397 ),
 .UNSPECIFIED. ) ;
#22575=AXIS2_PLACEMENT_3D ( 'NONE', #47608, #30767, #69061 ) ;
#22577=DIRECTION ( 'NONE',  ( -1.000000000000000000, 0.000000000000000000, 0.000000000000000000 ) ) ;
#22580=ORIENTED_EDGE ( 'NONE', *, *, #15817, .F. ) ;
#22589=VERTEX_POINT ( 'NONE', #12458 ) ;
#22590=LINE ( 'NONE', #44030, #44749 ) ;
#22593=CARTESIAN_POINT ( 'NONE',  ( 34.76618902119740540, 54.93755186520760958, 41.38025477438755928 ) ) ;
#22594=DIRECTION ( 'NONE',  ( -0.000000000000000000, -0.000000000000000000, -1.000000000000000000 ) ) ;
#22598=DIRECTION ( 'NONE',  ( -0.000000000000000000, -0.000000000000000000, -1.000000000000000000 ) ) ;
#22601=ORIENTED_EDGE ( 'NONE', *, *, #56275, .T. ) ;
#22603=LINE ( 'NONE', #54604, #69196 ) ;
#22608=LINE ( 'NONE', #1156, #10540 ) ;
#22612=DIRECTION ( 'NONE',  ( 0.000000000000000000, 0.000000000000000000, 1.000000000000000000 ) ) ;
#22616=CIRCLE ( 'NONE', #9176, 74.95140232871122521 ) ;
#22625=VERTEX_POINT ( 'NONE', #54658 ) ;
#22629=ORIENTED_EDGE ( 'NONE', *, *, #26229, .T. ) ;
#22639=FACE_OUTER_BOUND ( 'NONE', #4931, .T. ) ;
#22641=VERTEX_POINT ( 'NONE', #24411 ) ;
#22643=CARTESIAN_POINT ( 'NONE',  ( -37.26544890750056283, -8.987879958075955855, 13.32819397642332682 ) ) ;
#22645=DIRECTION ( 'NONE',  ( 0.5508969814521065267, -0.8345732537212999791, 0.000000000000000000 ) ) ;
#22646=CARTESIAN_POINT ( 'NONE',  ( -21.27554331372999741, 61.43430442924864820, 170.0000000000000000 ) ) ;
#22647=EDGE_CURVE ( 'NONE', #44455, #20799, #30719, .T. ) ;
#22654=CARTESIAN_POINT ( 'NONE',  ( -10.00000000000000000, 0.000000000000000000, 170.0010000000000048 ) ) ;
#22662=ORIENTED_EDGE ( 'NONE', *, *, #35754, .T. ) ;
#22695=CARTESIAN_POINT ( 'NONE',  ( 69.68177367721139603, 20.52767805628179687, 0.000000000000000000 ) ) ;
#22701=DIRECTION ( 'NONE',  ( -0.000000000000000000, -0.000000000000000000, -1.000000000000000000 ) ) ;
#22709=CIRCLE ( 'NONE', #59744, 65.00000000000000000 ) ;
#22711=EDGE_CURVE ( 'NONE', #58737, #49213, #69018, .T. ) ;
#22716=CARTESIAN_POINT ( 'NONE',  ( 24.96873044429757726, 1.250000000000021982, 0.000000000000000000 ) ) ;
#22726=EDGE_CURVE ( 'NONE', #65848, #60623, #32092, .T. ) ;
#22732=EDGE_CURVE ( 'NONE', #28312, #33243, #64443, .T. ) ;
#22733=ADVANCED_FACE ( 'NONE', ( #47223 ), #4936, .T. ) ;
#22740=DIRECTION ( 'NONE',  ( -0.000000000000000000, -0.000000000000000000, 1.000000000000000000 ) ) ;
#22747=CARTESIAN_POINT ( 'NONE',  ( 45.74764628539747235, 59.37057832282332726, 41.38025477438755928 ) ) ;
#22752=DIRECTION ( 'NONE',  ( 1.000000000000000000, 0.000000000000000000, 0.000000000000000000 ) ) ;
#22768=CARTESIAN_POINT ( 'NONE',  ( -26.69131247781221106, -59.26697088777007849, 40.00000000000003553 ) ) ;
#22774=ORIENTED_EDGE ( 'NONE', *, *, #12386, .F. ) ;
#22780=CARTESIAN_POINT ( 'NONE',  ( 0.000000000000000000, 0.000000000000000000, 170.0000000000000000 ) ) ;
#22781=VERTEX_POINT ( 'NONE', #68682 ) ;
#22792=ORIENTED_EDGE ( 'NONE', *, *, #28772, .F. ) ;
#22797=ORIENTED_EDGE ( 'NONE', *, *, #55831, .T. ) ;
#22798=CARTESIAN_POINT ( 'NONE',  ( 10.06749493632391967, 74.32123213259514216, 0.000000000000000000 ) ) ;
#22799=CARTESIAN_POINT ( 'NONE',  ( -29.87147652227456263, 68.79592317125366208, 73.58025477438755502 ) ) ;
#22802=DIRECTION ( 'NONE',  ( -1.000000000000000000, 0.000000000000000000, 0.000000000000000000 ) ) ;
#22808=EDGE_CURVE ( 'NONE', #32020, #6977, #60558, .T. ) ;
#22814=EDGE_CURVE ( 'NONE', #1146, #68932, #40886, .T. ) ;
#22815=DIRECTION ( 'NONE',  ( 0.000000000000000000, 0.000000000000000000, -1.000000000000000000 ) ) ;
#22816=CARTESIAN_POINT ( 'NONE',  ( 24.33197424463712011, -22.91807472895442999, 6.893343212288945310 ) ) ;
#22824=ORIENTED_EDGE ( 'NONE', *, *, #59299, .T. ) ;
#22825=CARTESIAN_POINT ( 'NONE',  ( 63.69186821587121017, 39.51023455020778385, 41.38025477438755928 ) ) ;
#22832=DIRECTION ( 'NONE',  ( -0.000000000000000000, -0.000000000000000000, -1.000000000000000000 ) ) ;
#22836=CARTESIAN_POINT ( 'NONE',  ( -42.36049017605873956, -61.90437280228297112, 170.0000000000000000 ) ) ;
#22837=LINE ( 'NONE', #7367, #62120 ) ;
#22843=ORIENTED_EDGE ( 'NONE', *, *, #52571, .T. ) ;
#22851=EDGE_LOOP ( 'NONE', ( #53701, #37494, #52398, #6694 ) ) ;
#22856=VERTEX_POINT ( 'NONE', #17294 ) ;
#22857=CARTESIAN_POINT ( 'NONE',  ( -84.49322488516129681, 0.000000000000000000, 43.58025477438756212 ) ) ;
#22873=AXIS2_PLACEMENT_3D ( 'NONE', #33776, #55926, #34126 ) ;
#22880=LINE ( 'NONE', #43623, #2491 ) ;
#22900=EDGE_CURVE ( 'NONE', #14951, #61903, #35568, .T. ) ;
#22901=CARTESIAN_POINT ( 'NONE',  ( 0.000000000000000000, 0.000000000000000000, 0.000000000000000000 ) ) ;
#22902=DIRECTION ( 'NONE',  ( -1.000000000000000000, 0.000000000000000000, 0.000000000000000000 ) ) ;
#22903=CARTESIAN_POINT ( 'NONE',  ( 33.40240440333036531, -1.250000000000021982, 6.893343212288935540 ) ) ;
#22909=ORIENTED_EDGE ( 'NONE', *, *, #12539, .F. ) ;
#22916=PLANE ( 'NONE',  #6344 ) ;
#22919=DIRECTION ( 'NONE',  ( -4.852411958229163333E-18, -1.576644219464802818E-18, -1.000000000000000000 ) ) ;
#22920=ORIENTED_EDGE ( 'NONE', *, *, #34778, .F. ) ;
#22928=LINE ( 'NONE', #39121, #4639 ) ;
#22929=AXIS2_PLACEMENT_3D ( 'NONE', #45631, #46304, #34397 ) ;
#22949=DIRECTION ( 'NONE',  ( -0.5508969814520944253, -0.8345732537213078617, 0.000000000000000000 ) ) ;
#22952=VERTEX_POINT ( 'NONE', #7798 ) ;
#22956=ORIENTED_EDGE ( 'NONE', *, *, #11464, .T. ) ;
#22970=CONICAL_SURFACE ( 'NONE', #31955, 74.95140232871122521, 0.8777644062502172329 ) ;
#22973=AXIS2_PLACEMENT_3D ( 'NONE', #55304, #21905, #43352 ) ;
#22976=VECTOR ( 'NONE', #20609, 1000.000000000000000 ) ;
#22978=DIRECTION ( 'NONE',  ( -0.000000000000000000, -0.000000000000000000, -1.000000000000000000 ) ) ;
#22993=ORIENTED_EDGE ( 'NONE', *, *, #35296, .F. ) ;
#22994=CARTESIAN_POINT ( 'NONE',  ( -65.00200000000002376, 1.249999999999979350, 170.0000000000000000 ) ) ;
#22996=ORIENTED_EDGE ( 'NONE', *, *, #9693, .T. ) ;
#23002=DIRECTION ( 'NONE',  ( -1.000000000000000000, 0.000000000000000000, 0.000000000000000000 ) ) ;
#23013=CARTESIAN_POINT ( 'NONE',  ( 70.34686579112810989, 18.11777090454213379, 41.38025477438755928 ) ) ;
#23016=AXIS2_PLACEMENT_3D ( 'NONE', #38112, #68735, #59556 ) ;
#23027=PLANE ( 'NONE',  #64681 ) ;
#23033=B_SPLINE_CURVE_WITH_KNOTS ( 'NONE', 3,
 ( #20547, #52222, #47619, #68412, #32155, #69071 ),
 .UNSPECIFIED., .F., .F.,
 ( 4, 2, 4 ),
 ( 0.03218943375184182137, 0.06469838935233371280, 0.09720734495282559728 ),
 .UNSPECIFIED. ) ;
#23035=EDGE_CURVE ( 'NONE', #61402, #16881, #35914, .T. ) ;
#23039=DIRECTION ( 'NONE',  ( -0.000000000000000000, -0.000000000000000000, -1.000000000000000000 ) ) ;
#23048=CARTESIAN_POINT ( 'NONE',  ( 0.000000000000000000, 0.000000000000000000, 40.00000000000003553 ) ) ;
#23057=ORIENTED_EDGE ( 'NONE', *, *, #67437, .F. ) ;
#23058=CARTESIAN_POINT ( 'NONE',  ( 74.01791526339567895, -12.16185512414844716, 170.0000000000000000 ) ) ;
#23062=FACE_OUTER_BOUND ( 'NONE', #62793, .T. ) ;
#23063=CIRCLE ( 'NONE', #55594, 24.99999999999985434 ) ;
#23065=ORIENTED_EDGE ( 'NONE', *, *, #39970, .F. ) ;
#23067=ORIENTED_EDGE ( 'NONE', *, *, #28907, .T. ) ;
#23094=ORIENTED_EDGE ( 'NONE', *, *, #17731, .F. ) ;
#23096=VERTEX_POINT ( 'NONE', #67252 ) ;
#23097=DIRECTION ( 'NONE',  ( -0.000000000000000000, -0.000000000000000000, 1.000000000000000000 ) ) ;
#23099=DIRECTION ( 'NONE',  ( -0.2225209339563184452, 0.9749279121818226201, 0.000000000000000000 ) ) ;
#23100=CARTESIAN_POINT ( 'NONE',  ( -51.84164840787130402, -39.21024726209533640, 40.00000000000003553 ) ) ;
#23106=ORIENTED_EDGE ( 'NONE', *, *, #68060, .T. ) ;
#23115=EDGE_LOOP ( 'NONE', ( #33693, #33735, #17520, #25529 ) ) ;
#23116=AXIS2_PLACEMENT_3D ( 'NONE', #45137, #13824, #8904 ) ;
#23123=ORIENTED_EDGE ( 'NONE', *, *, #17460, .F. ) ;
#23126=CARTESIAN_POINT ( 'NONE',  ( -71.90777365577140756, 21.14201501538314076, 41.38025477438755928 ) ) ;
#23141=ORIENTED_EDGE ( 'NONE', *, *, #38439, .T. ) ;
#23142=CYLINDRICAL_SURFACE ( 'NONE', #23896, 65.36598343705435354 ) ;
#23143=ORIENTED_EDGE ( 'NONE', *, *, #67750, .T. ) ;
#23147=CARTESIAN_POINT ( 'NONE',  ( 10.78925482157233340, 22.68765681156020264, 3.061616997868437868E-16 ) ) ;
#23148=ORIENTED_EDGE ( 'NONE', *, *, #18337, .T. ) ;
#23153=VERTEX_POINT ( 'NONE', #69292 ) ;
#23163=ORIENTED_EDGE ( 'NONE', *, *, #29612, .T. ) ;
#23165=CARTESIAN_POINT ( 'NONE',  ( -4.613603609465520172, 74.86839895266042788, 170.0000000000000000 ) ) ;
#23170=ADVANCED_FACE ( 'NONE', ( #62985 ), #22970, .T. ) ;
#23179=ORIENTED_EDGE ( 'NONE', *, *, #64852, .T. ) ;
#23180=EDGE_CURVE ( 'NONE', #13968, #25239, #52432, .T. ) ;
#23185=FACE_OUTER_BOUND ( 'NONE', #1546, .T. ) ;
#23186=CARTESIAN_POINT ( 'NONE',  ( 20.79325243092002751, 13.87950479462545772, 0.000000000000000000 ) ) ;
#23187=CARTESIAN_POINT ( 'NONE',  ( 61.91366885787729046, 28.42865614898999738, 3.061616997868437868E-16 ) ) ;
#23206=ORIENTED_EDGE ( 'NONE', *, *, #17460, .T. ) ;
#23208=ORIENTED_EDGE ( 'NONE', *, *, #3187, .T. ) ;
#23212=CARTESIAN_POINT ( 'NONE',  ( -30.63688115438417725, -13.36654903315597309, 6.893343212288941757 ) ) ;
#23220=CARTESIAN_POINT ( 'NONE',  ( 60.82895951008426749, -30.68107831874540636, 3.061616997868437868E-16 ) ) ;
#23221=ORIENTED_EDGE ( 'NONE', *, *, #54121, .F. ) ;
#23225=DIRECTION ( 'NONE',  ( 0.9362348706397417564, -0.3513748240813305279, 0.000000000000000000 ) ) ;
#23227=DIRECTION ( 'NONE',  ( -0.000000000000000000, -0.000000000000000000, -1.000000000000000000 ) ) ;
#23232=DIRECTION ( 'NONE',  ( -0.000000000000000000, -0.000000000000000000, -1.000000000000000000 ) ) ;
#23236=VERTEX_POINT ( 'NONE', #64710 ) ;
#23237=CIRCLE ( 'NONE', #25497, 25.12245591505646303 ) ;
#23240=VERTEX_POINT ( 'NONE', #29425 ) ;
#23244=ORIENTED_EDGE ( 'NONE', *, *, #7255, .F. ) ;
#23255=ORIENTED_EDGE ( 'NONE', *, *, #36557, .T. ) ;
#23263=CARTESIAN_POINT ( 'NONE',  ( 74.62299871641495486, 5.461138973199016533, 3.061616997868437868E-16 ) ) ;
#23267=ORIENTED_EDGE ( 'NONE', *, *, #65101, .F. ) ;
#23269=EDGE_CURVE ( 'NONE', #22457, #58687, #50875, .T. ) ;
#23272=LINE ( 'NONE', #48920, #45301 ) ;
#23273=CARTESIAN_POINT ( 'NONE',  ( -21.27554331372999741, 61.43430442924864820, 43.58025477438756923 ) ) ;
#23278=VECTOR ( 'NONE', #30401, 1000.000000000000114 ) ;
#23279=DIRECTION ( 'NONE',  ( -0.6910626489868580968, -0.7227948638273978821, 0.000000000000000000 ) ) ;
#23285=ADVANCED_FACE ( 'NONE', ( #48850 ), #32698, .F. ) ;
#23288=DIRECTION ( 'NONE',  ( -0.7818314824680221431, -0.6234898018587431423, 0.000000000000000000 ) ) ;
#23292=ADVANCED_FACE ( 'NONE', ( #54129 ), #27411, .T. ) ;
#23296=DIRECTION ( 'NONE',  ( -0.000000000000000000, -0.000000000000000000, -1.000000000000000000 ) ) ;
#23300=PLANE ( 'NONE',  #36475 ) ;
#23304=CARTESIAN_POINT ( 'NONE',  ( 0.000000000000000000, 0.000000000000000000, 40.00000000000003553 ) ) ;
#23310=AXIS2_PLACEMENT_3D ( 'NONE', #348, #33072, #4 ) ;
#23311=ORIENTED_EDGE ( 'NONE', *, *, #53666, .T. ) ;
#23314=DIRECTION ( 'NONE',  ( 0.000000000000000000, 0.000000000000000000, 1.000000000000000000 ) ) ;
#23318=ORIENTED_EDGE ( 'NONE', *, *, #28923, .F. ) ;
#23323=VECTOR ( 'NONE', #58060, 1000.000000000000114 ) ;
#23325=CARTESIAN_POINT ( 'NONE',  ( -64.18058723658640474, -10.37664328995270857, 41.38025477438755928 ) ) ;
#23336=CARTESIAN_POINT ( 'NONE',  ( -46.06722295615723795, -46.37372919877118704, 43.58025477438756212 ) ) ;
#23338=CARTESIAN_POINT ( 'NONE',  ( 0.000000000000000000, 0.000000000000000000, 0.000000000000000000 ) ) ;
#23343=ORIENTED_EDGE ( 'NONE', *, *, #380, .F. ) ;
#23351=CARTESIAN_POINT ( 'NONE',  ( 34.43940527065382895, 66.63700071734666608, 170.0000000000000000 ) ) ;
#23356=CARTESIAN_POINT ( 'NONE',  ( -49.45633214486770868, -14.94581086528446789, 26.66469066592268788 ) ) ;
#23357=VERTEX_POINT ( 'NONE', #4419 ) ;
#23362=CARTESIAN_POINT ( 'NONE',  ( 0.000000000000000000, 0.000000000000000000, 41.38025477438755928 ) ) ;
#23366=FACE_OUTER_BOUND ( 'NONE', #41420, .T. ) ;
#23373=CARTESIAN_POINT ( 'NONE',  ( -4.180838820196604466, 65.23214221112780820, 3.125053320693570611E-16 ) ) ;
#23375=B_SPLINE_CURVE_WITH_KNOTS ( 'NONE', 3,
 ( #18324, #39781, #29232, #29568, #23952, #61241 ),
 .UNSPECIFIED., .F., .F.,
 ( 4, 2, 4 ),
 ( 1.095770181104900047E-06, 0.03239442681617710207, 0.06478775786217309818 ),
 .UNSPECIFIED. ) ;
#23393=AXIS2_PLACEMENT_3D ( 'NONE', #12712, #6731, #50349 ) ;
#23395=ORIENTED_EDGE ( 'NONE', *, *, #60222, .T. ) ;
#23398=DIRECTION ( 'NONE',  ( 1.000000000000000000, 0.000000000000000000, 0.000000000000000000 ) ) ;
#23400=LINE ( 'NONE', #29350, #32205 ) ;
#23404=ORIENTED_EDGE ( 'NONE', *, *, #64103, .F. ) ;
#23405=VERTEX_POINT ( 'NONE', #10041 ) ;
#23412=LINE ( 'NONE', #29035, #32251 ) ;
#23424=ORIENTED_EDGE ( 'NONE', *, *, #22083, .T. ) ;
#23431=CARTESIAN_POINT ( 'NONE',  ( 0.000000000000000000, 0.000000000000000000, 41.38025477438755928 ) ) ;
#23433=ADVANCED_FACE ( 'NONE', ( #35750 ), #17331, .T. ) ;
#23435=DIRECTION ( 'NONE',  ( 0.3090169943749582759, -0.9510565162951499785, 0.000000000000000000 ) ) ;
#23438=CARTESIAN_POINT ( 'NONE',  ( 26.12852347772543737, 70.00000000000000000, 129.5802547743875550 ) ) ;
#23439=EDGE_LOOP ( 'NONE', ( #37397, #58569, #23424, #57408 ) ) ;
#23440=ORIENTED_EDGE ( 'NONE', *, *, #54651, .T. ) ;
#23441=ADVANCED_FACE ( 'NONE', ( #59252 ), #32528, .T. ) ;
#23450=CARTESIAN_POINT ( 'NONE',  ( -4.164416015344990285, -64.86646004871191451, 170.0000000000000000 ) ) ;
#23454=FACE_OUTER_BOUND ( 'NONE', #18935, .T. ) ;
#23464=CARTESIAN_POINT ( 'NONE',  ( 4.165045035620156710, 64.88046627338040651, 3.061616997868437868E-16 ) ) ;
#23468=CARTESIAN_POINT ( 'NONE',  ( -71.90777365577110913, -21.14201501538416395, 41.38025477438755928 ) ) ;
#23472=CIRCLE ( 'NONE', #61666, 24.99999999999985434 ) ;
#23475=LINE ( 'NONE', #44203, #56511 ) ;
#23493=ADVANCED_FACE ( 'NONE', ( #31838 ), #26334, .T. ) ;
#23495=VERTEX_POINT ( 'NONE', #4756 ) ;
#23500=ORIENTED_EDGE ( 'NONE', *, *, #44691, .T. ) ;
#23510=CARTESIAN_POINT ( 'NONE',  ( -22.06416059020191867, 12.01293505575286602, 0.000000000000000000 ) ) ;
#23514=VERTEX_POINT ( 'NONE', #16692 ) ;
#23516=ADVANCED_FACE ( 'NONE', ( #69463 ), #64892, .T. ) ;
#23538=DIRECTION ( 'NONE',  ( 0.9839295885986322210, -0.1785568947986229393, 0.000000000000000000 ) ) ;
#23544=ORIENTED_EDGE ( 'NONE', *, *, #17779, .F. ) ;
#23545=CARTESIAN_POINT ( 'NONE',  ( 8.828807734114020533, 74.48902371486721563, 170.0000000000000000 ) ) ;
#23554=AXIS2_PLACEMENT_3D ( 'NONE', #40127, #56293, #52734 ) ;
#23563=CARTESIAN_POINT ( 'NONE',  ( -53.31111153860250340, -37.18770477615797176, 170.0000000000000000 ) ) ;
#23567=DIRECTION ( 'NONE',  ( 0.9009688679024155933, 0.4338837391175656699, 0.000000000000000000 ) ) ;
#23571=ORIENTED_EDGE ( 'NONE', *, *, #57132, .F. ) ;
#23578=CARTESIAN_POINT ( 'NONE',  ( 12.93264331410934354, -21.39501663729232916, 0.000000000000000000 ) ) ;
#23581=AXIS2_PLACEMENT_3D ( 'NONE', #26949, #48376, #56039 ) ;
#23594=ADVANCED_FACE ( 'NONE', ( #66466 ), #34794, .F. ) ;
#23606=CARTESIAN_POINT ( 'NONE',  ( 0.000000000000000000, 0.000000000000000000, 40.00000000000003553 ) ) ;
#23611=EDGE_LOOP ( 'NONE', ( #66245, #24910, #42669, #40612 ) ) ;
#23621=EDGE_CURVE ( 'NONE', #42894, #35286, #24245, .T. ) ;
#23626=ORIENTED_EDGE ( 'NONE', *, *, #41161, .T. ) ;
#23627=ORIENTED_EDGE ( 'NONE', *, *, #8274, .F. ) ;
#23635=ORIENTED_EDGE ( 'NONE', *, *, #43186, .T. ) ;
#23639=CARTESIAN_POINT ( 'NONE',  ( -61.29635759142615115, 21.66977272663494958, 170.0000000000000000 ) ) ;
#23643=CARTESIAN_POINT ( 'NONE',  ( -65.36598343705435354, 0.000000000000000000, 41.38025477438755928 ) ) ;
#23645=LINE ( 'NONE', #56689, #66735 ) ;
#23650=ORIENTED_EDGE ( 'NONE', *, *, #25744, .T. ) ;
#23654=CARTESIAN_POINT ( 'NONE',  ( -32.53122303423116790, 7.681316636107238693, 6.893342932236740772 ) ) ;
#23674=CARTESIAN_POINT ( 'NONE',  ( -4.613603609464498767, -74.86839895266049894, 170.0000000000000000 ) ) ;
#23677=VECTOR ( 'NONE', #65571, 1000.000000000000114 ) ;
#23680=VECTOR ( 'NONE', #7731, 1000.000000000000000 ) ;
#23688=CARTESIAN_POINT ( 'NONE',  ( -65.00200000000002376, 1.250000000000011546, 41.38025477438755928 ) ) ;
#23697=VECTOR ( 'NONE', #12816, 1000.000000000000000 ) ;
#23701=CARTESIAN_POINT ( 'NONE',  ( 0.000000000000000000, 0.000000000000000000, 40.00000000000003553 ) ) ;
#23704=ORIENTED_EDGE ( 'NONE', *, *, #42413, .T. ) ;
#23708=CARTESIAN_POINT ( 'NONE',  ( -27.33809850692101051, 60.78020202768021818, 34.48241823986843713 ) ) ;
#23714=CARTESIAN_POINT ( 'NONE',  ( -64.83840629396345889, -4.580509716060184644, 40.00000000000003553 ) ) ;
#23723=CARTESIAN_POINT ( 'NONE',  ( 0.000000000000000000, 0.000000000000000000, 170.0000000000000000 ) ) ;
#23725=ORIENTED_EDGE ( 'NONE', *, *, #58455, .T. ) ;
#23737=ORIENTED_EDGE ( 'NONE', *, *, #9343, .T. ) ;
#23740=ADVANCED_FACE ( 'NONE', ( #56583 ), #17914, .T. ) ;
#23744=ORIENTED_EDGE ( 'NONE', *, *, #18650, .F. ) ;
#23745=DIRECTION ( 'NONE',  ( -1.000000000000000000, 0.000000000000000000, 0.000000000000000000 ) ) ;
#23753=ORIENTED_EDGE ( 'NONE', *, *, #1270, .T. ) ;
#23762=VERTEX_POINT ( 'NONE', #57283 ) ;
#23767=DIRECTION ( 'NONE',  ( -0.000000000000000000, -0.000000000000000000, -1.000000000000000000 ) ) ;
#23775=AXIS2_PLACEMENT_3D ( 'NONE', #20174, #25122, #8936 ) ;
#23780=CIRCLE ( 'NONE', #1325, 65.00000000000000000 ) ;
#23789=ORIENTED_EDGE ( 'NONE', *, *, #27091, .T. ) ;
#23796=CARTESIAN_POINT ( 'NONE',  ( 24.96873044429758082, -1.250000000000021982, 0.000000000000000000 ) ) ;
#23805=DIRECTION ( 'NONE',  ( -1.000000000000000000, 1.509903313490212895E-14, 2.135044278125301096E-16 ) ) ;
#23812=ORIENTED_EDGE ( 'NONE', *, *, #7801, .T. ) ;
#23833=VECTOR ( 'NONE', #51341, 1000.000000000000000 ) ;
#23835=CIRCLE ( 'NONE', #58654, 25.12245591505646303 ) ;
#23837=EDGE_LOOP ( 'NONE', ( #32925, #38279, #21548, #5281 ) ) ;
#23839=ORIENTED_EDGE ( 'NONE', *, *, #6902, .T. ) ;
#23840=CIRCLE ( 'NONE', #52977, 65.36598343705435354 ) ;
#23843=EDGE_CURVE ( 'NONE', #29654, #67731, #41854, .T. ) ;
#23859=ORIENTED_EDGE ( 'NONE', *, *, #55021, .T. ) ;
#23861=ORIENTED_EDGE ( 'NONE', *, *, #37219, .T. ) ;
#23862=CARTESIAN_POINT ( 'NONE',  ( 0.000000000000000000, 0.000000000000000000, 41.38025477438755928 ) ) ;
#23865=DIRECTION ( 'NONE',  ( 0.08963930890344089242, -0.9959742939952384022, 2.500042656554810340E-16 ) ) ;
#23872=CARTESIAN_POINT ( 'NONE',  ( 0.000000000000000000, 0.000000000000000000, 0.000000000000000000 ) ) ;
#23873=CARTESIAN_POINT ( 'NONE',  ( 28.03312937960905060, 18.20512990257157426, 6.893342934923163412 ) ) ;
#23880=VERTEX_POINT ( 'NONE', #21703 ) ;
#23881=VECTOR ( 'NONE', #52301, 1000.000000000000000 ) ;
#23885=DIRECTION ( 'NONE',  ( 1.000000000000000000, 0.000000000000000000, 0.000000000000000000 ) ) ;
#23892=VECTOR ( 'NONE', #9072, 1000.000000000000000 ) ;
#23896=AXIS2_PLACEMENT_3D ( 'NONE', #5557, #17859, #59020 ) ;
#23898=ORIENTED_EDGE ( 'NONE', *, *, #59527, .T. ) ;
#23901=DIRECTION ( 'NONE',  ( 0.9749279121818227312, 0.2225209339563184729, 5.102127870520021228E-18 ) ) ;
#23903=FACE_OUTER_BOUND ( 'NONE', #58031, .T. ) ;
#23908=CYLINDRICAL_SURFACE ( 'NONE', #53022, 65.36598343705435354 ) ;
#23920=AXIS2_PLACEMENT_3D ( 'NONE', #37508, #58613, #59645 ) ;
#23923=LINE ( 'NONE', #18992, #65075 ) ;
#23929=AXIS2_PLACEMENT_3D ( 'NONE', #26308, #64272, #37891 ) ;
#23937=VERTEX_POINT ( 'NONE', #23468 ) ;
#23951=ORIENTED_EDGE ( 'NONE', *, *, #46140, .F. ) ;
#23952=CARTESIAN_POINT ( 'NONE',  ( -17.35806719188560265, 28.56537455181723928, 6.893343212288936428 ) ) ;
#23953=VERTEX_POINT ( 'NONE', #44907 ) ;
#23957=FACE_OUTER_BOUND ( 'NONE', #36609, .T. ) ;
#23984=AXIS2_PLACEMENT_3D ( 'NONE', #65868, #27857, #49300 ) ;
#23986=VECTOR ( 'NONE', #66920, 1000.000000000000227 ) ;
#23987=ORIENTED_EDGE ( 'NONE', *, *, #48862, .F. ) ;
#23990=AXIS2_PLACEMENT_3D ( 'NONE', #66614, #40215, #8205 ) ;
#23991=DIRECTION ( 'NONE',  ( -0.000000000000000000, -0.000000000000000000, -1.000000000000000000 ) ) ;
#23993=EDGE_CURVE ( 'NONE', #11589, #46342, #30460, .T. ) ;
#24014=ORIENTED_EDGE ( 'NONE', *, *, #38207, .T. ) ;
#24023=VERTEX_POINT ( 'NONE', #21619 ) ;
#24026=ORIENTED_EDGE ( 'NONE', *, *, #12395, .F. ) ;
#24036=PLANE ( 'NONE',  #56828 ) ;
#24039=ORIENTED_EDGE ( 'NONE', *, *, #53887, .F. ) ;
#24040=AXIS2_PLACEMENT_3D ( 'NONE', #3489, #62931, #45714 ) ;
#24043=VERTEX_POINT ( 'NONE', #48673 ) ;
#24044=DIRECTION ( 'NONE',  ( -0.000000000000000000, -0.000000000000000000, 1.000000000000000000 ) ) ;
#24050=EDGE_CURVE ( 'NONE', #16525, #8487, #43065, .T. ) ;
#24056=ADVANCED_FACE ( 'NONE', ( #64536 ), #4754, .F. ) ;
#24064=DIRECTION ( 'NONE',  ( -3.989004196750080799E-18, -3.181124695048499213E-18, -1.000000000000000000 ) ) ;
#24073=ADVANCED_FACE ( 'NONE', ( #64185 ), #16690, .T. ) ;
#24084=LINE ( 'NONE', #61360, #63781 ) ;
#24085=CARTESIAN_POINT ( 'NONE',  ( 64.98797965777978902, 1.249999999999979350, 170.0000000000000000 ) ) ;
#24089=CARTESIAN_POINT ( 'NONE',  ( 8.828807734114011652, 74.48902371486721563, 133.5802547743875550 ) ) ;
#24091=ORIENTED_EDGE ( 'NONE', *, *, #35809, .T. ) ;
#24108=VERTEX_POINT ( 'NONE', #11400 ) ;
#24115=DIRECTION ( 'NONE',  ( 0.000000000000000000, 0.000000000000000000, 1.000000000000000000 ) ) ;
#24119=FACE_OUTER_BOUND ( 'NONE', #1720, .T. ) ;
#24126=ORIENTED_EDGE ( 'NONE', *, *, #28085, .T. ) ;
#24142=EDGE_CURVE ( 'NONE', #35701, #57672, #33236, .T. ) ;
#24154=DIRECTION ( 'NONE',  ( 0.9510565162951544194, -0.3090169943749446757, 0.000000000000000000 ) ) ;
#24163=EDGE_CURVE ( 'NONE', #34668, #45811, #39836, .T. ) ;
#24187=DIRECTION ( 'NONE',  ( -0.2225209339563042066, -0.9749279121818259508, 0.000000000000000000 ) ) ;
#24194=VERTEX_POINT ( 'NONE', #60653 ) ;
#24195=PLANE ( 'NONE',  #55860 ) ;
#24210=ORIENTED_EDGE ( 'NONE', *, *, #2326, .T. ) ;
#24221=EDGE_LOOP ( 'NONE', ( #45018, #4686, #65598, #21780 ) ) ;
#24231=VECTOR ( 'NONE', #43732, 1000.000000000000114 ) ;
#24233=CARTESIAN_POINT ( 'NONE',  ( 11.30618213853385967, 74.15344055032308290, 170.0000000000000000 ) ) ;
#24245=LINE ( 'NONE', #67166, #460 ) ;
#24263=ORIENTED_EDGE ( 'NONE', *, *, #22647, .T. ) ;
#24271=CARTESIAN_POINT ( 'NONE',  ( 73.51344971438123821, 14.61114034329559352, 41.38025477438755928 ) ) ;
#24299=ORIENTED_EDGE ( 'NONE', *, *, #133, .T. ) ;
#24319=LINE ( 'NONE', #55973, #32361 ) ;
#24323=CARTESIAN_POINT ( 'NONE',  ( 7.533997733929801655, -64.93035244659006366, 6.377659838150150565E-18 ) ) ;
#24328=CARTESIAN_POINT ( 'NONE',  ( 0.000000000000000000, 0.000000000000000000, 170.0000000000000000 ) ) ;
#24330=CONICAL_SURFACE ( 'NONE', #45706, 74.95140232871122521, 0.8777644062502172329 ) ;
#24333=EDGE_CURVE ( 'NONE', #5466, #56882, #3239, .T. ) ;
#24335=CARTESIAN_POINT ( 'NONE',  ( -84.49322488516129681, 0.000000000000000000, 43.58025477438756212 ) ) ;
#24337=CARTESIAN_POINT ( 'NONE',  ( -2.374459999240197572, -25.00999262126968148, 0.000000000000000000 ) ) ;
#24339=CARTESIAN_POINT ( 'NONE',  ( -63.33140416796853600, 16.18162651919395500, 41.38025477438755928 ) ) ;
#24340=CARTESIAN_POINT ( 'NONE',  ( 0.000000000000000000, 0.000000000000000000, 0.000000000000000000 ) ) ;
#24349=DIRECTION ( 'NONE',  ( 0.000000000000000000, 0.000000000000000000, 1.000000000000000000 ) ) ;
#24351=CARTESIAN_POINT ( 'NONE',  ( 22.93737758745371735, 9.943676855699235873, 0.000000000000000000 ) ) ;
#24355=ORIENTED_EDGE ( 'NONE', *, *, #43049, .F. ) ;
#24357=ORIENTED_EDGE ( 'NONE', *, *, #8082, .F. ) ;
#24359=CARTESIAN_POINT ( 'NONE',  ( -18.24318075359455804, -17.27206262134411574, 0.000000000000000000 ) ) ;
#24361=VERTEX_POINT ( 'NONE', #52847 ) ;
#24369=AXIS2_PLACEMENT_3D ( 'NONE', #13233, #68003, #35981 ) ;
#24370=LINE ( 'NONE', #45814, #47745 ) ;
#24388=DIRECTION ( 'NONE',  ( 0.3090169943749447312, 0.9510565162951544194, -0.000000000000000000 ) ) ;
#24392=AXIS2_PLACEMENT_3D ( 'NONE', #6619, #65371, #6263 ) ;
#24394=VERTEX_POINT ( 'NONE', #11324 ) ;
#24397=DIRECTION ( 'NONE',  ( -0.000000000000000000, -0.000000000000000000, -1.000000000000000000 ) ) ;
#24400=EDGE_CURVE ( 'NONE', #26725, #67396, #25299, .T. ) ;
#24403=LINE ( 'NONE', #19810, #12476 ) ;
#24407=ORIENTED_EDGE ( 'NONE', *, *, #61876, .T. ) ;
#24408=CARTESIAN_POINT ( 'NONE',  ( 8.942470798084380945, -23.47701018505899739, 3.061616997868437868E-16 ) ) ;
#24411=CARTESIAN_POINT ( 'NONE',  ( -13.32397999418070533, 63.99361958670518646, 41.38025477438755928 ) ) ;
#24416=VERTEX_POINT ( 'NONE', #20854 ) ;
#24420=AXIS2_PLACEMENT_3D ( 'NONE', #22857, #18628, #7030 ) ;
#24422=CARTESIAN_POINT ( 'NONE',  ( 9.962235950565768050, -64.23203137738408941, 40.00000000000003553 ) ) ;
#24426=AXIS2_PLACEMENT_3D ( 'NONE', #28898, #60195, #2508 ) ;
#24427=B_SPLINE_CURVE_WITH_KNOTS ( 'NONE', 3,
 ( #36671, #10609, #9592, #5347 ),
 .UNSPECIFIED., .F., .F.,
 ( 4, 4 ),
 ( 0.1259919275528360305, 0.1829744153748752156 ),
 .UNSPECIFIED. ) ;
#24435=DIRECTION ( 'NONE',  ( -0.000000000000000000, -0.000000000000000000, -1.000000000000000000 ) ) ;
#24442=ORIENTED_EDGE ( 'NONE', *, *, #52416, .F. ) ;
#24443=EDGE_LOOP ( 'NONE', ( #30489, #33331, #68676, #36266, #18924, #26155, #42329, #40409, #63348 ) ) ;
#24444=FACE_OUTER_BOUND ( 'NONE', #16527, .T. ) ;
#24446=DIRECTION ( 'NONE',  ( 0.5128992774058949156, 0.8584487936018728726, 2.500042656554809354E-16 ) ) ;
#24447=VERTEX_POINT ( 'NONE', #59508 ) ;
#24457=CARTESIAN_POINT ( 'NONE',  ( -3.566018963826330879, 51.54211443464424036, 26.66469066592269144 ) ) ;
#24469=CARTESIAN_POINT ( 'NONE',  ( -63.33140416796830152, -16.18162651919485384, 6.377659838150159810E-18 ) ) ;
#24470=ADVANCED_FACE ( 'NONE', ( #17303 ), #23300, .T. ) ;
#24481=EDGE_CURVE ( 'NONE', #37440, #26997, #55284, .T. ) ;
#24493=VERTEX_POINT ( 'NONE', #59857 ) ;
#24495=AXIS2_PLACEMENT_3D ( 'NONE', #22377, #59999, #6894 ) ;
#24497=CARTESIAN_POINT ( 'NONE',  ( 70.34686579112809568, 18.11777090454216577, 170.0000000000000000 ) ) ;
#24501=CARTESIAN_POINT ( 'NONE',  ( -74.81012118577224612, 5.477980300262961677, 170.0000000000000000 ) ) ;
#24505=DIRECTION ( 'NONE',  ( 0.9009688679024218105, -0.4338837391175525693, 0.000000000000000000 ) ) ;
#24507=CARTESIAN_POINT ( 'NONE',  ( 20.89850557012432830, 13.94239061780435662, 3.061616997868437868E-16 ) ) ;
#24516=ORIENTED_EDGE ( 'NONE', *, *, #18886, .T. ) ;
#24521=CARTESIAN_POINT ( 'NONE',  ( 0.000000000000000000, 0.000000000000000000, 40.00000000000003553 ) ) ;
#24538=CARTESIAN_POINT ( 'NONE',  ( -34.75846525699014933, 54.92585086258208804, 40.00000000000003553 ) ) ;
#24540=VERTEX_POINT ( 'NONE', #18351 ) ;
#24546=EDGE_CURVE ( 'NONE', #38709, #43082, #15183, .T. ) ;
#24552=VERTEX_POINT ( 'NONE', #4171 ) ;
#24565=EDGE_CURVE ( 'NONE', #62736, #34240, #68018, .T. ) ;
#24568=CARTESIAN_POINT ( 'NONE',  ( -65.20298343242130557, -4.613322252418190494, 43.58025477438756212 ) ) ;
#24577=LINE ( 'NONE', #13656, #31846 ) ;
#24600=ORIENTED_EDGE ( 'NONE', *, *, #29303, .F. ) ;
#24602=CARTESIAN_POINT ( 'NONE',  ( 21.27121078971612889, 61.42097029141972087, 73.58025477438755502 ) ) ;
#24609=( NAMED_UNIT ( * ) PLANE_ANGLE_UNIT ( ) SI_UNIT ( $, .RADIAN. ) );
#24620=ORIENTED_EDGE ( 'NONE', *, *, #19312, .F. ) ;
#24622=EDGE_CURVE ( 'NONE', #45386, #7953, #48422, .T. ) ;
#24626=LINE ( 'NONE', #7499, #44348 ) ;
#24627=ORIENTED_EDGE ( 'NONE', *, *, #8021, .F. ) ;
#24634=EDGE_CURVE ( 'NONE', #33798, #40228, #65331, .T. ) ;
#24635=CARTESIAN_POINT ( 'NONE',  ( 36.85262215550067566, 53.56030941157737146, 170.0000000000000000 ) ) ;
#24645=ADVANCED_FACE ( 'NONE', ( #611 ), #64987, .T. ) ;
#24650=CARTESIAN_POINT ( 'NONE',  ( -4.613603609465529054, 74.86839895266042788, 133.5802547743875550 ) ) ;
#24654=FACE_OUTER_BOUND ( 'NONE', #36832, .T. ) ;
#24666=CARTESIAN_POINT ( 'NONE',  ( 60.82895951008426749, -30.68107831874539926, 43.58025477438756923 ) ) ;
#24680=CARTESIAN_POINT ( 'NONE',  ( -2.747334540031024730, -33.31268936679798287, 6.893343212288937316 ) ) ;
#24691=CARTESIAN_POINT ( 'NONE',  ( 0.000000000000000000, 0.000000000000000000, 170.0000000000000000 ) ) ;
#24693=AXIS2_PLACEMENT_3D ( 'NONE', #54882, #7054, #28512 ) ;
#24696=ORIENTED_EDGE ( 'NONE', *, *, #65600, .T. ) ;
#24707=ORIENTED_EDGE ( 'NONE', *, *, #28336, .T. ) ;
#24711=CIRCLE ( 'NONE', #30324, 65.36598343705435354 ) ;
#24712=FACE_OUTER_BOUND ( 'NONE', #52819, .T. ) ;
#24724=ORIENTED_EDGE ( 'NONE', *, *, #43009, .F. ) ;
#24725=CARTESIAN_POINT ( 'NONE',  ( -14.19745717986860534, 56.58567516677720022, 27.58472369372398347 ) ) ;
#24727=CYLINDRICAL_SURFACE ( 'NONE', #5342, 65.36598343705435354 ) ;
#24728=DIRECTION ( 'NONE',  ( -1.000000000000000000, 0.000000000000000000, 0.000000000000000000 ) ) ;
#24739=ORIENTED_EDGE ( 'NONE', *, *, #48620, .T. ) ;
#24752=PLANE ( 'NONE',  #30802 ) ;
#24760=EDGE_CURVE ( 'NONE', #28906, #26796, #35654, .T. ) ;
#24764=CARTESIAN_POINT ( 'NONE',  ( 0.000000000000000000, 0.000000000000000000, 0.000000000000000000 ) ) ;
#24772=LINE ( 'NONE', #35322, #67219 ) ;
#24775=ORIENTED_EDGE ( 'NONE', *, *, #8831, .T. ) ;
#24776=CARTESIAN_POINT ( 'NONE',  ( -25.10237775011639982, -1.004202417053851937, 0.000000000000000000 ) ) ;
#24784=ORIENTED_EDGE ( 'NONE', *, *, #10397, .T. ) ;
#24789=VECTOR ( 'NONE', #2753, 1000.000000000000000 ) ;
#24794=ORIENTED_EDGE ( 'NONE', *, *, #42643, .T. ) ;
#24800=CARTESIAN_POINT ( 'NONE',  ( -15.67984581961064450, 63.08044415722863363, 170.0000000000000000 ) ) ;
#24802=LINE ( 'NONE', #30081, #36415 ) ;
#24808=CARTESIAN_POINT ( 'NONE',  ( 6.590627084543000613, -57.96611065023441967, 27.58472315868180402 ) ) ;
#24824=VERTEX_POINT ( 'NONE', #63864 ) ;
#24826=EDGE_LOOP ( 'NONE', ( #3163, #39248, #50039, #2913, #41058, #616, #11308, #6727, #93 ) ) ;
#24832=AXIS2_PLACEMENT_3D ( 'NONE', #11737, #5762, #49711 ) ;
#24836=CIRCLE ( 'NONE', #13630, 74.95140232871122521 ) ;
#24854=DIRECTION ( 'NONE',  ( 0.2225209339563184452, -0.9749279121818226201, 0.000000000000000000 ) ) ;
#24861=EDGE_CURVE ( 'NONE', #69425, #54206, #57553, .T. ) ;
#24865=ORIENTED_EDGE ( 'NONE', *, *, #39661, .F. ) ;
#24868=CARTESIAN_POINT ( 'NONE',  ( -52.69240448066660321, 53.30312580971368419, 41.38025477438755928 ) ) ;
#24869=ADVANCED_FACE ( 'NONE', ( #51921 ), #36440, .F. ) ;
#24893=VECTOR ( 'NONE', #63237, 1000.000000000000000 ) ;
#24895=DIRECTION ( 'NONE',  ( -1.000000000000000000, 0.000000000000000000, 0.000000000000000000 ) ) ;
#24898=EDGE_LOOP ( 'NONE', ( #55350, #21264, #9061, #21243 ) ) ;
#24910=ORIENTED_EDGE ( 'NONE', *, *, #18743, .F. ) ;
#24916=DIRECTION ( 'NONE',  ( -0.2660368455666826670, 0.9639628606958512425, 5.102127870520021228E-18 ) ) ;
#24918=CARTESIAN_POINT ( 'NONE',  ( 15.68296563925591514, -63.09411298019745828, 170.0000000000000000 ) ) ;
#24922=DIRECTION ( 'NONE',  ( 5.096990367256702165E-18, 2.289061013375335776E-19, -1.000000000000000000 ) ) ;
#24924=LINE ( 'NONE', #51655, #8420 ) ;
#24937=PLANE ( 'NONE',  #32962 ) ;
#24940=EDGE_LOOP ( 'NONE', ( #24299, #11934, #39262, #60059 ) ) ;
#24941=CYLINDRICAL_SURFACE ( 'NONE', #49233, 65.00000000000000000 ) ;
#24947=ADVANCED_FACE ( 'NONE', ( #528 ), #21976, .T. ) ;
#24949=AXIS2_PLACEMENT_3D ( 'NONE', #49616, #17264, #39096 ) ;
#24950=DIRECTION ( 'NONE',  ( -0.000000000000000000, -0.000000000000000000, -1.000000000000000000 ) ) ;
#24952=EDGE_CURVE ( 'NONE', #27671, #50073, #9562, .T. ) ;
#24959=DIRECTION ( 'NONE',  ( 0.000000000000000000, 0.000000000000000000, -1.000000000000000000 ) ) ;
#24961=DIRECTION ( 'NONE',  ( 1.000000000000000000, 0.000000000000000000, 0.000000000000000000 ) ) ;
#24964=CARTESIAN_POINT ( 'NONE',  ( 12.93264331410902379, 21.39501663729252456, 0.000000000000000000 ) ) ;
#24972=EDGE_CURVE ( 'NONE', #14304, #29783, #34291, .T. ) ;
#24977=DIRECTION ( 'NONE',  ( -0.04486483035051863633, 0.9989930665413144784, 0.000000000000000000 ) ) ;
#24982=B_SPLINE_CURVE_WITH_KNOTS ( 'NONE', 3,
 ( #59028, #58338, #63636, #63289 ),
 .UNSPECIFIED., .F., .F.,
 ( 4, 4 ),
 ( 9.900409499076797036E-07, 0.05658314289920114010 ),
 .UNSPECIFIED. ) ;
#25008=AXIS2_PLACEMENT_3D ( 'NONE', #52962, #4787, #47683 ) ;
#25011=CARTESIAN_POINT ( 'NONE',  ( 6.564829507346109594, 24.24955267099648992, 3.061616997868437868E-16 ) ) ;
#25012=CARTESIAN_POINT ( 'NONE',  ( 8.828807734114020533, 74.48902371486721563, 170.0000000000000000 ) ) ;
#25015=DIRECTION ( 'NONE',  ( -0.000000000000000000, -0.000000000000000000, -1.000000000000000000 ) ) ;
#25030=EDGE_CURVE ( 'NONE', #67530, #62756, #56764, .T. ) ;
#25031=ORIENTED_EDGE ( 'NONE', *, *, #49375, .T. ) ;
#25035=CARTESIAN_POINT ( 'NONE',  ( 29.69502258243350923, 57.82046033912877903, 170.0000000000000000 ) ) ;
#25037=DIRECTION ( 'NONE',  ( -0.6910626489868580968, -0.7227948638273978821, 0.000000000000000000 ) ) ;
#25043=DIRECTION ( 'NONE',  ( -1.000000000000000000, 0.000000000000000000, 0.000000000000000000 ) ) ;
#25046=VECTOR ( 'NONE', #32275, 1000.000000000000000 ) ;
#25050=CYLINDRICAL_SURFACE ( 'NONE', #5073, 65.36598343705435354 ) ;
#25061=CARTESIAN_POINT ( 'NONE',  ( -63.73419499958981049, -12.83646726144931449, 170.0000000000000000 ) ) ;
#25063=DIRECTION ( 'NONE',  ( -0.000000000000000000, -0.000000000000000000, -1.000000000000000000 ) ) ;
#25080=ORIENTED_EDGE ( 'NONE', *, *, #32573, .F. ) ;
#25089=FACE_OUTER_BOUND ( 'NONE', #24826, .T. ) ;
#25097=VERTEX_POINT ( 'NONE', #55737 ) ;
#25099=VECTOR ( 'NONE', #65152, 1000.000000000000114 ) ;
#25100=CARTESIAN_POINT ( 'NONE',  ( -4.180838820195677208, -65.23214221112785083, 6.377659838150132077E-18 ) ) ;
#25108=CARTESIAN_POINT ( 'NONE',  ( 11.30618213853385967, 74.15344055032308290, 43.58025477438756212 ) ) ;
#25109=B_SPLINE_CURVE_WITH_KNOTS ( 'NONE', 3,
 ( #54744, #44898, #17459, #27666, #18518, #34005 ),
 .UNSPECIFIED., .F., .F.,
 ( 4, 2, 4 ),
 ( 0.03218941534092201184, 0.06469837595388618079, 0.09720733656685034973 ),
 .UNSPECIFIED. ) ;
#25119=FACE_OUTER_BOUND ( 'NONE', #4121, .T. ) ;
#25122=DIRECTION ( 'NONE',  ( -0.000000000000000000, -0.000000000000000000, -1.000000000000000000 ) ) ;
#25134=DIRECTION ( 'NONE',  ( -0.000000000000000000, -0.000000000000000000, -1.000000000000000000 ) ) ;
#25138=CARTESIAN_POINT ( 'NONE',  ( 61.62594073580573450, -21.79346734964915555, 43.58025477438756212 ) ) ;
#25139=CARTESIAN_POINT ( 'NONE',  ( 21.98745393275190807, 71.71550996510528364, 73.58025477438755502 ) ) ;
#25143=LINE ( 'NONE', #67023, #4529 ) ;
#25148=VERTEX_POINT ( 'NONE', #56780 ) ;
#25163=DIRECTION ( 'NONE',  ( -0.000000000000000000, -0.000000000000000000, 1.000000000000000000 ) ) ;
#25170=EDGE_LOOP ( 'NONE', ( #52181, #7594, #42259, #33081 ) ) ;
#25177=CARTESIAN_POINT ( 'NONE',  ( -1.666933348992582609, 64.97862212458815634, 133.5802547743875550 ) ) ;
#25179=ORIENTED_EDGE ( 'NONE', *, *, #41634, .F. ) ;
#25180=ORIENTED_EDGE ( 'NONE', *, *, #53016, .T. ) ;
#25181=EDGE_CURVE ( 'NONE', #51034, #14895, #56566, .T. ) ;
#25187=CARTESIAN_POINT ( 'NONE',  ( 24.96873044429758082, -1.250000000000021982, 0.000000000000000000 ) ) ;
#25191=FACE_OUTER_BOUND ( 'NONE', #48784, .T. ) ;
#25199=DIRECTION ( 'NONE',  ( -0.000000000000000000, -0.000000000000000000, -1.000000000000000000 ) ) ;
#25217=DIRECTION ( 'NONE',  ( -1.000000000000000000, 0.000000000000000000, 0.000000000000000000 ) ) ;
#25220=ORIENTED_EDGE ( 'NONE', *, *, #22390, .F. ) ;
#25224=DIRECTION ( 'NONE',  ( -0.000000000000000000, -0.000000000000000000, -1.000000000000000000 ) ) ;
#25226=DIRECTION ( 'NONE',  ( 0.2225209339563042066, 0.9749279121818259508, 0.000000000000000000 ) ) ;
#25227=VERTEX_POINT ( 'NONE', #46908 ) ;
#25229=ORIENTED_EDGE ( 'NONE', *, *, #5071, .F. ) ;
#25239=VERTEX_POINT ( 'NONE', #67688 ) ;
#25242=VECTOR ( 'NONE', #26591, 1000.000000000000114 ) ;
#25251=DIRECTION ( 'NONE',  ( -0.6234898018587431423, 0.7818314824680220321, 0.000000000000000000 ) ) ;
#25258=CYLINDRICAL_SURFACE ( 'NONE', #59802, 65.00000000000000000 ) ;
#25261=LINE ( 'NONE', #67147, #37722 ) ;
#25273=EDGE_CURVE ( 'NONE', #66442, #66077, #65802, .T. ) ;
#25277=VERTEX_POINT ( 'NONE', #26835 ) ;
#25287=EDGE_CURVE ( 'NONE', #46531, #42019, #21216, .T. ) ;
#25288=ORIENTED_EDGE ( 'NONE', *, *, #67750, .F. ) ;
#25297=VECTOR ( 'NONE', #36315, 1000.000000000000000 ) ;
#25299=CIRCLE ( 'NONE', #64583, 25.12245591505646303 ) ;
#25304=CONICAL_SURFACE ( 'NONE', #34338, 65.00000000000000000, 0.7853981633974497223 ) ;
#25309=DIRECTION ( 'NONE',  ( 0.3090169943749447312, 0.9510565162951545304, 0.000000000000000000 ) ) ;
#25315=ORIENTED_EDGE ( 'NONE', *, *, #33239, .F. ) ;
#25317=CARTESIAN_POINT ( 'NONE',  ( -24.39249304643438521, 60.24953346690454481, 133.5802547743875550 ) ) ;
#25321=CARTESIAN_POINT ( 'NONE',  ( 0.000000000000000000, 0.000000000000000000, 0.000000000000000000 ) ) ;
#25322=DIRECTION ( 'NONE',  ( 0.1342332658176522420, 0.9909497617679351444, 0.000000000000000000 ) ) ;
#25325=DIRECTION ( 'NONE',  ( 1.000000000000000000, 0.000000000000000000, -0.000000000000000000 ) ) ;
#25327=EDGE_CURVE ( 'NONE', #4383, #48419, #5712, .T. ) ;
#25330=CARTESIAN_POINT ( 'NONE',  ( -74.81012118577218928, -5.477980300263996405, 43.58025477438756212 ) ) ;
#25348=AXIS2_PLACEMENT_3D ( 'NONE', #40012, #49860, #1689 ) ;
#25353=VECTOR ( 'NONE', #17614, 1000.000000000000227 ) ;
#25354=ORIENTED_EDGE ( 'NONE', *, *, #25760, .F. ) ;
#25357=PLANE ( 'NONE',  #12981 ) ;
#25359=DIRECTION ( 'NONE',  ( -1.000000000000000000, 0.000000000000000000, 0.000000000000000000 ) ) ;
#25368=CARTESIAN_POINT ( 'NONE',  ( -62.31345272479909880, 18.49415068377641447, 40.00000000000003553 ) ) ;
#25375=EDGE_CURVE ( 'NONE', #6967, #62563, #11334, .T. ) ;
#25377=VERTEX_POINT ( 'NONE', #6055 ) ;
#25384=AXIS2_PLACEMENT_3D ( 'NONE', #63645, #59634, #32918 ) ;
#25389=CIRCLE ( 'NONE', #1834, 25.12245591505646303 ) ;
#25395=ORIENTED_EDGE ( 'NONE', *, *, #24622, .T. ) ;
#25397=AXIS2_PLACEMENT_3D ( 'NONE', #59467, #11278, #33100 ) ;
#25417=ORIENTED_EDGE ( 'NONE', *, *, #37702, .F. ) ;
#25418=CARTESIAN_POINT ( 'NONE',  ( 35.43132475791147584, -14.63273365840185924, 13.32819397642333037 ) ) ;
#25429=CARTESIAN_POINT ( 'NONE',  ( 63.72039997003725631, -12.83396383267754537, 170.0000000000000000 ) ) ;
#25430=VERTEX_POINT ( 'NONE', #54943 ) ;
#25435=EDGE_CURVE ( 'NONE', #6675, #35022, #18019, .T. ) ;
#25442=CARTESIAN_POINT ( 'NONE',  ( 45.82394788922869822, -46.11928342727429708, 170.0000000000000000 ) ) ;
#25451=ORIENTED_EDGE ( 'NONE', *, *, #40407, .F. ) ;
#25465=DIRECTION ( 'NONE',  ( 0.000000000000000000, 0.000000000000000000, 1.000000000000000000 ) ) ;
#25469=CARTESIAN_POINT ( 'NONE',  ( 51.85299110299440173, 39.21848821248450179, 170.0000000000000000 ) ) ;
#25478=VERTEX_POINT ( 'NONE', #39469 ) ;
#25485=VECTOR ( 'NONE', #35910, 1000.000000000000000 ) ;
#25487=CARTESIAN_POINT ( 'NONE',  ( 23.17627457812085723, 71.32923872213659422, 0.000000000000000000 ) ) ;
#25490=AXIS2_PLACEMENT_3D ( 'NONE', #62551, #46704, #67830 ) ;
#25494=DIRECTION ( 'NONE',  ( 0.000000000000000000, 0.000000000000000000, -1.000000000000000000 ) ) ;
#25497=AXIS2_PLACEMENT_3D ( 'NONE', #12987, #22832, #33037 ) ;
#25506=VERTEX_POINT ( 'NONE', #50715 ) ;
#25511=CARTESIAN_POINT ( 'NONE',  ( 0.000000000000000000, 0.000000000000000000, 170.0000000000000000 ) ) ;
#25512=PLANE ( 'NONE',  #26435 ) ;
#25529=ORIENTED_EDGE ( 'NONE', *, *, #8181, .F. ) ;
#25531=VECTOR ( 'NONE', #68513, 1000.000000000000000 ) ;
#25536=DIRECTION ( 'NONE',  ( -1.000000000000000000, 0.000000000000000000, 0.000000000000000000 ) ) ;
#25552=ORIENTED_EDGE ( 'NONE', *, *, #17726, .T. ) ;
#25553=DIRECTION ( 'NONE',  ( -0.000000000000000000, -0.000000000000000000, -1.000000000000000000 ) ) ;
#25572=CARTESIAN_POINT ( 'NONE',  ( 0.000000000000000000, 0.000000000000000000, 0.000000000000000000 ) ) ;
#25574=CARTESIAN_POINT ( 'NONE',  ( -24.40147488398712383, 5.437648709335531905, 0.000000000000000000 ) ) ;
#25581=CARTESIAN_POINT ( 'NONE',  ( 69.77839676787863255, 27.52340539440045575, 43.58025477438756923 ) ) ;
#25598=EDGE_CURVE ( 'NONE', #49220, #69425, #42191, .T. ) ;
#25615=DIRECTION ( 'NONE',  ( 0.6910626489868685329, -0.7227948638273878901, 0.000000000000000000 ) ) ;
#25618=DIRECTION ( 'NONE',  ( -0.2225209339563184452, 0.9749279121818226201, 0.000000000000000000 ) ) ;
#25621=LINE ( 'NONE', #36505, #25531 ) ;
#25625=LINE ( 'NONE', #52339, #45458 ) ;
#25626=ORIENTED_EDGE ( 'NONE', *, *, #3558, .F. ) ;
#25630=FACE_OUTER_BOUND ( 'NONE', #43956, .T. ) ;
#25639=DIRECTION ( 'NONE',  ( -0.000000000000000000, -0.000000000000000000, 1.000000000000000000 ) ) ;
#25641=VECTOR ( 'NONE', #51873, 1000.000000000000000 ) ;
#25645=EDGE_CURVE ( 'NONE', #23880, #14487, #35930, .T. ) ;
#25648=DIRECTION ( 'NONE',  ( -1.000000000000000000, 0.000000000000000000, 0.000000000000000000 ) ) ;
#25654=CARTESIAN_POINT ( 'NONE',  ( 23.17627457812085723, 71.32923872213659422, 0.000000000000000000 ) ) ;
#25656=DIRECTION ( 'NONE',  ( -0.000000000000000000, -0.000000000000000000, -1.000000000000000000 ) ) ;
#25674=PLANE ( 'NONE',  #9652 ) ;
#25681=VERTEX_POINT ( 'NONE', #9543 ) ;
#25682=VECTOR ( 'NONE', #63615, 1000.000000000000000 ) ;
#25685=EDGE_CURVE ( 'NONE', #54974, #43521, #69131, .T. ) ;
#25700=DIRECTION ( 'NONE',  ( 1.000000000000000000, 0.000000000000000000, 0.000000000000000000 ) ) ;
#25701=FACE_OUTER_BOUND ( 'NONE', #67013, .T. ) ;
#25717=ORIENTED_EDGE ( 'NONE', *, *, #61795, .F. ) ;
#25722=DIRECTION ( 'NONE',  ( -1.000000000000000000, 0.000000000000000000, 0.000000000000000000 ) ) ;
#25723=EDGE_CURVE ( 'NONE', #9408, #24552, #36625, .T. ) ;
#25730=CARTESIAN_POINT ( 'NONE',  ( 22.18075376363910323, 11.79626863379964696, 0.000000000000000000 ) ) ;
#25735=LINE ( 'NONE', #46828, #28064 ) ;
#25744=EDGE_CURVE ( 'NONE', #41626, #49164, #5296, .T. ) ;
#25750=ORIENTED_EDGE ( 'NONE', *, *, #60981, .F. ) ;
#25752=CARTESIAN_POINT ( 'NONE',  ( 0.000000000000000000, 0.000000000000000000, 41.38025477438755928 ) ) ;
#25753=LINE ( 'NONE', #3593, #35916 ) ;
#25754=B_SPLINE_CURVE_WITH_KNOTS ( 'NONE', 3,
 ( #41609, #57789, #42302, #63764 ),
 .UNSPECIFIED., .F., .F.,
 ( 4, 4 ),
 ( 9.900409498950027967E-07, 0.05658314289920114010 ),
 .UNSPECIFIED. ) ;
#25758=DIRECTION ( 'NONE',  ( -0.04486483035051862939, 0.9989930665413143673, 0.000000000000000000 ) ) ;
#25760=EDGE_CURVE ( 'NONE', #26008, #61883, #47495, .T. ) ;
#25761=ADVANCED_FACE ( 'NONE', ( #15513 ), #68956, .T. ) ;
#25763=DIRECTION ( 'NONE',  ( 9.110201094256374036E-19, -5.020134576618366632E-18, -1.000000000000000000 ) ) ;
#25766=DIRECTION ( 'NONE',  ( 0.2225209339563184452, -0.9749279121818226201, 0.000000000000000000 ) ) ;
#25767=LINE ( 'NONE', #47196, #53456 ) ;
#25770=DIRECTION ( 'NONE',  ( 1.000000000000000000, 0.000000000000000000, 0.000000000000000000 ) ) ;
#25772=CARTESIAN_POINT ( 'NONE',  ( 11.30618213853490239, -74.15344055032291237, 170.0000000000000000 ) ) ;
#25789=DIRECTION ( 'NONE',  ( 0.2225209339563184452, -0.9749279121818226201, 0.000000000000000000 ) ) ;
#25792=ORIENTED_EDGE ( 'NONE', *, *, #46678, .T. ) ;
#25800=LINE ( 'NONE', #15232, #43881 ) ;
#25804=CARTESIAN_POINT ( 'NONE',  ( -42.32797523529043104, -61.85511477251480983, 41.38025477438755928 ) ) ;
#25806=EDGE_CURVE ( 'NONE', #42469, #55620, #16542, .T. ) ;
#25811=DIRECTION ( 'NONE',  ( 0.000000000000000000, 0.000000000000000000, 1.000000000000000000 ) ) ;
#25814=ORIENTED_EDGE ( 'NONE', *, *, #55858, .F. ) ;
#25826=CIRCLE ( 'NONE', #10091, 74.95140232871122521 ) ;
#25845=VECTOR ( 'NONE', #26789, 1000.000000000000114 ) ;
#25849=DIRECTION ( 'NONE',  ( 0.000000000000000000, 0.000000000000000000, 1.000000000000000000 ) ) ;
#25851=ADVANCED_FACE ( 'NONE', ( #1766 ), #7391, .T. ) ;
#25858=ORIENTED_EDGE ( 'NONE', *, *, #29015, .T. ) ;
#25864=LINE ( 'NONE', #63833, #9064 ) ;
#25875=CIRCLE ( 'NONE', #2284, 25.12245591505646303 ) ;
#25896=ORIENTED_EDGE ( 'NONE', *, *, #17060, .F. ) ;
#25900=ORIENTED_EDGE ( 'NONE', *, *, #45020, .T. ) ;
#25901=EDGE_CURVE ( 'NONE', #37545, #22341, #30926, .T. ) ;
#25903=VERTEX_POINT ( 'NONE', #9465 ) ;
#25908=VECTOR ( 'NONE', #11840, 1000.000000000000114 ) ;
#25917=LINE ( 'NONE', #18644, #51583 ) ;
#25922=CARTESIAN_POINT ( 'NONE',  ( -52.13778968636736977, -39.42540649522066332, 3.125053320693577513E-16 ) ) ;
#25923=ORIENTED_EDGE ( 'NONE', *, *, #50193, .T. ) ;
#25927=CARTESIAN_POINT ( 'NONE',  ( -24.75616454008739709, -3.483147608717210630, 0.000000000000000000 ) ) ;
#25931=ORIENTED_EDGE ( 'NONE', *, *, #60345, .F. ) ;
#25958=VERTEX_POINT ( 'NONE', #9813 ) ;
#25964=CARTESIAN_POINT ( 'NONE',  ( 0.000000000000000000, 0.000000000000000000, 170.0000000000000000 ) ) ;
#25978=CARTESIAN_POINT ( 'NONE',  ( 39.77028211725739482, 51.87520073220942862, 41.38025477438755928 ) ) ;
#25982=B_SPLINE_CURVE_WITH_KNOTS ( 'NONE', 3,
 ( #14573, #14235, #14907, #2639, #36375, #36029 ),
 .UNSPECIFIED., .F., .F.,
 ( 4, 2, 4 ),
 ( 1.095770181106998147E-06, 0.03239442681617711595, 0.06478775786217312593 ),
 .UNSPECIFIED. ) ;
#25996=CARTESIAN_POINT ( 'NONE',  ( 41.72486082342750535, 50.31647622756258187, 6.377659838150125143E-18 ) ) ;
#25998=ORIENTED_EDGE ( 'NONE', *, *, #56446, .F. ) ;
#25999=LINE ( 'NONE', #21391, #26624 ) ;
#26003=ORIENTED_EDGE ( 'NONE', *, *, #49305, .F. ) ;
#26008=VERTEX_POINT ( 'NONE', #4694 ) ;
#26009=LINE ( 'NONE', #42847, #40098 ) ;
#26017=ORIENTED_EDGE ( 'NONE', *, *, #28408, .T. ) ;
#26020=CARTESIAN_POINT ( 'NONE',  ( -45.14452651541945727, 49.02628140145412772, 34.48241795236665297 ) ) ;
#26036=VECTOR ( 'NONE', #40164, 1000.000000000000000 ) ;
#26040=DIRECTION ( 'NONE',  ( -0.000000000000000000, -0.000000000000000000, -1.000000000000000000 ) ) ;
#26042=ORIENTED_EDGE ( 'NONE', *, *, #15554, .F. ) ;
#26046=CARTESIAN_POINT ( 'NONE',  ( 21.98745393275189386, 71.71550996510525522, 43.58025477438756923 ) ) ;
#26050=PLANE ( 'NONE',  #30567 ) ;
#26052=EDGE_CURVE ( 'NONE', #33038, #66237, #47588, .T. ) ;
#26053=VECTOR ( 'NONE', #47424, 1000.000000000000000 ) ;
#26056=ORIENTED_EDGE ( 'NONE', *, *, #37626, .T. ) ;
#26061=EDGE_CURVE ( 'NONE', #62951, #57182, #11904, .T. ) ;
#26062=ORIENTED_EDGE ( 'NONE', *, *, #56326, .T. ) ;
#26073=VERTEX_POINT ( 'NONE', #47251 ) ;
#26082=AXIS2_PLACEMENT_3D ( 'NONE', #54517, #7044, #54163 ) ;
#26085=CARTESIAN_POINT ( 'NONE',  ( -56.44201257846630426, 32.26641783793562723, 41.38025477438755928 ) ) ;
#26089=CARTESIAN_POINT ( 'NONE',  ( -7.306921498789654024, -37.63116382989763764, 13.32819299319722894 ) ) ;
#26102=CARTESIAN_POINT ( 'NONE',  ( -65.36598343705435354, 0.000000000000000000, 41.38025477438755928 ) ) ;
#26104=EDGE_CURVE ( 'NONE', #46943, #19302, #14565, .T. ) ;
#26105=ORIENTED_EDGE ( 'NONE', *, *, #1246, .F. ) ;
#26113=DIRECTION ( 'NONE',  ( -4.258099457802062126E-18, 2.810746842852082347E-18, -1.000000000000000000 ) ) ;
#26116=CARTESIAN_POINT ( 'NONE',  ( -1.666933348992582609, 64.97862212458815634, 170.0000000000000000 ) ) ;
#26117=DIRECTION ( 'NONE',  ( 0.3930250316539278255, -0.9195277725514487965, 0.000000000000000000 ) ) ;
#26124=FACE_OUTER_BOUND ( 'NONE', #23115, .T. ) ;
#26128=EDGE_CURVE ( 'NONE', #43797, #26875, #19490, .T. ) ;
#26133=CIRCLE ( 'NONE', #65448, 74.95140232871122521 ) ;
#26137=LINE ( 'NONE', #47571, #2599 ) ;
#26140=B_SPLINE_CURVE_WITH_KNOTS ( 'NONE', 3,
 ( #38913, #11815, #1614, #65644, #57080, #8892 ),
 .UNSPECIFIED., .F., .F.,
 ( 4, 2, 4 ),
 ( 0.03218945466321617571, 0.06469840457090975105, 0.09720735447860334721 ),
 .UNSPECIFIED. ) ;
#26149=EDGE_CURVE ( 'NONE', #30965, #61262, #22603, .T. ) ;
#26155=ORIENTED_EDGE ( 'NONE', *, *, #16888, .T. ) ;
#26161=CARTESIAN_POINT ( 'NONE',  ( 24.34427655538957680, -5.688250960945929080, 0.000000000000000000 ) ) ;
#26165=DIRECTION ( 'NONE',  ( -0.000000000000000000, 0.000000000000000000, -1.000000000000000000 ) ) ;
#26167=CARTESIAN_POINT ( 'NONE',  ( 0.000000000000000000, 0.000000000000000000, 41.38025477438755928 ) ) ;
#26168=AXIS2_PLACEMENT_3D ( 'NONE', #35653, #57105, #55184 ) ;
#26171=FACE_OUTER_BOUND ( 'NONE', #21818, .T. ) ;
#26181=ADVANCED_FACE ( 'NONE', ( #54244 ), #44503, .T. ) ;
#26198=CARTESIAN_POINT ( 'NONE',  ( -29.70166638324966968, 57.83280658984257627, 170.0000000000000000 ) ) ;
#26202=EDGE_CURVE ( 'NONE', #2304, #30365, #452, .T. ) ;
#26203=ORIENTED_EDGE ( 'NONE', *, *, #44624, .T. ) ;
#26205=EDGE_CURVE ( 'NONE', #46223, #15646, #47936, .T. ) ;
#26211=ORIENTED_EDGE ( 'NONE', *, *, #34000, .T. ) ;
#26214=( NAMED_UNIT ( * ) PLANE_ANGLE_UNIT ( ) SI_UNIT ( $, .RADIAN. ) );
#26227=CARTESIAN_POINT ( 'NONE',  ( 0.000000000000000000, 0.000000000000000000, 40.00000000000003553 ) ) ;
#26229=EDGE_CURVE ( 'NONE', #24394, #9160, #27179, .T. ) ;
#26231=EDGE_CURVE ( 'NONE', #47253, #20436, #21226, .T. ) ;
#26245=ORIENTED_EDGE ( 'NONE', *, *, #51938, .T. ) ;
#26249=VECTOR ( 'NONE', #54300, 1000.000000000000000 ) ;
#26254=DIRECTION ( 'NONE',  ( 0.3090169943749447312, 0.9510565162951544194, -0.000000000000000000 ) ) ;
#26258=CARTESIAN_POINT ( 'NONE',  ( -59.09450113343241640, 27.07101652673493319, 170.0000000000000000 ) ) ;
#26267=EDGE_CURVE ( 'NONE', #937, #19006, #37989, .T. ) ;
#26269=CARTESIAN_POINT ( 'NONE',  ( 56.74421265833558436, 32.44697398030905333, 6.377659838150106654E-18 ) ) ;
#26272=VERTEX_POINT ( 'NONE', #1152 ) ;
#26274=CIRCLE ( 'NONE', #27413, 65.36598343705435354 ) ;
#26278=VECTOR ( 'NONE', #59499, 1000.000000000000000 ) ;
#26280=DIRECTION ( 'NONE',  ( -0.9749279121818259508, 0.2225209339563041788, 0.000000000000000000 ) ) ;
#26300=CARTESIAN_POINT ( 'NONE',  ( 0.000000000000000000, 0.000000000000000000, 2.000000000000001776 ) ) ;
#26302=CARTESIAN_POINT ( 'NONE',  ( 0.000000000000000000, 0.000000000000000000, 40.00000000000003553 ) ) ;
#26307=ORIENTED_EDGE ( 'NONE', *, *, #52408, .F. ) ;
#26308=CARTESIAN_POINT ( 'NONE',  ( 0.000000000000000000, 0.000000000000000000, 43.58025477438756212 ) ) ;
#26311=CARTESIAN_POINT ( 'NONE',  ( -2.116120943112233643, 74.98056102853672655, 133.5802547743875550 ) ) ;
#26313=LINE ( 'NONE', #47743, #36723 ) ;
#26320=DIRECTION ( 'NONE',  ( -0.000000000000000000, -0.000000000000000000, -1.000000000000000000 ) ) ;
#26321=VERTEX_POINT ( 'NONE', #26501 ) ;
#26327=AXIS2_PLACEMENT_3D ( 'NONE', #3005, #24115, #45553 ) ;
#26334=CONICAL_SURFACE ( 'NONE', #57761, 65.00000000000000000, 0.7853981633974497223 ) ;
#26335=VERTEX_POINT ( 'NONE', #59878 ) ;
#26338=CIRCLE ( 'NONE', #56613, 65.00000000000000000 ) ;
#26350=CARTESIAN_POINT ( 'NONE',  ( -84.49322488516129681, 0.000000000000000000, 43.58025477438756212 ) ) ;
#26360=ORIENTED_EDGE ( 'NONE', *, *, #58904, .F. ) ;
#26361=ORIENTED_EDGE ( 'NONE', *, *, #21212, .F. ) ;
#26364=CARTESIAN_POINT ( 'NONE',  ( -39.40355428794429571, 43.02169521020481824, 27.58472315868180402 ) ) ;
#26370=ORIENTED_EDGE ( 'NONE', *, *, #1043, .F. ) ;
#26371=VECTOR ( 'NONE', #10768, 999.9999999999998863 ) ;
#26372=CARTESIAN_POINT ( 'NONE',  ( 0.000000000000000000, 0.000000000000000000, 43.58025477438756212 ) ) ;
#26373=VERTEX_POINT ( 'NONE', #24359 ) ;
#26388=CIRCLE ( 'NONE', #7261, 65.00000000000000000 ) ;
#26394=CARTESIAN_POINT ( 'NONE',  ( -29.49715813532712971, -42.41725772201189670, 26.66469104408689361 ) ) ;
#26407=ORIENTED_EDGE ( 'NONE', *, *, #26758, .T. ) ;
#26410=CARTESIAN_POINT ( 'NONE',  ( -4.613603609465545041, 74.86839895266042788, 73.58025477438755502 ) ) ;
#26412=DIRECTION ( 'NONE',  ( -0.7227948638273978821, 0.6910626489868580968, 0.000000000000000000 ) ) ;
#26421=VECTOR ( 'NONE', #7137, 999.9999999999998863 ) ;
#26426=EDGE_CURVE ( 'NONE', #32477, #68560, #44735, .T. ) ;
#26429=AXIS2_PLACEMENT_3D ( 'NONE', #63942, #42141, #63605 ) ;
#26430=ORIENTED_EDGE ( 'NONE', *, *, #54938, .F. ) ;
#26435=AXIS2_PLACEMENT_3D ( 'NONE', #52223, #20215, #57166 ) ;
#26447=LINE ( 'NONE', #47884, #15324 ) ;
#26461=DIRECTION ( 'NONE',  ( -0.000000000000000000, -0.000000000000000000, -1.000000000000000000 ) ) ;
#26467=CARTESIAN_POINT ( 'NONE',  ( -25.03927907554148291, -61.76276460681540925, 34.48241823986843713 ) ) ;
#26474=AXIS2_PLACEMENT_3D ( 'NONE', #54106, #21771, #27392 ) ;
#26478=VECTOR ( 'NONE', #19395, 1000.000000000000000 ) ;
#26488=FACE_OUTER_BOUND ( 'NONE', #30619, .T. ) ;
#26489=CYLINDRICAL_SURFACE ( 'NONE', #23775, 65.36598343705435354 ) ;
#26491=CARTESIAN_POINT ( 'NONE',  ( -60.41792053122248518, -24.01035990323518021, 170.0000000000000000 ) ) ;
#26498=ORIENTED_EDGE ( 'NONE', *, *, #19047, .T. ) ;
#26501=CARTESIAN_POINT ( 'NONE',  ( 70.60157554497457966, 25.16207943727196295, 41.38025477438755928 ) ) ;
#26522=ADVANCED_FACE ( 'NONE', ( #40868 ), #25050, .T. ) ;
#26523=VECTOR ( 'NONE', #62744, 1000.000000000000000 ) ;
#26524=VECTOR ( 'NONE', #42241, 1000.000000000000000 ) ;
#26525=ORIENTED_EDGE ( 'NONE', *, *, #9687, .T. ) ;
#26532=PLANE ( 'NONE',  #64647 ) ;
#26537=ORIENTED_EDGE ( 'NONE', *, *, #58850, .T. ) ;
#26551=ORIENTED_EDGE ( 'NONE', *, *, #3730, .T. ) ;
#26556=ORIENTED_EDGE ( 'NONE', *, *, #21450, .T. ) ;
#26560=CARTESIAN_POINT ( 'NONE',  ( 0.000000000000000000, 0.000000000000000000, 0.000000000000000000 ) ) ;
#26561=CARTESIAN_POINT ( 'NONE',  ( 0.000000000000000000, 0.000000000000000000, 0.000000000000000000 ) ) ;
#26563=DIRECTION ( 'NONE',  ( 1.000000000000000000, 0.000000000000000000, 0.000000000000000000 ) ) ;
#26567=ORIENTED_EDGE ( 'NONE', *, *, #4964, .T. ) ;
#26569=CYLINDRICAL_SURFACE ( 'NONE', #18151, 65.36598343705435354 ) ;
#26575=EDGE_CURVE ( 'NONE', #42734, #19578, #47171, .T. ) ;
#26583=CARTESIAN_POINT ( 'NONE',  ( -61.41100614348627573, -43.07262267896732766, 43.58025477438756212 ) ) ;
#26588=B_SPLINE_CURVE_WITH_KNOTS ( 'NONE', 3,
 ( #37597, #5252, #15805, #32675, #5923, #53419 ),
 .UNSPECIFIED., .F., .F.,
 ( 4, 2, 4 ),
 ( 0.03218950539619244711, 0.06469844149454670457, 0.09720737759290096203 ),
 .UNSPECIFIED. ) ;
#26589=CARTESIAN_POINT ( 'NONE',  ( 11.29825944729730303, 74.09495289493001735, 41.38025477438755928 ) ) ;
#26591=DIRECTION ( 'NONE',  ( -0.9839295885986321100, 0.1785568947986229116, 0.000000000000000000 ) ) ;
#26593=ORIENTED_EDGE ( 'NONE', *, *, #62583, .T. ) ;
#26595=ORIENTED_EDGE ( 'NONE', *, *, #35835, .F. ) ;
#26599=EDGE_CURVE ( 'NONE', #21961, #3417, #32061, .T. ) ;
#26600=DIRECTION ( 'NONE',  ( -0.000000000000000000, -0.000000000000000000, -1.000000000000000000 ) ) ;
#26602=ORIENTED_EDGE ( 'NONE', *, *, #68461, .T. ) ;
#26605=ORIENTED_EDGE ( 'NONE', *, *, #60899, .T. ) ;
#26609=AXIS2_PLACEMENT_3D ( 'NONE', #26302, #48758, #58631 ) ;
#26611=CARTESIAN_POINT ( 'NONE',  ( -2.116120943112233643, 74.98056102853672655, 170.0000000000000000 ) ) ;
#26621=CARTESIAN_POINT ( 'NONE',  ( -40.27405704175634327, 63.28161525591265502, 170.0000000000000000 ) ) ;
#26623=ADVANCED_FACE ( 'NONE', ( #63385 ), #68324, .T. ) ;
#26624=VECTOR ( 'NONE', #42511, 1000.000000000000000 ) ;
#26633=FACE_OUTER_BOUND ( 'NONE', #21522, .T. ) ;
#26634=ORIENTED_EDGE ( 'NONE', *, *, #52628, .F. ) ;
#26636=VECTOR ( 'NONE', #61732, 1000.000000000000000 ) ;
#26642=FACE_OUTER_BOUND ( 'NONE', #55023, .T. ) ;
#26663=AXIS2_PLACEMENT_3D ( 'NONE', #3564, #52770, #58399 ) ;
#26672=VECTOR ( 'NONE', #34888, 1000.000000000000114 ) ;
#26680=VERTEX_POINT ( 'NONE', #20811 ) ;
#26692=ORIENTED_EDGE ( 'NONE', *, *, #63838, .F. ) ;
#26693=DIRECTION ( 'NONE',  ( -1.000000000000000000, 0.000000000000000000, 0.000000000000000000 ) ) ;
#26702=ADVANCED_FACE ( 'NONE', ( #48211 ), #5329, .T. ) ;
#26712=ORIENTED_EDGE ( 'NONE', *, *, #47001, .F. ) ;
#26714=DIRECTION ( 'NONE',  ( -0.000000000000000000, -0.000000000000000000, -1.000000000000000000 ) ) ;
#26719=CIRCLE ( 'NONE', #30097, 65.36598343705435354 ) ;
#26725=VERTEX_POINT ( 'NONE', #69344 ) ;
#26739=ORIENTED_EDGE ( 'NONE', *, *, #56025, .T. ) ;
#26746=PLANE ( 'NONE',  #54075 ) ;
#26747=EDGE_CURVE ( 'NONE', #32676, #58236, #9228, .T. ) ;
#26750=ORIENTED_EDGE ( 'NONE', *, *, #42928, .T. ) ;
#26754=DIRECTION ( 'NONE',  ( 0.1342332658176522420, 0.9909497617679351444, 0.000000000000000000 ) ) ;
#26757=VERTEX_POINT ( 'NONE', #64065 ) ;
#26758=EDGE_CURVE ( 'NONE', #52558, #38915, #7732, .T. ) ;
#26765=CIRCLE ( 'NONE', #69438, 65.00000000000000000 ) ;
#26766=EDGE_CURVE ( 'NONE', #27252, #45135, #63733, .T. ) ;
#26774=LINE ( 'NONE', #47870, #18899 ) ;
#26776=CARTESIAN_POINT ( 'NONE',  ( -74.58602291351368763, 7.967916035251062290, 43.58025477438756212 ) ) ;
#26782=VERTEX_POINT ( 'NONE', #64761 ) ;
#26785=DIRECTION ( 'NONE',  ( -0.000000000000000000, -0.000000000000000000, -1.000000000000000000 ) ) ;
#26789=DIRECTION ( 'NONE',  ( 0.9989930665413143673, 0.04486483035051862939, -0.000000000000000000 ) ) ;
#26796=VERTEX_POINT ( 'NONE', #59120 ) ;
#26798=VERTEX_POINT ( 'NONE', #12344 ) ;
#26799=CARTESIAN_POINT ( 'NONE',  ( -62.66631205405158767, -18.59153367093452403, 3.125053320693551382E-16 ) ) ;
#26803=DIRECTION ( 'NONE',  ( -0.4738686624729966379, -0.8805955318567391110, 0.000000000000000000 ) ) ;
#26804=FACE_OUTER_BOUND ( 'NONE', #68530, .T. ) ;
#26808=CARTESIAN_POINT ( 'NONE',  ( -21.77424121867212392, -54.12382879860719243, 27.58472369383527578 ) ) ;
#26814=CIRCLE ( 'NONE', #49237, 25.12245591505646303 ) ;
#26823=CARTESIAN_POINT ( 'NONE',  ( -55.15976438495108169, -34.41253982194112382, 0.000000000000000000 ) ) ;
#26829=EDGE_CURVE ( 'NONE', #27522, #21766, #28158, .T. ) ;
#26835=CARTESIAN_POINT ( 'NONE',  ( -66.97713359923307053, -33.64188291209072190, 41.38025477438755928 ) ) ;
#26839=VERTEX_POINT ( 'NONE', #16219 ) ;
#26843=ORIENTED_EDGE ( 'NONE', *, *, #5096, .F. ) ;
#26848=ORIENTED_EDGE ( 'NONE', *, *, #50040, .T. ) ;
#26862=CARTESIAN_POINT ( 'NONE',  ( 14.07802349576188483, 39.28261617699831731, 13.79046340968177198 ) ) ;
#26874=CARTESIAN_POINT ( 'NONE',  ( 0.000000000000000000, 0.000000000000000000, 170.0000000000000000 ) ) ;
#26875=VERTEX_POINT ( 'NONE', #17975 ) ;
#26876=CARTESIAN_POINT ( 'NONE',  ( 0.000000000000000000, 0.000000000000000000, 41.38025477438755928 ) ) ;
#26883=EDGE_CURVE ( 'NONE', #44841, #14663, #38743, .T. ) ;
#26887=ORIENTED_EDGE ( 'NONE', *, *, #5392, .F. ) ;
#26893=CIRCLE ( 'NONE', #23554, 65.00000000000000000 ) ;
#26901=CARTESIAN_POINT ( 'NONE',  ( 0.000000000000000000, 0.000000000000000000, 41.38025477438755928 ) ) ;
#26908=CARTESIAN_POINT ( 'NONE',  ( 12.93264331410934354, -21.39501663729232916, 0.000000000000000000 ) ) ;
#26911=DIRECTION ( 'NONE',  ( -2.437361367520486303E-16, 5.563118268671760803E-17, 1.000000000000000000 ) ) ;
#26916=ORIENTED_EDGE ( 'NONE', *, *, #13190, .F. ) ;
#26924=ORIENTED_EDGE ( 'NONE', *, *, #7048, .T. ) ;
#26926=DIRECTION ( 'NONE',  ( -0.04486483035051862939, 0.9989930665413143673, 0.000000000000000000 ) ) ;
#26932=DIRECTION ( 'NONE',  ( 1.000000000000000000, 0.000000000000000000, -0.000000000000000000 ) ) ;
#26948=FACE_OUTER_BOUND ( 'NONE', #4909, .T. ) ;
#26949=CARTESIAN_POINT ( 'NONE',  ( 0.000000000000000000, 0.000000000000000000, 43.58025477438756212 ) ) ;
#26956=DIRECTION ( 'NONE',  ( 0.000000000000000000, 0.000000000000000000, 1.000000000000000000 ) ) ;
#26960=EDGE_CURVE ( 'NONE', #35779, #58062, #34525, .T. ) ;
#26966=FACE_OUTER_BOUND ( 'NONE', #14073, .T. ) ;
#26979=VERTEX_POINT ( 'NONE', #8814 ) ;
#26997=VERTEX_POINT ( 'NONE', #47448 ) ;
#27004=ORIENTED_EDGE ( 'NONE', *, *, #11327, .T. ) ;
#27012=ORIENTED_EDGE ( 'NONE', *, *, #31514, .F. ) ;
#27024=COLOUR_RGB ( '',0.7921568627450980005, 0.8196078431372548767, 0.9333333333333333481 ) ;
#27025=CARTESIAN_POINT ( 'NONE',  ( 0.000000000000000000, 0.000000000000000000, 40.00000000000003553 ) ) ;
#27033=CARTESIAN_POINT ( 'NONE',  ( -14.27739076362511206, -30.22315722928984627, 6.893343212288939093 ) ) ;
#27044=FACE_OUTER_BOUND ( 'NONE', #28807, .T. ) ;
#27046=DIRECTION ( 'NONE',  ( 1.000000000000000000, 0.000000000000000000, -0.000000000000000000 ) ) ;
#27055=DIRECTION ( 'NONE',  ( -1.000000000000000000, 0.000000000000000000, 0.000000000000000000 ) ) ;
#27057=VERTEX_POINT ( 'NONE', #21758 ) ;
#27063=CYLINDRICAL_SURFACE ( 'NONE', #60880, 65.00000000000000000 ) ;
#27078=CARTESIAN_POINT ( 'NONE',  ( -13.32397999418070533, 63.99361958670518646, 6.377659838150144402E-18 ) ) ;
#27079=AXIS2_PLACEMENT_3D ( 'NONE', #10622, #9607, #68680 ) ;
#27080=LINE ( 'NONE', #16184, #12161 ) ;
#27091=EDGE_CURVE ( 'NONE', #1572, #34467, #19178, .T. ) ;
#27097=EDGE_LOOP ( 'NONE', ( #27994, #16498, #33704, #24014 ) ) ;
#27098=ORIENTED_EDGE ( 'NONE', *, *, #56275, .F. ) ;
#27118=CARTESIAN_POINT ( 'NONE',  ( 25.97682105948609532, 21.03539606394572914, 6.893343212288937316 ) ) ;
#27120=FACE_OUTER_BOUND ( 'NONE', #55847, .T. ) ;
#27121=LINE ( 'NONE', #11635, #66284 ) ;
#27127=DIRECTION ( 'NONE',  ( -0.000000000000000000, 0.000000000000000000, -1.000000000000000000 ) ) ;
#27129=ORIENTED_EDGE ( 'NONE', *, *, #61637, .F. ) ;
#27132=ORIENTED_EDGE ( 'NONE', *, *, #40932, .T. ) ;
#27139=VECTOR ( 'NONE', #46790, 1000.000000000000000 ) ;
#27151=EDGE_CURVE ( 'NONE', #35812, #35756, #23063, .T. ) ;
#27158=LINE ( 'NONE', #43677, #52084 ) ;
#27162=ORIENTED_EDGE ( 'NONE', *, *, #31602, .F. ) ;
#27177=ORIENTED_EDGE ( 'NONE', *, *, #14616, .F. ) ;
#27179=LINE ( 'NONE', #49321, #32146 ) ;
#27192=DIRECTION ( 'NONE',  ( 0.9839295885986321100, -0.1785568947986229116, 0.000000000000000000 ) ) ;
#27195=FACE_OUTER_BOUND ( 'NONE', #19407, .T. ) ;
#27203=CARTESIAN_POINT ( 'NONE',  ( 0.000000000000000000, 0.000000000000000000, 0.000000000000000000 ) ) ;
#27206=ADVANCED_FACE ( 'NONE', ( #21594 ), #38782, .T. ) ;
#27224=ORIENTED_EDGE ( 'NONE', *, *, #35882, .T. ) ;
#27231=B_SPLINE_CURVE_WITH_KNOTS ( 'NONE', 3,
 ( #8271, #24457, #29720, #1962 ),
 .UNSPECIFIED., .F., .F.,
 ( 4, 4 ),
 ( 9.900409499187197193E-07, 0.05658314289920116785 ),
 .UNSPECIFIED. ) ;
#27233=CARTESIAN_POINT ( 'NONE',  ( 4.165045035621076863, -64.88046627338039229, 170.0000000000000000 ) ) ;
#27240=CARTESIAN_POINT ( 'NONE',  ( -81.83265147652316784, 46.58665115056960815, 133.5802547743875550 ) ) ;
#27242=DIRECTION ( 'NONE',  ( -0.000000000000000000, -0.000000000000000000, -1.000000000000000000 ) ) ;
#27252=VERTEX_POINT ( 'NONE', #37779 ) ;
#27253=VERTEX_POINT ( 'NONE', #21255 ) ;
#27271=VERTEX_POINT ( 'NONE', #9678 ) ;
#27277=DIRECTION ( 'NONE',  ( -0.000000000000000000, -0.000000000000000000, -1.000000000000000000 ) ) ;
#27278=VERTEX_POINT ( 'NONE', #58877 ) ;
#27280=VECTOR ( 'NONE', #12093, 999.9999999999998863 ) ;
#27293=ORIENTED_EDGE ( 'NONE', *, *, #5063, .F. ) ;
#27298=CARTESIAN_POINT ( 'NONE',  ( 24.39800339187930334, -60.26242556095670722, 43.58025477438756923 ) ) ;
#27300=LINE ( 'NONE', #48742, #7503 ) ;
#27312=EDGE_CURVE ( 'NONE', #7485, #37971, #6810, .T. ) ;
#27314=DIRECTION ( 'NONE',  ( -0.6234898018587318180, -0.7818314824680311359, 0.000000000000000000 ) ) ;
#27315=DIRECTION ( 'NONE',  ( 0.7530714660036195163, -0.6579387259397027066, 0.000000000000000000 ) ) ;
#27316=FACE_OUTER_BOUND ( 'NONE', #35034, .T. ) ;
#27320=DIRECTION ( 'NONE',  ( 0.3090169943749582759, -0.9510565162951499785, 0.000000000000000000 ) ) ;
#27322=CARTESIAN_POINT ( 'NONE',  ( 31.22608621030911280, -41.16111794767503085, 26.66469104408689006 ) ) ;
#27329=AXIS2_PLACEMENT_3D ( 'NONE', #2274, #60654, #66310 ) ;
#27344=DIRECTION ( 'NONE',  ( 0.1785568947986370669, -0.9839295885986296675, 5.102127870520021999E-18 ) ) ;
#27350=EDGE_CURVE ( 'NONE', #26757, #43605, #36256, .T. ) ;
#27358=DIRECTION ( 'NONE',  ( -0.9749279121818226201, -0.2225209339563184452, 0.000000000000000000 ) ) ;
#27361=DIRECTION ( 'NONE',  ( 0.000000000000000000, 0.000000000000000000, 1.000000000000000000 ) ) ;
#27363=EDGE_LOOP ( 'NONE', ( #50072, #53278, #12256, #35084 ) ) ;
#27367=AXIS2_PLACEMENT_3D ( 'NONE', #2194, #23991, #60921 ) ;
#27374=ORIENTED_EDGE ( 'NONE', *, *, #31321, .F. ) ;
#27375=ORIENTED_EDGE ( 'NONE', *, *, #58715, .T. ) ;
#27380=LINE ( 'NONE', #31634, #46805 ) ;
#27382=LINE ( 'NONE', #48820, #11174 ) ;
#27383=DIRECTION ( 'NONE',  ( -0.000000000000000000, -0.000000000000000000, 1.000000000000000000 ) ) ;
#27390=EDGE_CURVE ( 'NONE', #55620, #13308, #27919, .T. ) ;
#27392=DIRECTION ( 'NONE',  ( -1.000000000000000000, 0.000000000000000000, 0.000000000000000000 ) ) ;
#27403=DIRECTION ( 'NONE',  ( -1.000000000000000000, 0.000000000000000000, 0.000000000000000000 ) ) ;
#27410=AXIS2_PLACEMENT_3D ( 'NONE', #36126, #30500, #4462 ) ;
#27411=PLANE ( 'NONE',  #64531 ) ;
#27413=AXIS2_PLACEMENT_3D ( 'NONE', #62460, #4066, #4406 ) ;
#27424=AXIS2_PLACEMENT_3D ( 'NONE', #46219, #25134, #62052 ) ;
#27425=DIRECTION ( 'NONE',  ( 1.000000000000000000, 0.000000000000000000, 0.000000000000000000 ) ) ;
#27426=CARTESIAN_POINT ( 'NONE',  ( 0.000000000000000000, 0.000000000000000000, 170.0000000000000000 ) ) ;
#27427=ORIENTED_EDGE ( 'NONE', *, *, #24400, .T. ) ;
#27430=CARTESIAN_POINT ( 'NONE',  ( -72.29721455218883364, -19.95276341750119897, 43.58025477438756212 ) ) ;
#27431=CARTESIAN_POINT ( 'NONE',  ( 0.000000000000000000, 0.000000000000000000, 41.38025477438755928 ) ) ;
#27440=ADVANCED_FACE ( 'NONE', ( #46175 ), #28741, .T. ) ;
#27443=FACE_OUTER_BOUND ( 'NONE', #46456, .T. ) ;
#27448=EDGE_CURVE ( 'NONE', #19844, #4383, #65804, .T. ) ;
#27453=DIRECTION ( 'NONE',  ( -0.000000000000000000, -0.000000000000000000, -1.000000000000000000 ) ) ;
#27454=DIRECTION ( 'NONE',  ( -0.000000000000000000, -0.000000000000000000, -1.000000000000000000 ) ) ;
#27470=CYLINDRICAL_SURFACE ( 'NONE', #37269, 65.36598343705435354 ) ;
#27477=ORIENTED_EDGE ( 'NONE', *, *, #65209, .F. ) ;
#27485=EDGE_CURVE ( 'NONE', #634, #17560, #45485, .T. ) ;
#27492=ORIENTED_EDGE ( 'NONE', *, *, #34347, .F. ) ;
#27499=ORIENTED_EDGE ( 'NONE', *, *, #45433, .F. ) ;
#27517=AXIS2_PLACEMENT_3D ( 'NONE', #15632, #5065, #10681 ) ;
#27518=ORIENTED_EDGE ( 'NONE', *, *, #16439, .T. ) ;
#27522=VERTEX_POINT ( 'NONE', #51808 ) ;
#27525=VECTOR ( 'NONE', #34674, 1000.000000000000000 ) ;
#27531=ORIENTED_EDGE ( 'NONE', *, *, #47455, .T. ) ;
#27548=ORIENTED_EDGE ( 'NONE', *, *, #43186, .F. ) ;
#27555=CARTESIAN_POINT ( 'NONE',  ( -21.03405120204975276, 13.73704776265648775, 3.061616997868437868E-16 ) ) ;
#27559=VECTOR ( 'NONE', #62418, 1000.000000000000000 ) ;
#27561=ORIENTED_EDGE ( 'NONE', *, *, #50212, .F. ) ;
#27562=ORIENTED_EDGE ( 'NONE', *, *, #37558, .F. ) ;
#27568=EDGE_CURVE ( 'NONE', #57138, #33166, #24427, .T. ) ;
#27573=ORIENTED_EDGE ( 'NONE', *, *, #27568, .T. ) ;
#27574=ORIENTED_EDGE ( 'NONE', *, *, #33111, .T. ) ;
#27581=B_SPLINE_CURVE_WITH_KNOTS ( 'NONE', 3,
 ( #38711, #60155, #32734, #54874 ),
 .UNSPECIFIED., .F., .F.,
 ( 4, 4 ),
 ( 9.900409499218689877E-07, 0.05658314289920114704 ),
 .UNSPECIFIED. ) ;
#27587=( LENGTH_UNIT ( ) NAMED_UNIT ( * ) SI_UNIT ( .MILLI., .METRE. ) );
#27595=EDGE_LOOP ( 'NONE', ( #18691, #27574, #36554, #44970 ) ) ;
#27601=CARTESIAN_POINT ( 'NONE',  ( -39.55079474733624068, -51.59997227571039957, 170.0000000000000000 ) ) ;
#27613=ORIENTED_EDGE ( 'NONE', *, *, #12104, .F. ) ;
#27619=VECTOR ( 'NONE', #55019, 1000.000000000000000 ) ;
#27625=ORIENTED_EDGE ( 'NONE', *, *, #13092, .T. ) ;
#27636=VERTEX_POINT ( 'NONE', #17990 ) ;
#27638=CARTESIAN_POINT ( 'NONE',  ( -74.81012118577218928, -5.477980300263997293, 170.0000000000000000 ) ) ;
#27648=CARTESIAN_POINT ( 'NONE',  ( 21.38432669262978436, 61.76910524360982180, 41.38025477438755928 ) ) ;
#27651=CARTESIAN_POINT ( 'NONE',  ( -1.683356153843273750, 65.34430428700410687, 43.58025477438756212 ) ) ;
#27652=CARTESIAN_POINT ( 'NONE',  ( 0.000000000000000000, 0.000000000000000000, 0.000000000000000000 ) ) ;
#27659=AXIS2_PLACEMENT_3D ( 'NONE', #41926, #52481, #14843 ) ;
#27661=CARTESIAN_POINT ( 'NONE',  ( 0.000000000000000000, 0.000000000000000000, 40.00000000000003553 ) ) ;
#27665=AXIS2_PLACEMENT_3D ( 'NONE', #14789, #15826, #31658 ) ;
#27666=CARTESIAN_POINT ( 'NONE',  ( 50.71116774460843857, -28.84239744659915416, 27.58472369397436452 ) ) ;
#27671=VERTEX_POINT ( 'NONE', #43303 ) ;
#27685=EDGE_CURVE ( 'NONE', #37383, #21254, #65481, .T. ) ;
#27704=LINE ( 'NONE', #1328, #20458 ) ;
#27714=CARTESIAN_POINT ( 'NONE',  ( 57.30278335769541087, 48.40406511297401693, 170.0000000000000000 ) ) ;
#27716=VECTOR ( 'NONE', #57131, 1000.000000000000000 ) ;
#27720=FACE_OUTER_BOUND ( 'NONE', #30096, .T. ) ;
#27721=AXIS2_PLACEMENT_3D ( 'NONE', #26350, #41835, #25325 ) ;
#27729=ORIENTED_EDGE ( 'NONE', *, *, #44037, .T. ) ;
#27734=CARTESIAN_POINT ( 'NONE',  ( -6.802008071587034799, -24.18409554641273473, 0.000000000000000000 ) ) ;
#27740=ORIENTED_EDGE ( 'NONE', *, *, #28997, .T. ) ;
#27743=B_SPLINE_CURVE_WITH_KNOTS ( 'NONE', 3,
 ( #64956, #58967, #5166, #69518 ),
 .UNSPECIFIED., .F., .F.,
 ( 4, 4 ),
 ( 0.1259919275528358085, 0.1829744153748746882 ),
 .UNSPECIFIED. ) ;
#27750=EDGE_LOOP ( 'NONE', ( #45033, #62976, #44867, #5639 ) ) ;
#27753=CARTESIAN_POINT ( 'NONE',  ( 64.52696037203369883, -10.43950074664762440, 43.58025477438756212 ) ) ;
#27754=CARTESIAN_POINT ( 'NONE',  ( -62.31345272479883590, -18.49415068377726357, 40.00000000000003553 ) ) ;
#27763=DIRECTION ( 'NONE',  ( -0.000000000000000000, -0.000000000000000000, -1.000000000000000000 ) ) ;
#27766=VECTOR ( 'NONE', #3633, 1000.000000000000000 ) ;
#27773=CARTESIAN_POINT ( 'NONE',  ( 0.000000000000000000, 0.000000000000000000, 0.000000000000000000 ) ) ;
#27782=ORIENTED_EDGE ( 'NONE', *, *, #58215, .T. ) ;
#27784=EDGE_LOOP ( 'NONE', ( #2323, #3768, #27832, #17997 ) ) ;
#27787=CARTESIAN_POINT ( 'NONE',  ( -64.97888516016270444, -7.103257987406331964, 43.58025477438756212 ) ) ;
#27791=CARTESIAN_POINT ( 'NONE',  ( -16.35146342289083776, -18.91109843266265500, 0.000000000000000000 ) ) ;
#27794=EDGE_LOOP ( 'NONE', ( #2452, #57041, #27012, #4862 ) ) ;
#27797=DIRECTION ( 'NONE',  ( 1.000000000000000000, 0.000000000000000000, 0.000000000000000000 ) ) ;
#27804=ORIENTED_EDGE ( 'NONE', *, *, #9056, .F. ) ;
#27806=LINE ( 'NONE', #49245, #64888 ) ;
#27808=CIRCLE ( 'NONE', #6481, 25.12245591505646303 ) ;
#27810=DIRECTION ( 'NONE',  ( 1.156482317317871232E-16, -3.126709176169244633E-16, 1.000000000000000000 ) ) ;
#27813=LINE ( 'NONE', #17251, #6907 ) ;
#27818=ORIENTED_EDGE ( 'NONE', *, *, #20727, .T. ) ;
#27820=CONICAL_SURFACE ( 'NONE', #50284, 74.95140232871122521, 0.8777644062502172329 ) ;
#27825=DIRECTION ( 'NONE',  ( -0.000000000000000000, 1.000000000000000000, -0.000000000000000000 ) ) ;
#27832=ORIENTED_EDGE ( 'NONE', *, *, #9282, .T. ) ;
#27833=AXIS2_PLACEMENT_3D ( 'NONE', #38732, #28525, #1444 ) ;
#27841=CARTESIAN_POINT ( 'NONE',  ( -59.89379335984725117, 45.06047301136835870, 41.38025477438755928 ) ) ;
#27843=EDGE_CURVE ( 'NONE', #7110, #25478, #51389, .T. ) ;
#27851=DIRECTION ( 'NONE',  ( -0.000000000000000000, -0.000000000000000000, -1.000000000000000000 ) ) ;
#27857=DIRECTION ( 'NONE',  ( -0.000000000000000000, -0.000000000000000000, -1.000000000000000000 ) ) ;
#27863=ADVANCED_FACE ( 'NONE', ( #63321 ), #25357, .T. ) ;
#27870=DIRECTION ( 'NONE',  ( -0.000000000000000000, -0.000000000000000000, -1.000000000000000000 ) ) ;
#27872=ADVANCED_FACE ( 'NONE', ( #10524 ), #42871, .T. ) ;
#27877=PLANE ( 'NONE',  #1115 ) ;
#27879=ORIENTED_EDGE ( 'NONE', *, *, #57085, .F. ) ;
#27883=CARTESIAN_POINT ( 'NONE',  ( 47.73902449249074920, -57.85799893277823713, 170.0000000000000000 ) ) ;
#27889=EDGE_CURVE ( 'NONE', #34656, #12108, #49896, .T. ) ;
#27903=ORIENTED_EDGE ( 'NONE', *, *, #69525, .T. ) ;
#27915=PLANE ( 'NONE',  #42989 ) ;
#27918=AXIS2_PLACEMENT_3D ( 'NONE', #54773, #1318, #38604 ) ;
#27919=LINE ( 'NONE', #49007, #24231 ) ;
#27923=DIRECTION ( 'NONE',  ( -0.2225209339563184452, 0.9749279121818226201, 0.000000000000000000 ) ) ;
#27924=DIRECTION ( 'NONE',  ( -0.000000000000000000, -0.000000000000000000, -1.000000000000000000 ) ) ;
#27926=VERTEX_POINT ( 'NONE', #677 ) ;
#27942=CARTESIAN_POINT ( 'NONE',  ( 0.000000000000000000, 0.000000000000000000, 43.58025477438756212 ) ) ;
#27944=ADVANCED_FACE ( 'NONE', ( #23185 ), #16840, .F. ) ;
#27959=FACE_OUTER_BOUND ( 'NONE', #939, .T. ) ;
#27965=AXIS2_PLACEMENT_3D ( 'NONE', #43099, #52958, #53298 ) ;
#27985=DIRECTION ( 'NONE',  ( -4.573512162503992243E-19, 5.081588203714606302E-18, -1.000000000000000000 ) ) ;
#27993=ORIENTED_EDGE ( 'NONE', *, *, #60529, .F. ) ;
#27994=ORIENTED_EDGE ( 'NONE', *, *, #2977, .F. ) ;
#27997=DIRECTION ( 'NONE',  ( 1.000000000000000000, 0.000000000000000000, 0.000000000000000000 ) ) ;
#28004=PLANE ( 'NONE',  #64388 ) ;
#28007=CARTESIAN_POINT ( 'NONE',  ( -56.44201257846630426, 32.26641783793562723, 170.0000000000000000 ) ) ;
#28008=VERTEX_POINT ( 'NONE', #28092 ) ;
#28015=AXIS2_PLACEMENT_3D ( 'NONE', #51531, #62426, #14243 ) ;
#28016=DIRECTION ( 'NONE',  ( -1.954612056407539268E-16, -1.558751100573764160E-16, 1.000000000000000000 ) ) ;
#28026=LINE ( 'NONE', #13257, #17483 ) ;
#28034=CARTESIAN_POINT ( 'NONE',  ( 49.42891899764522634, -30.98851909993380360, 27.58472315868181113 ) ) ;
#28040=EDGE_LOOP ( 'NONE', ( #27625, #68471, #58209, #19289 ) ) ;
#28045=CARTESIAN_POINT ( 'NONE',  ( 0.000000000000000000, 0.000000000000000000, 40.00000000000003553 ) ) ;
#28051=DIRECTION ( 'NONE',  ( 0.8805955318567322276, 0.4738686624730095165, 2.500042656554810340E-16 ) ) ;
#28064=VECTOR ( 'NONE', #42248, 1000.000000000000114 ) ;
#28066=EDGE_LOOP ( 'NONE', ( #33861, #41036, #24091, #23812 ) ) ;
#28067=DIRECTION ( 'NONE',  ( -0.000000000000000000, -0.000000000000000000, 1.000000000000000000 ) ) ;
#28072=VERTEX_POINT ( 'NONE', #34447 ) ;
#28074=ORIENTED_EDGE ( 'NONE', *, *, #37219, .F. ) ;
#28075=AXIS2_PLACEMENT_3D ( 'NONE', #23606, #45395, #66527 ) ;
#28085=EDGE_CURVE ( 'NONE', #43922, #53047, #7353, .T. ) ;
#28088=CARTESIAN_POINT ( 'NONE',  ( -71.96466849523049802, -21.15771699337099321, 170.0000000000000000 ) ) ;
#28092=CARTESIAN_POINT ( 'NONE',  ( 17.98081503251174240, -17.36923402935755689, 0.000000000000000000 ) ) ;
#28113=ORIENTED_EDGE ( 'NONE', *, *, #28676, .F. ) ;
#28116=DIRECTION ( 'NONE',  ( -0.000000000000000000, 0.000000000000000000, -1.000000000000000000 ) ) ;
#28123=CARTESIAN_POINT ( 'NONE',  ( -71.96466849523049802, -21.15771699337099321, 170.0000000000000000 ) ) ;
#28127=ORIENTED_EDGE ( 'NONE', *, *, #51326, .T. ) ;
#28133=CIRCLE ( 'NONE', #49460, 25.12245591505646303 ) ;
#28134=ORIENTED_EDGE ( 'NONE', *, *, #38264, .T. ) ;
#28139=DIRECTION ( 'NONE',  ( -0.9959742939952382912, -0.08963930890344087854, 0.000000000000000000 ) ) ;
#28142=AXIS2_PLACEMENT_3D ( 'NONE', #14013, #28813, #29492 ) ;
#28145=ORIENTED_EDGE ( 'NONE', *, *, #24565, .F. ) ;
#28153=EDGE_LOOP ( 'NONE', ( #3501, #51537, #30698, #52279 ) ) ;
#28154=LINE ( 'NONE', #65820, #25353 ) ;
#28156=ORIENTED_EDGE ( 'NONE', *, *, #22422, .T. ) ;
#28158=LINE ( 'NONE', #38026, #43216 ) ;
#28159=DIRECTION ( 'NONE',  ( -1.000000000000000000, 0.000000000000000000, 0.000000000000000000 ) ) ;
#28160=LINE ( 'NONE', #54542, #38282 ) ;
#28162=CARTESIAN_POINT ( 'NONE',  ( 51.85299110299499148, -39.21848821248373440, 170.0000000000000000 ) ) ;
#28163=CARTESIAN_POINT ( 'NONE',  ( 17.05487707116232343, 34.33113399044100333, 13.32819299319724671 ) ) ;
#28173=VERTEX_POINT ( 'NONE', #30195 ) ;
#28174=PLANE ( 'NONE',  #3728 ) ;
#28194=EDGE_CURVE ( 'NONE', #42819, #28516, #60798, .T. ) ;
#28200=CARTESIAN_POINT ( 'NONE',  ( -68.06184294702747195, 31.38946074233368222, 41.38025477438755928 ) ) ;
#28201=CARTESIAN_POINT ( 'NONE',  ( -71.96466849523048381, -21.15771699337101808, 43.58025477438756923 ) ) ;
#28213=CARTESIAN_POINT ( 'NONE',  ( 24.79066879238614263, -3.228426989449305839, 0.000000000000000000 ) ) ;
#28214=VERTEX_POINT ( 'NONE', #2419 ) ;
#28222=ORIENTED_EDGE ( 'NONE', *, *, #31301, .T. ) ;
#28223=AXIS2_PLACEMENT_3D ( 'NONE', #54492, #47485, #64360 ) ;
#28224=ORIENTED_EDGE ( 'NONE', *, *, #21433, .F. ) ;
#28234=VECTOR ( 'NONE', #50775, 1000.000000000000000 ) ;
#28238=LINE ( 'NONE', #49333, #62873 ) ;
#28239=CYLINDRICAL_SURFACE ( 'NONE', #37415, 65.36598343705435354 ) ;
#28241=DIRECTION ( 'NONE',  ( -0.000000000000000000, -0.000000000000000000, -1.000000000000000000 ) ) ;
#28242=CARTESIAN_POINT ( 'NONE',  ( 50.03867889673311709, 42.05760816978183669, 6.377659838150144402E-18 ) ) ;
#28246=DIRECTION ( 'NONE',  ( 0.000000000000000000, 0.000000000000000000, 1.000000000000000000 ) ) ;
#28249=LINE ( 'NONE', #44432, #9706 ) ;
#28250=EDGE_CURVE ( 'NONE', #15856, #35508, #8037, .T. ) ;
#28259=ORIENTED_EDGE ( 'NONE', *, *, #53488, .F. ) ;
#28263=EDGE_CURVE ( 'NONE', #43897, #58070, #31919, .T. ) ;
#28265=CARTESIAN_POINT ( 'NONE',  ( 15.68296563925497900, 63.09411298019765013, 43.58025477438756923 ) ) ;
#28270=ORIENTED_EDGE ( 'NONE', *, *, #3986, .T. ) ;
#28272=DIRECTION ( 'NONE',  ( -0.000000000000000000, -0.000000000000000000, -1.000000000000000000 ) ) ;
#28283=ORIENTED_EDGE ( 'NONE', *, *, #36950, .F. ) ;
#28284=ADVANCED_FACE ( 'NONE', ( #30535 ), #51984, .T. ) ;
#28302=LINE ( 'NONE', #33598, #68122 ) ;
#28303=ORIENTED_EDGE ( 'NONE', *, *, #21995, .T. ) ;
#28312=VERTEX_POINT ( 'NONE', #63920 ) ;
#28313=DIRECTION ( 'NONE',  ( 0.000000000000000000, 0.000000000000000000, 1.000000000000000000 ) ) ;
#28317=CARTESIAN_POINT ( 'NONE',  ( 61.94551956023253325, 24.58367740818825098, 34.48241823985146937 ) ) ;
#28336=EDGE_CURVE ( 'NONE', #59849, #68407, #25389, .T. ) ;
#28343=CARTESIAN_POINT ( 'NONE',  ( -65.36598343705435354, 0.000000000000000000, 41.38025477438755928 ) ) ;
#28345=VERTEX_POINT ( 'NONE', #46351 ) ;
#28358=VERTEX_POINT ( 'NONE', #43833 ) ;
#28365=CARTESIAN_POINT ( 'NONE',  ( -25.10237775011640338, 1.004202417053489116, 3.061616997868437868E-16 ) ) ;
#28372=ORIENTED_EDGE ( 'NONE', *, *, #25806, .F. ) ;
#28377=FACE_OUTER_BOUND ( 'NONE', #67049, .T. ) ;
#28381=AXIS2_PLACEMENT_3D ( 'NONE', #67435, #19580, #3071 ) ;
#28392=CONICAL_SURFACE ( 'NONE', #20548, 74.95140232871122521, 0.8777644062502172329 ) ;
#28394=CIRCLE ( 'NONE', #37369, 65.00000000000000000 ) ;
#28395=CARTESIAN_POINT ( 'NONE',  ( -37.04655464516844177, 53.85410457537859230, 41.38025477438755928 ) ) ;
#28408=EDGE_CURVE ( 'NONE', #47168, #48718, #12198, .T. ) ;
#28410=FACE_OUTER_BOUND ( 'NONE', #6776, .T. ) ;
#28422=LINE ( 'NONE', #29129, #49721 ) ;
#28426=ORIENTED_EDGE ( 'NONE', *, *, #66678, .T. ) ;
#28436=AXIS2_PLACEMENT_3D ( 'NONE', #33542, #6787, #54970 ) ;
#28440=VECTOR ( 'NONE', #26911, 1000.000000000000000 ) ;
#28444=AXIS2_PLACEMENT_3D ( 'NONE', #47839, #4592, #25722 ) ;
#28446=ORIENTED_EDGE ( 'NONE', *, *, #30493, .F. ) ;
#28454=CARTESIAN_POINT ( 'NONE',  ( -84.49322488516129681, 0.000000000000000000, 43.58025477438756212 ) ) ;
#28460=CARTESIAN_POINT ( 'NONE',  ( 49.76301652092167416, 41.81676920493115546, 170.0000000000000000 ) ) ;
#28461=CARTESIAN_POINT ( 'NONE',  ( 61.28323125814100081, 21.66484633135460669, 40.00000000000003553 ) ) ;
#28470=ORIENTED_EDGE ( 'NONE', *, *, #47792, .T. ) ;
#28484=CARTESIAN_POINT ( 'NONE',  ( 0.000000000000000000, 0.000000000000000000, 43.58025477438756212 ) ) ;
#28485=AXIS2_PLACEMENT_3D ( 'NONE', #30883, #37180, #58626 ) ;
#28491=EDGE_LOOP ( 'NONE', ( #50458, #6771, #5824, #15219, #43264, #15398, #10187, #31283 ) ) ;
#28492=AXIS2_PLACEMENT_3D ( 'NONE', #7267, #55435, #50518 ) ;
#28498=VERTEX_POINT ( 'NONE', #18864 ) ;
#28500=CARTESIAN_POINT ( 'NONE',  ( 31.89651141207616192, -56.63578868294582946, 40.00000000000003553 ) ) ;
#28508=DIRECTION ( 'NONE',  ( -0.000000000000000000, -0.000000000000000000, -1.000000000000000000 ) ) ;
#28512=DIRECTION ( 'NONE',  ( 0.000000000000000000, -0.000000000000000000, 1.000000000000000000 ) ) ;
#28516=VERTEX_POINT ( 'NONE', #19192 ) ;
#28525=DIRECTION ( 'NONE',  ( -0.000000000000000000, -0.000000000000000000, -1.000000000000000000 ) ) ;
#28538=DIRECTION ( 'NONE',  ( -0.3090169943749582759, 0.9510565162951499785, 0.000000000000000000 ) ) ;
#28540=DIRECTION ( 'NONE',  ( 0.000000000000000000, 0.000000000000000000, 1.000000000000000000 ) ) ;
#28542=CARTESIAN_POINT ( 'NONE',  ( -63.73419499958981049, -12.83646726144931449, 0.000000000000000000 ) ) ;
#28547=CONICAL_SURFACE ( 'NONE', #58805, 65.00000000000000000, 0.7853981633974497223 ) ;
#28549=CIRCLE ( 'NONE', #8371, 74.95140232871122521 ) ;
#28552=DIRECTION ( 'NONE',  ( 0.000000000000000000, 0.000000000000000000, 1.000000000000000000 ) ) ;
#28557=LINE ( 'NONE', #6402, #13944 ) ;
#28566=VERTEX_POINT ( 'NONE', #35387 ) ;
#28567=FACE_OUTER_BOUND ( 'NONE', #17069, .T. ) ;
#28569=CARTESIAN_POINT ( 'NONE',  ( 61.28323125814129213, -21.66484633135379667, 170.0000000000000000 ) ) ;
#28577=EDGE_CURVE ( 'NONE', #34081, #58070, #45936, .T. ) ;
#28579=CARTESIAN_POINT ( 'NONE',  ( -65.36598343705435354, 0.000000000000000000, 41.38025477438755928 ) ) ;
#28580=EDGE_LOOP ( 'NONE', ( #3433, #47277, #1995, #8119 ) ) ;
#28587=VECTOR ( 'NONE', #41450, 1000.000000000000000 ) ;
#28598=AXIS2_PLACEMENT_3D ( 'NONE', #5813, #37139, #26932 ) ;
#28599=FACE_OUTER_BOUND ( 'NONE', #16171, .T. ) ;
#28601=AXIS2_PLACEMENT_3D ( 'NONE', #34493, #1775, #1071 ) ;
#28603=FACE_OUTER_BOUND ( 'NONE', #36485, .T. ) ;
#28608=VERTEX_POINT ( 'NONE', #23796 ) ;
#28617=DIRECTION ( 'NONE',  ( 4.852411958229186445E-18, -1.576644219464734062E-18, -1.000000000000000000 ) ) ;
#28622=EDGE_LOOP ( 'NONE', ( #32143, #17002, #52097, #52078 ) ) ;
#28631=ORIENTED_EDGE ( 'NONE', *, *, #45480, .F. ) ;
#28633=CIRCLE ( 'NONE', #3930, 74.95140232871122521 ) ;
#28634=LINE ( 'NONE', #55353, #14737 ) ;
#28636=LINE ( 'NONE', #8225, #19910 ) ;
#28637=CARTESIAN_POINT ( 'NONE',  ( 47.73902449249082025, -57.85799893277825845, 43.58025477438756923 ) ) ;
#28639=LINE ( 'NONE', #23013, #49474 ) ;
#28642=VECTOR ( 'NONE', #33288, 1000.000000000000114 ) ;
#28644=CARTESIAN_POINT ( 'NONE',  ( 39.54205320694412507, -51.58901073076707888, 170.0000000000000000 ) ) ;
#28654=VECTOR ( 'NONE', #20714, 1000.000000000000114 ) ;
#28657=VERTEX_POINT ( 'NONE', #17824 ) ;
#28676=EDGE_CURVE ( 'NONE', #2074, #44289, #11680, .T. ) ;
#28678=CARTESIAN_POINT ( 'NONE',  ( -29.87147652227456263, -74.98256102853682137, 73.58025477438756923 ) ) ;
#28680=B_SPLINE_CURVE_WITH_KNOTS ( 'NONE', 3,
 ( #55429, #28715, #1278, #34350, #55790, #7614 ),
 .UNSPECIFIED., .F., .F.,
 ( 4, 2, 4 ),
 ( 0.03218939915585355971, 0.06469836417558699759, 0.09720732919532043548 ),
 .UNSPECIFIED. ) ;
#28686=DIRECTION ( 'NONE',  ( -0.6910626489868580968, -0.7227948638273978821, 0.000000000000000000 ) ) ;
#28692=EDGE_CURVE ( 'NONE', #44289, #11417, #46271, .T. ) ;
#28699=CARTESIAN_POINT ( 'NONE',  ( -74.69807204964287450, -6.722948167758066695, 43.58025477438756212 ) ) ;
#28710=LINE ( 'NONE', #65649, #18125 ) ;
#28715=CARTESIAN_POINT ( 'NONE',  ( 14.72760812434781208, 30.00634360379971000, 6.893342934305382030 ) ) ;
#28719=ORIENTED_EDGE ( 'NONE', *, *, #48640, .T. ) ;
#28721=CARTESIAN_POINT ( 'NONE',  ( -19.46539569203812903, -15.68752276659308365, 0.000000000000000000 ) ) ;
#28723=DIRECTION ( 'NONE',  ( 0.8584487936018728726, -0.5128992774058949156, 0.000000000000000000 ) ) ;
#28729=DIRECTION ( 'NONE',  ( -0.9510565162951544194, 0.3090169943749446757, 0.000000000000000000 ) ) ;
#28735=DIRECTION ( 'NONE',  ( -1.000000000000000000, 0.000000000000000000, 0.000000000000000000 ) ) ;
#28739=AXIS2_PLACEMENT_3D ( 'NONE', #567, #17073, #22019 ) ;
#28741=CONICAL_SURFACE ( 'NONE', #14123, 65.00000000000000000, 0.7853981633974497223 ) ;
#28747=VERTEX_POINT ( 'NONE', #3710 ) ;
#28749=CARTESIAN_POINT ( 'NONE',  ( 0.000000000000000000, 0.000000000000000000, 41.38025477438755928 ) ) ;
#28751=DIRECTION ( 'NONE',  ( 0.7530714660036195163, -0.6579387259397027066, 0.000000000000000000 ) ) ;
#28755=VECTOR ( 'NONE', #13802, 1000.000000000000227 ) ;
#28756=DIRECTION ( 'NONE',  ( 0.000000000000000000, 0.000000000000000000, 1.000000000000000000 ) ) ;
#28759=EDGE_CURVE ( 'NONE', #3025, #65848, #39119, .T. ) ;
#28761=CARTESIAN_POINT ( 'NONE',  ( -61.41100614348690101, 43.07262267896644659, 43.58025477438756923 ) ) ;
#28766=DIRECTION ( 'NONE',  ( 0.000000000000000000, 0.000000000000000000, 1.000000000000000000 ) ) ;
#28769=VERTEX_POINT ( 'NONE', #54917 ) ;
#28772=EDGE_CURVE ( 'NONE', #6708, #13790, #16660, .T. ) ;
#28775=ORIENTED_EDGE ( 'NONE', *, *, #42928, .F. ) ;
#28790=EDGE_LOOP ( 'NONE', ( #22080, #35868, #16201, #61662, #52881, #43580, #50573, #46480, #2665 ) ) ;
#28798=CARTESIAN_POINT ( 'NONE',  ( -48.12872802574198516, -43.70867239603780519, 170.0000000000000000 ) ) ;
#28806=DIRECTION ( 'NONE',  ( -0.000000000000000000, -0.000000000000000000, -1.000000000000000000 ) ) ;
#28807=EDGE_LOOP ( 'NONE', ( #2770, #46170, #65547, #33079, #47276, #20741, #56907, #30009, #67163, #11498, #26537, #35582, #11119, #31924, #45049, #52777, #8900, #16675, #4001, #27162, #5958, #24627, #39378 ) ) ;
#28813=DIRECTION ( 'NONE',  ( -0.000000000000000000, 0.000000000000000000, -1.000000000000000000 ) ) ;
#28819=DIRECTION ( 'NONE',  ( 0.9839295885986295565, 0.1785568947986370392, -0.000000000000000000 ) ) ;
#28827=EDGE_CURVE ( 'NONE', #42019, #26008, #1123, .T. ) ;
#28828=VERTEX_POINT ( 'NONE', #14104 ) ;
#28829=DIRECTION ( 'NONE',  ( -1.000000000000000000, 0.000000000000000000, 0.000000000000000000 ) ) ;
#28832=CARTESIAN_POINT ( 'NONE',  ( -38.12206941991763642, -16.97122571883291897, 13.79046340968177731 ) ) ;
#28835=ADVANCED_FACE ( 'NONE', ( #67249 ), #46449, .T. ) ;
#28840=DIRECTION ( 'NONE',  ( 1.000000000000000000, 0.000000000000000000, 0.000000000000000000 ) ) ;
#28845=AXIS2_PLACEMENT_3D ( 'NONE', #64015, #42559, #30983 ) ;
#28851=ORIENTED_EDGE ( 'NONE', *, *, #62023, .T. ) ;
#28855=ORIENTED_EDGE ( 'NONE', *, *, #5474, .T. ) ;
#28856=VECTOR ( 'NONE', #29541, 999.9999999999998863 ) ;
#28879=CARTESIAN_POINT ( 'NONE',  ( -1.740765642171157257, 66.62262586640527218, 34.48241795236666718 ) ) ;
#28897=CARTESIAN_POINT ( 'NONE',  ( -4.180838820196593808, 65.23214221112780820, 41.38025477438755928 ) ) ;
#28898=CARTESIAN_POINT ( 'NONE',  ( 0.000000000000000000, 0.000000000000000000, 0.000000000000000000 ) ) ;
#28899=AXIS2_PLACEMENT_3D ( 'NONE', #57313, #56616, #40436 ) ;
#28905=EDGE_LOOP ( 'NONE', ( #181, #21295, #36449, #32047 ) ) ;
#28906=VERTEX_POINT ( 'NONE', #51404 ) ;
#28907=EDGE_CURVE ( 'NONE', #55398, #41122, #50696, .T. ) ;
#28909=CARTESIAN_POINT ( 'NONE',  ( -14.19745703647395274, -56.58567453852795381, 27.58472315868180402 ) ) ;
#28916=DIRECTION ( 'NONE',  ( -1.000000000000000000, 0.000000000000000000, 0.000000000000000000 ) ) ;
#28923=EDGE_CURVE ( 'NONE', #37187, #45254, #12572, .T. ) ;
#28924=ORIENTED_EDGE ( 'NONE', *, *, #67594, .F. ) ;
#28925=EDGE_CURVE ( 'NONE', #62951, #20416, #14192, .T. ) ;
#28926=CARTESIAN_POINT ( 'NONE',  ( -53.31111153860302210, 37.18770477615724701, 170.0000000000000000 ) ) ;
#28927=LINE ( 'NONE', #45084, #55238 ) ;
#28933=VERTEX_POINT ( 'NONE', #18694 ) ;
#28937=AXIS2_PLACEMENT_3D ( 'NONE', #33495, #1124, #13078 ) ;
#28952=EDGE_LOOP ( 'NONE', ( #6768, #56569, #18272, #57058, #38742, #40564, #5527, #39195, #23343 ) ) ;
#28953=VECTOR ( 'NONE', #38714, 1000.000000000000000 ) ;
#28954=ADVANCED_FACE ( 'NONE', ( #46803 ), #19851, .T. ) ;
#28968=DIRECTION ( 'NONE',  ( -0.8090169943749506709, 0.5877852522924686962, 0.000000000000000000 ) ) ;
#28975=VERTEX_POINT ( 'NONE', #13077 ) ;
#28991=ADVANCED_FACE ( 'NONE', ( #40149 ), #61603, .F. ) ;
#28993=AXIS2_PLACEMENT_3D ( 'NONE', #42309, #41617, #67671 ) ;
#28996=CARTESIAN_POINT ( 'NONE',  ( -24.07306065005153783, 53.14126621947204399, 27.58472369383525802 ) ) ;
#28997=EDGE_CURVE ( 'NONE', #27057, #52056, #8138, .T. ) ;
#29015=EDGE_CURVE ( 'NONE', #49177, #29619, #56909, .T. ) ;
#29027=ORIENTED_EDGE ( 'NONE', *, *, #42643, .F. ) ;
#29032=ORIENTED_EDGE ( 'NONE', *, *, #37471, .F. ) ;
#29035=CARTESIAN_POINT ( 'NONE',  ( -18.89790202299119315, -62.20684691518632548, 43.58025477438756923 ) ) ;
#29040=ORIENTED_EDGE ( 'NONE', *, *, #44447, .F. ) ;
#29049=CARTESIAN_POINT ( 'NONE',  ( -34.75846525698938194, -54.92585086258257121, 40.00000000000003553 ) ) ;
#29054=CARTESIAN_POINT ( 'NONE',  ( -18.89790202299119315, -62.20684691518632548, 0.000000000000000000 ) ) ;
#29066=FACE_OUTER_BOUND ( 'NONE', #34808, .T. ) ;
#29070=VERTEX_POINT ( 'NONE', #26046 ) ;
#29079=LINE ( 'NONE', #61758, #22185 ) ;
#29080=ADVANCED_FACE ( 'NONE', ( #36253 ), #2989, .T. ) ;
#29093=CIRCLE ( 'NONE', #9954, 65.00000000000000000 ) ;
#29096=CARTESIAN_POINT ( 'NONE',  ( 28.03312966668345041, -18.20513007408997197, 6.893343212288941757 ) ) ;
#29105=ORIENTED_EDGE ( 'NONE', *, *, #62771, .F. ) ;
#29129=CARTESIAN_POINT ( 'NONE',  ( -53.60725281709859757, -37.40286400928327026, 6.377659838150123602E-18 ) ) ;
#29138=FACE_OUTER_BOUND ( 'NONE', #64749, .T. ) ;
#29140=CARTESIAN_POINT ( 'NONE',  ( 30.58844092318264529, -28.38418505339829778, 13.79046340968177908 ) ) ;
#29144=EDGE_CURVE ( 'NONE', #55150, #3858, #6331, .T. ) ;
#29148=DIRECTION ( 'NONE',  ( 4.492911005741668837E-18, -2.417738509769519932E-18, -1.000000000000000000 ) ) ;
#29149=DIRECTION ( 'NONE',  ( 0.2225209339563184452, -0.9749279121818226201, -5.146830507070804164E-17 ) ) ;
#29156=ORIENTED_EDGE ( 'NONE', *, *, #41530, .F. ) ;
#29162=DIRECTION ( 'NONE',  ( 0.000000000000000000, 0.000000000000000000, 1.000000000000000000 ) ) ;
#29171=CIRCLE ( 'NONE', #43750, 65.00000000000000000 ) ;
#29182=B_SPLINE_CURVE_WITH_KNOTS ( 'NONE', 3,
 ( #54057, #43168, #50201, #64994, #17126, #65337 ),
 .UNSPECIFIED., .F., .F.,
 ( 4, 2, 4 ),
 ( 1.095770181113686320E-06, 0.03239442681617711595, 0.06478775786217312593 ),
 .UNSPECIFIED. ) ;
#29184=DIRECTION ( 'NONE',  ( -0.9009688679024218105, 0.4338837391175525693, 0.000000000000000000 ) ) ;
#29191=CARTESIAN_POINT ( 'NONE',  ( 4.606779575614314837, -24.69646479044436305, 3.061616997868437868E-16 ) ) ;
#29198=CARTESIAN_POINT ( 'NONE',  ( -17.90772993695011905, -72.84144224619156205, 43.58025477438756212 ) ) ;
#29199=ORIENTED_EDGE ( 'NONE', *, *, #61382, .F. ) ;
#29218=AXIS2_PLACEMENT_3D ( 'NONE', #12804, #27924, #23002 ) ;
#29220=CARTESIAN_POINT ( 'NONE',  ( -1.368053059006204331, 58.32353538761584133, 27.58472315868180402 ) ) ;
#29223=CARTESIAN_POINT ( 'NONE',  ( 23.37466857204352522, 46.07527450587193130, 26.66469066592269499 ) ) ;
#29227=EDGE_CURVE ( 'NONE', #16, #58236, #50318, .T. ) ;
#29231=VERTEX_POINT ( 'NONE', #57632 ) ;
#29232=CARTESIAN_POINT ( 'NONE',  ( -31.08850265415324188, 49.36609516667732578, 27.58472315868180402 ) ) ;
#29240=VECTOR ( 'NONE', #67364, 999.9999999999998863 ) ;
#29241=CARTESIAN_POINT ( 'NONE',  ( -42.32797523529131922, 61.85511477251419166, 41.38025477438755928 ) ) ;
#29253=ORIENTED_EDGE ( 'NONE', *, *, #25685, .T. ) ;
#29254=EDGE_CURVE ( 'NONE', #62436, #23495, #64779, .T. ) ;
#29262=EDGE_CURVE ( 'NONE', #23762, #67138, #26313, .T. ) ;
#29263=ORIENTED_EDGE ( 'NONE', *, *, #25723, .T. ) ;
#29264=DIRECTION ( 'NONE',  ( 1.000000000000000000, 0.000000000000000000, 0.000000000000000000 ) ) ;
#29275=DIRECTION ( 'NONE',  ( 1.000000000000000000, 0.000000000000000000, 0.000000000000000000 ) ) ;
#29296=EDGE_LOOP ( 'NONE', ( #44941, #10674, #64325, #36392 ) ) ;
#29303=EDGE_CURVE ( 'NONE', #35812, #61203, #11488, .T. ) ;
#29318=CIRCLE ( 'NONE', #16940, 65.36598343705435354 ) ;
#29327=CARTESIAN_POINT ( 'NONE',  ( -66.25334423260856909, -7.217961380022510198, 34.48241823979542886 ) ) ;
#29347=CARTESIAN_POINT ( 'NONE',  ( 0.000000000000000000, 0.000000000000000000, 0.000000000000000000 ) ) ;
#29350=CARTESIAN_POINT ( 'NONE',  ( 60.82895951008426749, -30.68107831874539926, 41.38025477438755928 ) ) ;
#29356=CIRCLE ( 'NONE', #58558, 25.12245591505646303 ) ;
#29357=VECTOR ( 'NONE', #22309, 1000.000000000000114 ) ;
#29372=EDGE_CURVE ( 'NONE', #61844, #22131, #53603, .T. ) ;
#29378=DIRECTION ( 'NONE',  ( -1.000000000000000000, 0.000000000000000000, 0.000000000000000000 ) ) ;
#29382=ORIENTED_EDGE ( 'NONE', *, *, #4984, .F. ) ;
#29385=FACE_OUTER_BOUND ( 'NONE', #39592, .T. ) ;
#29388=CARTESIAN_POINT ( 'NONE',  ( 8.828807734113995664, 74.48902371486721563, 73.58025477438756923 ) ) ;
#29392=EDGE_CURVE ( 'NONE', #66476, #33038, #10812, .T. ) ;
#29394=EDGE_CURVE ( 'NONE', #4959, #65795, #65682, .T. ) ;
#29395=VECTOR ( 'NONE', #46468, 1000.000000000000000 ) ;
#29397=PLANE ( 'NONE',  #7669 ) ;
#29400=CARTESIAN_POINT ( 'NONE',  ( -2.368959188627552503, -24.88750755625419941, 0.000000000000000000 ) ) ;
#29406=PRODUCT_DEFINITION_SHAPE ( 'NONE', 'NONE',  #39219 ) ;
#29410=CARTESIAN_POINT ( 'NONE',  ( 56.74421265833603201, -32.44697398030824331, 3.125053320693577513E-16 ) ) ;
#29423=CARTESIAN_POINT ( 'NONE',  ( 33.40240406473286328, 1.250000000000020206, 6.893342931450256117 ) ) ;
#29425=CARTESIAN_POINT ( 'NONE',  ( 30.12852347772541961, 58.62603998952764783, 73.58025477438755502 ) ) ;
#29450=EDGE_LOOP ( 'NONE', ( #5057, #8885, #51592, #23627, #35369, #40162, #67236, #43858, #23065 ) ) ;
#29451=VECTOR ( 'NONE', #62201, 1000.000000000000114 ) ;
#29454=EDGE_CURVE ( 'NONE', #20799, #61203, #55852, .T. ) ;
#29462=CARTESIAN_POINT ( 'NONE',  ( -24.39249304643357519, -60.24953346690487166, 170.0000000000000000 ) ) ;
#29467=DIRECTION ( 'NONE',  ( -0.000000000000000000, -0.000000000000000000, -1.000000000000000000 ) ) ;
#29471=EDGE_CURVE ( 'NONE', #8304, #64355, #45948, .T. ) ;
#29479=PLANE ( 'NONE',  #31426 ) ;
#29488=CARTESIAN_POINT ( 'NONE',  ( 74.01791526339553684, 12.16185512414947034, 170.0000000000000000 ) ) ;
#29492=DIRECTION ( 'NONE',  ( -1.000000000000000000, 0.000000000000000000, 0.000000000000000000 ) ) ;
#29493=ORIENTED_EDGE ( 'NONE', *, *, #62408, .T. ) ;
#29498=LINE ( 'NONE', #8757, #29451 ) ;
#29505=AXIS2_PLACEMENT_3D ( 'NONE', #46631, #35050, #3383 ) ;
#29528=CARTESIAN_POINT ( 'NONE',  ( 40.81683905770021425, 8.677580323404230356, 13.79046412291064883 ) ) ;
#29533=ORIENTED_EDGE ( 'NONE', *, *, #46920, .F. ) ;
#29539=AXIS2_PLACEMENT_3D ( 'NONE', #66015, #11823, #38555 ) ;
#29541=DIRECTION ( 'NONE',  ( -0.2660368455666826670, 0.9639628606958513535, 0.000000000000000000 ) ) ;
#29547=VECTOR ( 'NONE', #20167, 1000.000000000000000 ) ;
#29551=ORIENTED_EDGE ( 'NONE', *, *, #17779, .T. ) ;
#29568=CARTESIAN_POINT ( 'NONE',  ( -21.93488196095011844, 35.49895255660060656, 13.79046340968177908 ) ) ;
#29573=CARTESIAN_POINT ( 'NONE',  ( 64.52696037203357093, 10.43950074664854633, 41.38025477438755928 ) ) ;
#29574=DIRECTION ( 'NONE',  ( -0.000000000000000000, -0.000000000000000000, -1.000000000000000000 ) ) ;
#29579=ORIENTED_EDGE ( 'NONE', *, *, #63356, .F. ) ;
#29581=CARTESIAN_POINT ( 'NONE',  ( -65.00200000000002376, 1.250000000000021982, 3.061616997868437868E-16 ) ) ;
#29582=CARTESIAN_POINT ( 'NONE',  ( 17.14961149657550976, 48.73599200008756327, 26.66469104408689716 ) ) ;
#29600=CYLINDRICAL_SURFACE ( 'NONE', #42371, 65.00000000000000000 ) ;
#29612=EDGE_CURVE ( 'NONE', #60419, #23236, #53528, .T. ) ;
#29614=VERTEX_POINT ( 'NONE', #55898 ) ;
#29619=VERTEX_POINT ( 'NONE', #56235 ) ;
#29626=ORIENTED_EDGE ( 'NONE', *, *, #15378, .T. ) ;
#29636=AXIS2_PLACEMENT_3D ( 'NONE', #27661, #590, #58976 ) ;
#29650=VECTOR ( 'NONE', #13774, 1000.000000000000000 ) ;
#29654=VERTEX_POINT ( 'NONE', #34797 ) ;
#29661=VECTOR ( 'NONE', #22919, 1000.000000000000000 ) ;
#29668=ORIENTED_EDGE ( 'NONE', *, *, #61211, .F. ) ;
#29685=CARTESIAN_POINT ( 'NONE',  ( -19.44450032618849633, -27.18813209818722498, 6.893343212288935540 ) ) ;
#29690=EDGE_LOOP ( 'NONE', ( #7831, #20092, #27375, #25900 ) ) ;
#29692=CARTESIAN_POINT ( 'NONE',  ( 70.21761529798025947, 26.35311180610075610, 43.58025477438756212 ) ) ;
#29698=EDGE_LOOP ( 'NONE', ( #3133, #43919, #26498, #8269 ) ) ;
#29700=DIRECTION ( 'NONE',  ( 0.000000000000000000, 0.000000000000000000, 1.000000000000000000 ) ) ;
#29701=EDGE_CURVE ( 'NONE', #28566, #3016, #39718, .T. ) ;
#29703=DIRECTION ( 'NONE',  ( -0.000000000000000000, -0.000000000000000000, -1.000000000000000000 ) ) ;
#29704=ORIENTED_EDGE ( 'NONE', *, *, #52039, .F. ) ;
#29720=CARTESIAN_POINT ( 'NONE',  ( -2.967675169455163520, 38.21895468312379052, 13.32819299319723783 ) ) ;
#29730=CARTESIAN_POINT ( 'NONE',  ( -13.24252603915608617, 63.63674649211943546, 170.0000000000000000 ) ) ;
#29731=DIRECTION ( 'NONE',  ( -0.08963930890344087854, 0.9959742939952382912, 0.000000000000000000 ) ) ;
#29732=ADVANCED_FACE ( 'NONE', ( #14376 ), #8406, .T. ) ;
#29737=AXIS2_PLACEMENT_3D ( 'NONE', #41151, #3177, #62612 ) ;
#29745=AXIS2_PLACEMENT_3D ( 'NONE', #69110, #43760, #42392 ) ;
#29753=VERTEX_POINT ( 'NONE', #51322 ) ;
#29766=PLANE ( 'NONE',  #44177 ) ;
#29769=CARTESIAN_POINT ( 'NONE',  ( -16.68907004672388084, 73.11959341363670717, 0.000000000000000000 ) ) ;
#29783=VERTEX_POINT ( 'NONE', #26311 ) ;
#29786=CARTESIAN_POINT ( 'NONE',  ( 0.000000000000000000, 0.000000000000000000, 170.0000000000000000 ) ) ;
#29787=ORIENTED_EDGE ( 'NONE', *, *, #64005, .F. ) ;
#29793=FACE_OUTER_BOUND ( 'NONE', #6145, .T. ) ;
#29794=EDGE_CURVE ( 'NONE', #62258, #3570, #20677, .T. ) ;
#29797=DIRECTION ( 'NONE',  ( 0.000000000000000000, 0.000000000000000000, 1.000000000000000000 ) ) ;
#29800=CARTESIAN_POINT ( 'NONE',  ( -34.96012151086435438, -55.23134702900938464, 43.58025477438756212 ) ) ;
#29806=ORIENTED_EDGE ( 'NONE', *, *, #40488, .T. ) ;
#29807=ORIENTED_EDGE ( 'NONE', *, *, #59061, .F. ) ;
#29812=ORIENTED_EDGE ( 'NONE', *, *, #64229, .T. ) ;
#29827=DIRECTION ( 'NONE',  ( 0.9959742939952382912, 0.08963930890344087854, 0.000000000000000000 ) ) ;
#29830=EDGE_LOOP ( 'NONE', ( #7952, #39695, #5424, #67549 ) ) ;
#29836=ORIENTED_EDGE ( 'NONE', *, *, #56025, .F. ) ;
#29837=CARTESIAN_POINT ( 'NONE',  ( 56.56044447577782108, 35.24940721789563725, 34.48241823993598132 ) ) ;
#29848=ORIENTED_EDGE ( 'NONE', *, *, #68784, .T. ) ;
#29849=PLANE ( 'NONE',  #54423 ) ;
#29851=CARTESIAN_POINT ( 'NONE',  ( -20.93485882276935328, -13.66498028065569059, 0.000000000000000000 ) ) ;
#29864=EDGE_CURVE ( 'NONE', #32511, #39395, #7560, .T. ) ;
#29866=CARTESIAN_POINT ( 'NONE',  ( -72.57286576968782299, -18.73210786364450442, 41.38025477438755928 ) ) ;
#29874=PRESENTATION_STYLE_ASSIGNMENT (( #14396 ) ) ;
#29877=LINE ( 'NONE', #67185, #51488 ) ;
#29897=EDGE_LOOP ( 'NONE', ( #48694, #13318, #35426, #1171 ) ) ;
#29899=DIRECTION ( 'NONE',  ( 1.000000000000000000, 0.000000000000000000, -0.000000000000000000 ) ) ;
#29911=ORIENTED_EDGE ( 'NONE', *, *, #47466, .F. ) ;
#29915=ADVANCED_FACE ( 'NONE', ( #47741 ), #69204, .T. ) ;
#29921=CYLINDRICAL_SURFACE ( 'NONE', #66922, 10.00000000000000000 ) ;
#29927=CARTESIAN_POINT ( 'NONE',  ( -36.53690438256410289, 73.43472186181504924, 133.5802547743875550 ) ) ;
#29935=ORIENTED_EDGE ( 'NONE', *, *, #19128, .T. ) ;
#29942=DIRECTION ( 'NONE',  ( 0.000000000000000000, 0.000000000000000000, 1.000000000000000000 ) ) ;
#29947=CARTESIAN_POINT ( 'NONE',  ( -72.62976060914719767, -18.74780984163136210, 43.58025477438756212 ) ) ;
#29956=ORIENTED_EDGE ( 'NONE', *, *, #4928, .T. ) ;
#29970=PLANE ( 'NONE',  #8153 ) ;
#29981=CARTESIAN_POINT ( 'NONE',  ( 0.000000000000000000, 0.000000000000000000, 41.38025477438755928 ) ) ;
#29989=DIRECTION ( 'NONE',  ( 0.000000000000000000, 0.000000000000000000, 1.000000000000000000 ) ) ;
#29991=VECTOR ( 'NONE', #14216, 999.9999999999998863 ) ;
#29994=CARTESIAN_POINT ( 'NONE',  ( -8.062763356759356626, -40.94272338264845956, 13.79046412294881208 ) ) ;
#29995=DIRECTION ( 'NONE',  ( 0.9362348706397417564, -0.3513748240813305279, 0.000000000000000000 ) ) ;
#30006=ADVANCED_FACE ( 'NONE', ( #25630 ), #47064, .T. ) ;
#30009=ORIENTED_EDGE ( 'NONE', *, *, #68461, .F. ) ;
#30011=ORIENTED_EDGE ( 'NONE', *, *, #42666, .F. ) ;
#30025=CARTESIAN_POINT ( 'NONE',  ( -60.67627457812066183, -44.08389392193601708, 0.000000000000000000 ) ) ;
#30028=EDGE_CURVE ( 'NONE', #30365, #21034, #34274, .T. ) ;
#30035=CIRCLE ( 'NONE', #50264, 74.95140232871122521 ) ;
#30039=DIRECTION ( 'NONE',  ( -0.000000000000000000, -0.000000000000000000, -1.000000000000000000 ) ) ;
#30044=ORIENTED_EDGE ( 'NONE', *, *, #60421, .T. ) ;
#30045=AXIS2_PLACEMENT_3D ( 'NONE', #51746, #51058, #19040 ) ;
#30048=CARTESIAN_POINT ( 'NONE',  ( -0.6225858807736643907, -41.72441896235496728, 13.79046412284827383 ) ) ;
#30051=LINE ( 'NONE', #34980, #45806 ) ;
#30052=EDGE_CURVE ( 'NONE', #17792, #3940, #67111, .T. ) ;
#30060=ORIENTED_EDGE ( 'NONE', *, *, #21024, .T. ) ;
#30063=FACE_OUTER_BOUND ( 'NONE', #13164, .T. ) ;
#30064=DIRECTION ( 'NONE',  ( 1.000000000000000000, 0.000000000000000000, 0.000000000000000000 ) ) ;
#30080=ORIENTED_EDGE ( 'NONE', *, *, #6132, .F. ) ;
#30081=CARTESIAN_POINT ( 'NONE',  ( 13.24564585880038514, 63.65041531508843065, 170.0000000000000000 ) ) ;
#30082=VERTEX_POINT ( 'NONE', #5868 ) ;
#30083=ORIENTED_EDGE ( 'NONE', *, *, #5686, .F. ) ;
#30086=CARTESIAN_POINT ( 'NONE',  ( -84.49322488516129681, 0.000000000000000000, 43.58025477438756212 ) ) ;
#30087=CARTESIAN_POINT ( 'NONE',  ( 0.000000000000000000, 0.000000000000000000, 41.38025477438755928 ) ) ;
#30096=EDGE_LOOP ( 'NONE', ( #25552, #1199, #38398, #15111 ) ) ;
#30097=AXIS2_PLACEMENT_3D ( 'NONE', #33943, #24435, #34292 ) ;
#30106=VERTEX_POINT ( 'NONE', #22407 ) ;
#30124=ORIENTED_EDGE ( 'NONE', *, *, #13414, .F. ) ;
#30133=SHAPE_DEFINITION_REPRESENTATION ( #29406, #55473 ) ;
#30137=LINE ( 'NONE', #51588, #5376 ) ;
#30140=DIRECTION ( 'NONE',  ( -0.000000000000000000, -0.000000000000000000, 1.000000000000000000 ) ) ;
#30141=ORIENTED_EDGE ( 'NONE', *, *, #19954, .F. ) ;
#30143=EDGE_CURVE ( 'NONE', #48419, #53230, #8230, .T. ) ;
#30146=ORIENTED_EDGE ( 'NONE', *, *, #32245, .F. ) ;
#30154=DIRECTION ( 'NONE',  ( -0.000000000000000000, -0.000000000000000000, -1.000000000000000000 ) ) ;
#30161=VERTEX_POINT ( 'NONE', #25108 ) ;
#30173=CARTESIAN_POINT ( 'NONE',  ( -50.92620509423088038, 55.07344309828770434, 43.58025477438756212 ) ) ;
#30182=LINE ( 'NONE', #18930, #9024 ) ;
#30187=ORIENTED_EDGE ( 'NONE', *, *, #31366, .F. ) ;
#30195=CARTESIAN_POINT ( 'NONE',  ( 26.12852347772543737, 70.00000000000000000, 77.58025477438755502 ) ) ;
#30203=AXIS2_PLACEMENT_3D ( 'NONE', #11905, #31982, #48137 ) ;
#30205=DIRECTION ( 'NONE',  ( 1.000000000000000000, 0.000000000000000000, 0.000000000000000000 ) ) ;
#30211=CARTESIAN_POINT ( 'NONE',  ( -61.29635759142585982, -21.66977272663580578, 41.38025477438755928 ) ) ;
#30222=B_SPLINE_CURVE_WITH_KNOTS ( 'NONE', 3,
 ( #1820, #61250, #56308, #61596, #13070, #65843 ),
 .UNSPECIFIED., .F., .F.,
 ( 4, 2, 4 ),
 ( 1.095770181105393655E-06, 0.03239442681617711595, 0.06478775786217312593 ),
 .UNSPECIFIED. ) ;
#30223=CARTESIAN_POINT ( 'NONE',  ( -65.36598343705435354, 0.000000000000000000, 41.38025477438755928 ) ) ;
#30229=ORIENTED_EDGE ( 'NONE', *, *, #19669, .F. ) ;
#30241=DIRECTION ( 'NONE',  ( 0.8345732537212999791, 0.5508969814521065267, -0.000000000000000000 ) ) ;
#30244=DIRECTION ( 'NONE',  ( -0.000000000000000000, 1.000000000000000000, -0.000000000000000000 ) ) ;
#30247=ORIENTED_EDGE ( 'NONE', *, *, #57323, .F. ) ;
#30253=CARTESIAN_POINT ( 'NONE',  ( 50.03867889673372105, -42.05760816978111194, 41.38025477438755928 ) ) ;
#30273=ORIENTED_EDGE ( 'NONE', *, *, #22726, .F. ) ;
#30275=VERTEX_POINT ( 'NONE', #13085 ) ;
#30277=EDGE_CURVE ( 'NONE', #12796, #21766, #43469, .T. ) ;
#30280=CARTESIAN_POINT ( 'NONE',  ( -1.666933348991701536, -64.97862212458815634, 170.0000000000000000 ) ) ;
#30298=CARTESIAN_POINT ( 'NONE',  ( 24.36509522349078338, -70.94296747916756374, 170.0000000000000000 ) ) ;
#30304=ORIENTED_EDGE ( 'NONE', *, *, #21984, .F. ) ;
#30305=EDGE_LOOP ( 'NONE', ( #56024, #26430, #49452, #27818 ) ) ;
#30313=ORIENTED_EDGE ( 'NONE', *, *, #65850, .F. ) ;
#30314=CARTESIAN_POINT ( 'NONE',  ( 70.21761529798025947, 26.35311180610075610, 0.000000000000000000 ) ) ;
#30318=ORIENTED_EDGE ( 'NONE', *, *, #32168, .F. ) ;
#30324=AXIS2_PLACEMENT_3D ( 'NONE', #54733, #53688, #5508 ) ;
#30331=EDGE_CURVE ( 'NONE', #51505, #18983, #46113, .T. ) ;
#30343=LINE ( 'NONE', #36657, #19793 ) ;
#30349=DIRECTION ( 'NONE',  ( -0.9749279121818259508, 0.2225209339563042066, 5.102127870520021228E-18 ) ) ;
#30352=VERTEX_POINT ( 'NONE', #14796 ) ;
#30355=EDGE_CURVE ( 'NONE', #31287, #28498, #64453, .T. ) ;
#30356=CARTESIAN_POINT ( 'NONE',  ( 0.000000000000000000, 0.000000000000000000, 40.00000000000003553 ) ) ;
#30365=VERTEX_POINT ( 'NONE', #62299 ) ;
#30367=CARTESIAN_POINT ( 'NONE',  ( -7.486743542470078339, 64.58150799671128084, 170.0000000000000000 ) ) ;
#30368=CYLINDRICAL_SURFACE ( 'NONE', #13925, 65.00000000000000000 ) ;
#30374=CARTESIAN_POINT ( 'NONE',  ( 24.91130694661013578, 3.250319586706704733, 0.000000000000000000 ) ) ;
#30375=FACE_OUTER_BOUND ( 'NONE', #49876, .T. ) ;
#30384=CARTESIAN_POINT ( 'NONE',  ( 44.01696072965949469, 47.84694004974210912, 170.0000000000000000 ) ) ;
#30390=ADVANCED_FACE ( 'NONE', ( #3222 ), #36259, .T. ) ;
#30394=ORIENTED_EDGE ( 'NONE', *, *, #9484, .T. ) ;
#30399=ORIENTED_EDGE ( 'NONE', *, *, #55850, .F. ) ;
#30401=DIRECTION ( 'NONE',  ( 0.9639628606958512425, 0.2660368455666826670, -0.000000000000000000 ) ) ;
#30411=EDGE_CURVE ( 'NONE', #35197, #10115, #38411, .T. ) ;
#30416=DIRECTION ( 'NONE',  ( 0.000000000000000000, 0.000000000000000000, 1.000000000000000000 ) ) ;
#30417=ORIENTED_EDGE ( 'NONE', *, *, #32310, .F. ) ;
#30440=EDGE_CURVE ( 'NONE', #53534, #23514, #18702, .T. ) ;
#30441=CARTESIAN_POINT ( 'NONE',  ( 30.12852347772543027, 100.0000000000000000, 73.58025477438755502 ) ) ;
#30444=VERTEX_POINT ( 'NONE', #29947 ) ;
#30447=LINE ( 'NONE', #4741, #7197 ) ;
#30448=CARTESIAN_POINT ( 'NONE',  ( 0.000000000000000000, 0.000000000000000000, 43.58025477438756212 ) ) ;
#30456=VECTOR ( 'NONE', #51928, 1000.000000000000000 ) ;
#30458=CARTESIAN_POINT ( 'NONE',  ( 23.17627457812085723, 71.32923872213659422, 43.58025477438756212 ) ) ;
#30460=LINE ( 'NONE', #14625, #61231 ) ;
#30470=DIRECTION ( 'NONE',  ( -0.9510565162951545304, 0.3090169943749447312, 2.500042656554810833E-16 ) ) ;
#30471=CARTESIAN_POINT ( 'NONE',  ( -58.00979178563854077, 29.32343869649098878, 170.0000000000000000 ) ) ;
#30474=EDGE_LOOP ( 'NONE', ( #48864, #17604, #38930, #5085 ) ) ;
#30476=ORIENTED_EDGE ( 'NONE', *, *, #12104, .T. ) ;
#30479=ORIENTED_EDGE ( 'NONE', *, *, #26575, .F. ) ;
#30489=ORIENTED_EDGE ( 'NONE', *, *, #27685, .F. ) ;
#30491=FACE_OUTER_BOUND ( 'NONE', #65876, .T. ) ;
#30492=VERTEX_POINT ( 'NONE', #48507 ) ;
#30493=EDGE_CURVE ( 'NONE', #30352, #46155, #59424, .T. ) ;
#30500=DIRECTION ( 'NONE',  ( -1.000000000000000000, 0.000000000000000000, 1.156482317317871478E-16 ) ) ;
#30523=EDGE_CURVE ( 'NONE', #21329, #50834, #21451, .T. ) ;
#30527=ORIENTED_EDGE ( 'NONE', *, *, #60421, .F. ) ;
#30534=CARTESIAN_POINT ( 'NONE',  ( 69.68177367721139603, 20.52767805628179332, 170.0000000000000000 ) ) ;
#30535=FACE_OUTER_BOUND ( 'NONE', #52998, .T. ) ;
#30536=FACE_OUTER_BOUND ( 'NONE', #10870, .T. ) ;
#30540=ORIENTED_EDGE ( 'NONE', *, *, #33035, .T. ) ;
#30548=CARTESIAN_POINT ( 'NONE',  ( 19.25636636730773077, 33.14646320116730749, 13.32819397642333392 ) ) ;
#30555=EDGE_CURVE ( 'NONE', #2845, #56665, #697, .T. ) ;
#30556=DIRECTION ( 'NONE',  ( 1.000000000000000000, 0.000000000000000000, 0.000000000000000000 ) ) ;
#30565=AXIS2_PLACEMENT_3D ( 'NONE', #25511, #31463, #37416 ) ;
#30567=AXIS2_PLACEMENT_3D ( 'NONE', #42562, #20079, #37272 ) ;
#30568=ADVANCED_FACE ( 'NONE', ( #17923 ), #22149, .F. ) ;
#30569=DIRECTION ( 'NONE',  ( -0.4338837391175656699, 0.9009688679024155933, 0.000000000000000000 ) ) ;
#30576=DIRECTION ( 'NONE',  ( 0.000000000000000000, 0.000000000000000000, 1.000000000000000000 ) ) ;
#30586=DIRECTION ( 'NONE',  ( 0.000000000000000000, 0.000000000000000000, 1.000000000000000000 ) ) ;
#30591=CARTESIAN_POINT ( 'NONE',  ( 0.000000000000000000, 0.000000000000000000, 41.38025477438755928 ) ) ;
#30596=LINE ( 'NONE', #3863, #42081 ) ;
#30602=CARTESIAN_POINT ( 'NONE',  ( 0.000000000000000000, 0.000000000000000000, 40.00000000000003553 ) ) ;
#30608=VECTOR ( 'NONE', #64666, 999.9999999999998863 ) ;
#30610=DIRECTION ( 'NONE',  ( -1.000000000000000000, 0.000000000000000000, 0.000000000000000000 ) ) ;
#30618=CARTESIAN_POINT ( 'NONE',  ( 74.01791526339567895, -12.16185512414844716, 170.0000000000000000 ) ) ;
#30619=EDGE_LOOP ( 'NONE', ( #66928, #57278, #61417, #6137 ) ) ;
#30632=ORIENTED_EDGE ( 'NONE', *, *, #704, .F. ) ;
#30634=CARTESIAN_POINT ( 'NONE',  ( 53.32245423372560111, 37.19594572654715137, 170.0000000000000000 ) ) ;
#30635=CARTESIAN_POINT ( 'NONE',  ( 21.27121078971613244, 61.42097029141973508, 40.00000000000003553 ) ) ;
#30658=LINE ( 'NONE', #3925, #68496 ) ;
#30665=EDGE_CURVE ( 'NONE', #35812, #37212, #7411, .T. ) ;
#30686=DIRECTION ( 'NONE',  ( 0.5877852522924685852, 0.8090169943749507819, 0.000000000000000000 ) ) ;
#30694=ORIENTED_EDGE ( 'NONE', *, *, #47021, .F. ) ;
#30695=AXIS2_PLACEMENT_3D ( 'NONE', #8147, #18350, #61947 ) ;
#30698=ORIENTED_EDGE ( 'NONE', *, *, #4928, .F. ) ;
#30700=ORIENTED_EDGE ( 'NONE', *, *, #31652, .T. ) ;
#30712=ORIENTED_EDGE ( 'NONE', *, *, #36931, .F. ) ;
#30716=DIRECTION ( 'NONE',  ( -0.000000000000000000, -0.000000000000000000, -1.000000000000000000 ) ) ;
#30717=DIRECTION ( 'NONE',  ( -0.8090169943749422332, -0.5877852522924802425, 0.000000000000000000 ) ) ;
#30719=LINE ( 'NONE', #19114, #6026 ) ;
#30728=DIRECTION ( 'NONE',  ( 0.8090169943749422332, 0.5877852522924802425, 0.000000000000000000 ) ) ;
#30732=ADVANCED_FACE ( 'NONE', ( #60127 ), #17572, .F. ) ;
#30741=CARTESIAN_POINT ( 'NONE',  ( -74.52723870109939242, -7.962625360375267469, 41.38025477438755928 ) ) ;
#30742=EDGE_LOOP ( 'NONE', ( #44080, #33997, #50143, #20790 ) ) ;
#30743=CARTESIAN_POINT ( 'NONE',  ( 0.000000000000000000, 0.000000000000000000, 170.0000000000000000 ) ) ;
#30747=CIRCLE ( 'NONE', #30695, 24.99999999999985434 ) ;
#30748=CARTESIAN_POINT ( 'NONE',  ( -9.273616082387997395, -77.77273080542778416, 73.58025477438756923 ) ) ;
#30749=CARTESIAN_POINT ( 'NONE',  ( -48.12872802574198516, -43.70867239603780519, 43.58025477438756923 ) ) ;
#30760=AXIS2_PLACEMENT_3D ( 'NONE', #3882, #20061, #37600 ) ;
#30761=EDGE_LOOP ( 'NONE', ( #14816, #32384, #2876, #65530 ) ) ;
#30764=VECTOR ( 'NONE', #28751, 1000.000000000000000 ) ;
#30767=DIRECTION ( 'NONE',  ( -0.000000000000000000, 0.000000000000000000, -1.000000000000000000 ) ) ;
#30773=VECTOR ( 'NONE', #40145, 1000.000000000000000 ) ;
#30776=FACE_OUTER_BOUND ( 'NONE', #45975, .T. ) ;
#30777=DIRECTION ( 'NONE',  ( 1.000000000000000000, 0.000000000000000000, 0.000000000000000000 ) ) ;
#30778=DIRECTION ( 'NONE',  ( -0.000000000000000000, -0.000000000000000000, -1.000000000000000000 ) ) ;
#30783=ORIENTED_EDGE ( 'NONE', *, *, #16181, .T. ) ;
#30799=FACE_OUTER_BOUND ( 'NONE', #22294, .T. ) ;
#30802=AXIS2_PLACEMENT_3D ( 'NONE', #30025, #30717, #68353 ) ;
#30820=ORIENTED_EDGE ( 'NONE', *, *, #19321, .F. ) ;
#30823=EDGE_CURVE ( 'NONE', #31341, #6300, #35490, .T. ) ;
#30828=ORIENTED_EDGE ( 'NONE', *, *, #44235, .T. ) ;
#30832=VERTEX_POINT ( 'NONE', #20339 ) ;
#30844=ORIENTED_EDGE ( 'NONE', *, *, #18886, .F. ) ;
#30845=CARTESIAN_POINT ( 'NONE',  ( -34.75846525699014933, 54.92585086258208804, 170.0000000000000000 ) ) ;
#30850=DIRECTION ( 'NONE',  ( 0.08963930890342655666, 0.9959742939952397345, 5.102127870520019688E-18 ) ) ;
#30853=ORIENTED_EDGE ( 'NONE', *, *, #48812, .T. ) ;
#30860=VECTOR ( 'NONE', #45974, 999.9999999999998863 ) ;
#30863=VECTOR ( 'NONE', #58171, 1000.000000000000000 ) ;
#30873=EDGE_CURVE ( 'NONE', #10821, #44801, #15068, .T. ) ;
#30874=CARTESIAN_POINT ( 'NONE',  ( -52.00772213768630081, 26.43299429372219578, 27.58472315868181113 ) ) ;
#30878=EDGE_LOOP ( 'NONE', ( #10306, #38321, #22065, #48487 ) ) ;
#30879=DIRECTION ( 'NONE',  ( -0.000000000000000000, 0.000000000000000000, -1.000000000000000000 ) ) ;
#30883=CARTESIAN_POINT ( 'NONE',  ( 0.000000000000000000, 0.000000000000000000, 40.00000000000003553 ) ) ;
#30885=DIRECTION ( 'NONE',  ( 0.8584487936018655452, 0.5128992774059071280, 0.000000000000000000 ) ) ;
#30892=ORIENTED_EDGE ( 'NONE', *, *, #31356, .T. ) ;
#30898=CARTESIAN_POINT ( 'NONE',  ( 25.57615758091871427, 44.89060318276072792, 26.66469104408690427 ) ) ;
#30904=VECTOR ( 'NONE', #52808, 1000.000000000000000 ) ;
#30922=VERTEX_POINT ( 'NONE', #49478 ) ;
#30926=LINE ( 'NONE', #62225, #38889 ) ;
#30929=EDGE_CURVE ( 'NONE', #24824, #66476, #62483, .T. ) ;
#30944=VECTOR ( 'NONE', #26280, 1000.000000000000000 ) ;
#30945=ORIENTED_EDGE ( 'NONE', *, *, #26202, .T. ) ;
#30960=CARTESIAN_POINT ( 'NONE',  ( -42.36049017605964195, 61.90437280228238848, 43.58025477438756923 ) ) ;
#30962=CARTESIAN_POINT ( 'NONE',  ( 21.80334764943355452, -25.33568884114822239, 6.893342937333462928 ) ) ;
#30965=VERTEX_POINT ( 'NONE', #61778 ) ;
#30983=DIRECTION ( 'NONE',  ( 1.000000000000000000, 0.000000000000000000, 0.000000000000000000 ) ) ;
#30985=CARTESIAN_POINT ( 'NONE',  ( -46.45214326556835971, 35.29454257130760908, 27.58472315868180402 ) ) ;
#30988=ORIENTED_EDGE ( 'NONE', *, *, #42196, .T. ) ;
#30995=DIRECTION ( 'NONE',  ( -0.000000000000000000, -0.000000000000000000, -1.000000000000000000 ) ) ;
#30997=ORIENTED_EDGE ( 'NONE', *, *, #25806, .T. ) ;
#31003=CARTESIAN_POINT ( 'NONE',  ( 64.97411640938599930, 37.36411256620309018, 41.38025477438755928 ) ) ;
#31007=AXIS2_PLACEMENT_3D ( 'NONE', #53957, #5786, #49032 ) ;
#31009=VERTEX_POINT ( 'NONE', #2364 ) ;
#31013=CIRCLE ( 'NONE', #668, 65.00000000000000000 ) ;
#31026=ORIENTED_EDGE ( 'NONE', *, *, #51372, .T. ) ;
#31031=CARTESIAN_POINT ( 'NONE',  ( -6.774725108395606377, -24.06456107444444825, 0.000000000000000000 ) ) ;
#31032=DIRECTION ( 'NONE',  ( 1.000000000000000000, 0.000000000000000000, 0.000000000000000000 ) ) ;
#31034=CARTESIAN_POINT ( 'NONE',  ( 60.40479419793796012, -24.00543350795315334, 40.00000000000003553 ) ) ;
#31048=EDGE_CURVE ( 'NONE', #27671, #45386, #19216, .T. ) ;
#31070=AXIS2_PLACEMENT_3D ( 'NONE', #59146, #10966, #48573 ) ;
#31071=CYLINDRICAL_SURFACE ( 'NONE', #26168, 65.00000000000000000 ) ;
#31073=EDGE_CURVE ( 'NONE', #33925, #8790, #30137, .T. ) ;
#31093=VERTEX_POINT ( 'NONE', #9027 ) ;
#31098=VECTOR ( 'NONE', #55789, 1000.000000000000227 ) ;
#31099=VERTEX_POINT ( 'NONE', #36441 ) ;
#31101=DIRECTION ( 'NONE',  ( -0.000000000000000000, -0.000000000000000000, -1.000000000000000000 ) ) ;
#31106=DIRECTION ( 'NONE',  ( 0.7530714660036195163, -0.6579387259397027066, 0.000000000000000000 ) ) ;
#31112=CIRCLE ( 'NONE', #46969, 65.00000000000000000 ) ;
#31117=DIRECTION ( 'NONE',  ( -0.9510565162951499785, -0.3090169943749582204, 0.000000000000000000 ) ) ;
#31120=FACE_OUTER_BOUND ( 'NONE', #64572, .T. ) ;
#31123=ORIENTED_EDGE ( 'NONE', *, *, #55332, .F. ) ;
#31128=DIRECTION ( 'NONE',  ( -0.9009688679024218105, 0.4338837391175525693, 0.000000000000000000 ) ) ;
#31137=ORIENTED_EDGE ( 'NONE', *, *, #61076, .F. ) ;
#31138=B_SPLINE_CURVE_WITH_KNOTS ( 'NONE', 3,
 ( #65830, #22550, #391, #38378 ),
 .UNSPECIFIED., .F., .F.,
 ( 4, 4 ),
 ( 0.1259919275528357530, 0.1829744153748744939 ),
 .UNSPECIFIED. ) ;
#31139=ORIENTED_EDGE ( 'NONE', *, *, #28925, .T. ) ;
#31142=DIRECTION ( 'NONE',  ( 1.000000000000000000, 0.000000000000000000, 0.000000000000000000 ) ) ;
#31145=EDGE_CURVE ( 'NONE', #35508, #34656, #33247, .T. ) ;
#31146=VECTOR ( 'NONE', #54056, 1000.000000000000114 ) ;
#31150=ORIENTED_EDGE ( 'NONE', *, *, #45340, .T. ) ;
#31152=ORIENTED_EDGE ( 'NONE', *, *, #13797, .F. ) ;
#31166=CARTESIAN_POINT ( 'NONE',  ( 32.67633850029795184, 58.08495024160666276, 34.48241795236665297 ) ) ;
#31178=CARTESIAN_POINT ( 'NONE',  ( -40.24154210098712525, -63.23235722614506216, 41.38025477438755928 ) ) ;
#31189=DIRECTION ( 'NONE',  ( 1.000000000000000000, 0.000000000000000000, 0.000000000000000000 ) ) ;
#31190=CARTESIAN_POINT ( 'NONE',  ( 0.000000000000000000, 0.000000000000000000, 0.000000000000000000 ) ) ;
#31192=CARTESIAN_POINT ( 'NONE',  ( 0.000000000000000000, 0.000000000000000000, 41.38025477438755928 ) ) ;
#31208=VERTEX_POINT ( 'NONE', #38871 ) ;
#31209=CARTESIAN_POINT ( 'NONE',  ( 0.000000000000000000, 0.000000000000000000, 170.0000000000000000 ) ) ;
#31210=ADVANCED_FACE ( 'NONE', ( #43770 ), #11414, .T. ) ;
#31215=DIRECTION ( 'NONE',  ( -0.000000000000000000, -0.000000000000000000, -1.000000000000000000 ) ) ;
#31217=ORIENTED_EDGE ( 'NONE', *, *, #37302, .F. ) ;
#31235=DIRECTION ( 'NONE',  ( -0.000000000000000000, -0.000000000000000000, -1.000000000000000000 ) ) ;
#31239=CARTESIAN_POINT ( 'NONE',  ( -34.96012151086436859, -55.23134702900938464, 41.38025477438755928 ) ) ;
#31244=EDGE_LOOP ( 'NONE', ( #28851, #6144, #60718, #13238 ) ) ;
#31255=ORIENTED_EDGE ( 'NONE', *, *, #24546, .F. ) ;
#31257=DIRECTION ( 'NONE',  ( 0.1342332658176522420, 0.9909497617679352555, -0.000000000000000000 ) ) ;
#31268=ORIENTED_EDGE ( 'NONE', *, *, #32168, .T. ) ;
#31277=ORIENTED_EDGE ( 'NONE', *, *, #63552, .F. ) ;
#31283=ORIENTED_EDGE ( 'NONE', *, *, #52628, .T. ) ;
#31287=VERTEX_POINT ( 'NONE', #40254 ) ;
#31296=DIRECTION ( 'NONE',  ( 1.000000000000000000, 0.000000000000000000, 0.000000000000000000 ) ) ;
#31299=FACE_OUTER_BOUND ( 'NONE', #15517, .T. ) ;
#31300=ORIENTED_EDGE ( 'NONE', *, *, #55674, .T. ) ;
#31301=EDGE_CURVE ( 'NONE', #50848, #925, #2619, .T. ) ;
#31302=DIRECTION ( 'NONE',  ( -0.8805955318567321166, -0.4738686624730094055, 0.000000000000000000 ) ) ;
#31309=CARTESIAN_POINT ( 'NONE',  ( -6.214074333988410359, 32.84308755423718651, 6.893343212288937316 ) ) ;
#31315=EDGE_CURVE ( 'NONE', #53910, #20254, #30051, .T. ) ;
#31321=EDGE_CURVE ( 'NONE', #43258, #13094, #18105, .T. ) ;
#31341=VERTEX_POINT ( 'NONE', #40942 ) ;
#31356=EDGE_CURVE ( 'NONE', #34646, #65008, #24084, .T. ) ;
#31363=ORIENTED_EDGE ( 'NONE', *, *, #47455, .F. ) ;
#31364=EDGE_CURVE ( 'NONE', #26796, #46943, #50803, .T. ) ;
#31365=EDGE_CURVE ( 'NONE', #19302, #36305, #26719, .T. ) ;
#31366=EDGE_CURVE ( 'NONE', #44661, #4035, #45525, .T. ) ;
#31370=DIRECTION ( 'NONE',  ( -0.000000000000000000, -0.000000000000000000, -1.000000000000000000 ) ) ;
#31378=CARTESIAN_POINT ( 'NONE',  ( -60.41792053122280493, 24.01035990323434177, 3.061616997868437868E-16 ) ) ;
#31384=PLANE ( 'NONE',  #32154 ) ;
#31386=ORIENTED_EDGE ( 'NONE', *, *, #17114, .T. ) ;
#31396=EDGE_CURVE ( 'NONE', #69476, #60419, #24772, .T. ) ;
#31402=CARTESIAN_POINT ( 'NONE',  ( 24.39800339187933176, -60.26242556095669300, 170.0000000000000000 ) ) ;
#31406=ORIENTED_EDGE ( 'NONE', *, *, #53653, .F. ) ;
#31414=CARTESIAN_POINT ( 'NONE',  ( 29.86848256228521237, 58.14280299503737837, 41.38025477438755928 ) ) ;
#31426=AXIS2_PLACEMENT_3D ( 'NONE', #2754, #50589, #66097 ) ;
#31439=CARTESIAN_POINT ( 'NONE',  ( 69.68177367721139603, 20.52767805628179332, 43.58025477438756923 ) ) ;
#31443=VECTOR ( 'NONE', #7119, 1000.000000000000000 ) ;
#31445=LINE ( 'NONE', #21565, #35428 ) ;
#31450=EDGE_CURVE ( 'NONE', #671, #69476, #61574, .T. ) ;
#31455=PLANE ( 'NONE',  #69146 ) ;
#31456=ORIENTED_EDGE ( 'NONE', *, *, #41613, .T. ) ;
#31463=DIRECTION ( 'NONE',  ( 0.000000000000000000, 0.000000000000000000, 1.000000000000000000 ) ) ;
#31478=EDGE_CURVE ( 'NONE', #30275, #61402, #9633, .T. ) ;
#31510=EDGE_CURVE ( 'NONE', #26272, #13054, #27080, .T. ) ;
#31514=EDGE_CURVE ( 'NONE', #47483, #32488, #6532, .T. ) ;
#31520=EDGE_LOOP ( 'NONE', ( #55569, #47425, #42525, #59911 ) ) ;
#31521=CARTESIAN_POINT ( 'NONE',  ( 63.74253542338309586, -39.54050679744447194, 170.0000000000000000 ) ) ;
#31522=FACE_OUTER_BOUND ( 'NONE', #18913, .T. ) ;
#31544=LINE ( 'NONE', #69506, #60595 ) ;
#31545=CARTESIAN_POINT ( 'NONE',  ( 0.000000000000000000, 0.000000000000000000, 41.38025477438755928 ) ) ;
#31552=PLANE ( 'NONE',  #37808 ) ;
#31560=CARTESIAN_POINT ( 'NONE',  ( 70.21761529798065737, -26.35311180609978976, 0.000000000000000000 ) ) ;
#31564=CARTESIAN_POINT ( 'NONE',  ( 45.74764628539832501, -59.37057832282265935, 41.38025477438755928 ) ) ;
#31590=ORIENTED_EDGE ( 'NONE', *, *, #48882, .F. ) ;
#31596=EDGE_CURVE ( 'NONE', #14304, #3292, #7703, .T. ) ;
#31598=ORIENTED_EDGE ( 'NONE', *, *, #37765, .F. ) ;
#31602=EDGE_CURVE ( 'NONE', #50613, #23880, #54142, .T. ) ;
#31603=CARTESIAN_POINT ( 'NONE',  ( 34.41143668122512622, -66.58502636910473882, 41.38025477438755928 ) ) ;
#31604=CIRCLE ( 'NONE', #59643, 24.99999999999985434 ) ;
#31605=CIRCLE ( 'NONE', #51792, 65.00000000000000000 ) ;
#31606=ORIENTED_EDGE ( 'NONE', *, *, #9484, .F. ) ;
#31607=DIRECTION ( 'NONE',  ( -1.000000000000000000, 0.000000000000000000, 0.000000000000000000 ) ) ;
#31613=EDGE_CURVE ( 'NONE', #48432, #18701, #1760, .T. ) ;
#31615=CARTESIAN_POINT ( 'NONE',  ( 0.000000000000000000, 0.000000000000000000, 41.38025477438755928 ) ) ;
#31630=B_SPLINE_CURVE_WITH_KNOTS ( 'NONE', 3,
 ( #52280, #14990, #56518, #51599 ),
 .UNSPECIFIED., .F., .F.,
 ( 4, 4 ),
 ( 9.900409499157970321E-07, 0.05658314289920115397 ),
 .UNSPECIFIED. ) ;
#31633=CARTESIAN_POINT ( 'NONE',  ( -50.88541732109811022, 55.03078243218087806, 41.38025477438755928 ) ) ;
#31634=CARTESIAN_POINT ( 'NONE',  ( 21.98745393275193294, 71.71550996510526943, 170.0000000000000000 ) ) ;
#31636=DIRECTION ( 'NONE',  ( 0.7227948638273878901, 0.6910626489868685329, -0.000000000000000000 ) ) ;
#31638=CARTESIAN_POINT ( 'NONE',  ( 63.69186821587179281, -39.51023455020688857, 41.38025477438755928 ) ) ;
#31640=ORIENTED_EDGE ( 'NONE', *, *, #34000, .F. ) ;
#31642=VERTEX_POINT ( 'NONE', #23563 ) ;
#31648=VECTOR ( 'NONE', #15511, 1000.000000000000114 ) ;
#31652=EDGE_CURVE ( 'NONE', #2785, #68173, #26765, .T. ) ;
#31658=DIRECTION ( 'NONE',  ( 1.000000000000000000, 0.000000000000000000, 0.000000000000000000 ) ) ;
#31663=DIRECTION ( 'NONE',  ( -1.000000000000000000, 0.000000000000000000, 0.000000000000000000 ) ) ;
#31664=DIRECTION ( 'NONE',  ( 0.000000000000000000, 0.000000000000000000, 1.000000000000000000 ) ) ;
#31667=ORIENTED_EDGE ( 'NONE', *, *, #62333, .F. ) ;
#31673=CARTESIAN_POINT ( 'NONE',  ( 69.68177367721197868, -20.52767805628085895, 43.58025477438756923 ) ) ;
#31675=EDGE_CURVE ( 'NONE', #57182, #25430, #33769, .T. ) ;
#31676=DIRECTION ( 'NONE',  ( 0.000000000000000000, 0.000000000000000000, 1.000000000000000000 ) ) ;
#31679=CARTESIAN_POINT ( 'NONE',  ( -60.41792053122248518, -24.01035990323518021, 41.38025477438755928 ) ) ;
#31689=ORIENTED_EDGE ( 'NONE', *, *, #52318, .F. ) ;
#31693=VECTOR ( 'NONE', #57652, 1000.000000000000000 ) ;
#31700=AXIS2_PLACEMENT_3D ( 'NONE', #53055, #20367, #25322 ) ;
#31709=ORIENTED_EDGE ( 'NONE', *, *, #67817, .T. ) ;
#31710=VECTOR ( 'NONE', #38258, 1000.000000000000000 ) ;
#31716=CARTESIAN_POINT ( 'NONE',  ( -74.58602291351368763, 7.967916035251061402, 170.0000000000000000 ) ) ;
#31727=EDGE_LOOP ( 'NONE', ( #37492, #20556, #24407, #9537 ) ) ;
#31735=PLANE ( 'NONE',  #61088 ) ;
#31736=DIRECTION ( 'NONE',  ( 4.974206872490772509E-18, 1.135330258912677140E-18, -1.000000000000000000 ) ) ;
#31737=EDGE_LOOP ( 'NONE', ( #22224, #37337, #34597, #46172 ) ) ;
#31740=CARTESIAN_POINT ( 'NONE',  ( -34.75846525699014933, 54.92585086258208804, 40.00000000000003553 ) ) ;
#31748=DIRECTION ( 'NONE',  ( -0.000000000000000000, 0.000000000000000000, -1.000000000000000000 ) ) ;
#31757=CIRCLE ( 'NONE', #45265, 65.36598343705435354 ) ;
#31767=EDGE_CURVE ( 'NONE', #16525, #67731, #39134, .T. ) ;
#31770=ORIENTED_EDGE ( 'NONE', *, *, #27568, .F. ) ;
#31773=ORIENTED_EDGE ( 'NONE', *, *, #55506, .F. ) ;
#31774=ORIENTED_EDGE ( 'NONE', *, *, #62688, .F. ) ;
#31776=DIRECTION ( 'NONE',  ( 0.000000000000000000, 0.000000000000000000, 1.000000000000000000 ) ) ;
#31780=CARTESIAN_POINT ( 'NONE',  ( 0.000000000000000000, 0.000000000000000000, 40.00000000000003553 ) ) ;
#31782=EDGE_CURVE ( 'NONE', #33970, #43782, #29877, .T. ) ;
#31784=EDGE_CURVE ( 'NONE', #11268, #22437, #13327, .T. ) ;
#31795=DIRECTION ( 'NONE',  ( 0.000000000000000000, 0.000000000000000000, -1.000000000000000000 ) ) ;
#31798=CONICAL_SURFACE ( 'NONE', #49758, 65.00000000000000000, 0.7853981633974497223 ) ;
#31809=AXIS2_PLACEMENT_3D ( 'NONE', #59429, #30995, #5618 ) ;
#31818=B_SPLINE_CURVE_WITH_KNOTS ( 'NONE', 3,
 ( #57025, #56671, #29582, #30635 ),
 .UNSPECIFIED., .F., .F.,
 ( 4, 4 ),
 ( 0.1259919275528358640, 0.1829744153748747992 ),
 .UNSPECIFIED. ) ;
#31825=EDGE_CURVE ( 'NONE', #27278, #42385, #57302, .T. ) ;
#31829=FACE_OUTER_BOUND ( 'NONE', #1343, .T. ) ;
#31834=CARTESIAN_POINT ( 'NONE',  ( 9.962235950564874543, 64.23203137738424573, 40.00000000000003553 ) ) ;
#31838=FACE_OUTER_BOUND ( 'NONE', #68113, .T. ) ;
#31846=VECTOR ( 'NONE', #44969, 1000.000000000000000 ) ;
#31847=FACE_OUTER_BOUND ( 'NONE', #1585, .T. ) ;
#31861=VECTOR ( 'NONE', #6686, 1000.000000000000114 ) ;
#31866=DIRECTION ( 'NONE',  ( -1.000000000000000000, 0.000000000000000000, 0.000000000000000000 ) ) ;
#31884=ORIENTED_EDGE ( 'NONE', *, *, #20976, .F. ) ;
#31888=CARTESIAN_POINT ( 'NONE',  ( -23.70047331481904607, -76.98764151615553430, 73.58025477438756923 ) ) ;
#31892=CARTESIAN_POINT ( 'NONE',  ( -10.00000000000000000, 0.000000000000000000, 2.000000000000001776 ) ) ;
#31899=LINE ( 'NONE', #53331, #17170 ) ;
#31912=VERTEX_POINT ( 'NONE', #15425 ) ;
#31919=LINE ( 'NONE', #4491, #43320 ) ;
#31923=DIRECTION ( 'NONE',  ( 0.04486483035051862939, -0.9989930665413143673, 0.000000000000000000 ) ) ;
#31924=ORIENTED_EDGE ( 'NONE', *, *, #24972, .F. ) ;
#31936=EDGE_CURVE ( 'NONE', #35650, #64382, #21381, .T. ) ;
#31943=ORIENTED_EDGE ( 'NONE', *, *, #28827, .T. ) ;
#31955=AXIS2_PLACEMENT_3D ( 'NONE', #15497, #31664, #10890 ) ;
#31959=VECTOR ( 'NONE', #7712, 1000.000000000000000 ) ;
#31963=CIRCLE ( 'NONE', #63401, 65.00000000000000000 ) ;
#31968=CARTESIAN_POINT ( 'NONE',  ( 10.00000000000000000, 1.224646799147353256E-15, 0.000000000000000000 ) ) ;
#31977=ORIENTED_EDGE ( 'NONE', *, *, #15817, .T. ) ;
#31982=DIRECTION ( 'NONE',  ( 0.000000000000000000, 0.000000000000000000, 1.000000000000000000 ) ) ;
#31987=EDGE_CURVE ( 'NONE', #42819, #67708, #67263, .T. ) ;
#31990=CIRCLE ( 'NONE', #29737, 65.36598343705435354 ) ;
#31997=AXIS2_PLACEMENT_3D ( 'NONE', #9641, #31101, #30064 ) ;
#32010=ORIENTED_EDGE ( 'NONE', *, *, #16376, .F. ) ;
#32014=CARTESIAN_POINT ( 'NONE',  ( -59.09450113343203270, -27.07101652673575032, 40.00000000000003553 ) ) ;
#32015=DIRECTION ( 'NONE',  ( 0.3930250316539278255, -0.9195277725514487965, 0.000000000000000000 ) ) ;
#32018=EDGE_CURVE ( 'NONE', #57123, #50465, #7750, .T. ) ;
#32020=VERTEX_POINT ( 'NONE', #2031 ) ;
#32022=ORIENTED_EDGE ( 'NONE', *, *, #10769, .T. ) ;
#32030=PLANE ( 'NONE',  #53601 ) ;
#32036=ORIENTED_EDGE ( 'NONE', *, *, #40407, .T. ) ;
#32038=ORIENTED_EDGE ( 'NONE', *, *, #9996, .T. ) ;
#32042=ORIENTED_EDGE ( 'NONE', *, *, #56706, .T. ) ;
#32047=ORIENTED_EDGE ( 'NONE', *, *, #45610, .T. ) ;
#32053=AXIS2_PLACEMENT_3D ( 'NONE', #8639, #47281, #35363 ) ;
#32055=CARTESIAN_POINT ( 'NONE',  ( 19.00668540189274225, -62.54164772954691642, 6.377659838150142862E-18 ) ) ;
#32056=CARTESIAN_POINT ( 'NONE',  ( 0.000000000000000000, 0.000000000000000000, 0.000000000000000000 ) ) ;
#32061=LINE ( 'NONE', #58775, #47747 ) ;
#32077=ORIENTED_EDGE ( 'NONE', *, *, #7394, .T. ) ;
#32081=ADVANCED_FACE ( 'NONE', ( #44215 ), #33343, .T. ) ;
#32086=DIRECTION ( 'NONE',  ( 1.000000000000000000, 0.000000000000000000, -0.000000000000000000 ) ) ;
#32088=ORIENTED_EDGE ( 'NONE', *, *, #33549, .T. ) ;
#32092=LINE ( 'NONE', #42971, #52133 ) ;
#32093=B_SPLINE_CURVE_WITH_KNOTS ( 'NONE', 3,
 ( #66951, #45123, #45470, #24725, #19085, #66268 ),
 .UNSPECIFIED., .F., .F.,
 ( 4, 2, 4 ),
 ( 0.03218933845493725937, 0.06469832000440833841, 0.09720730155387943827 ),
 .UNSPECIFIED. ) ;
#32095=VECTOR ( 'NONE', #1905, 1000.000000000000000 ) ;
#32097=ORIENTED_EDGE ( 'NONE', *, *, #56532, .F. ) ;
#32108=DIRECTION ( 'NONE',  ( -0.000000000000000000, -0.000000000000000000, 1.000000000000000000 ) ) ;
#32120=CARTESIAN_POINT ( 'NONE',  ( 21.38432669263065122, -61.76910524360950916, 41.38025477438755928 ) ) ;
#32121=EDGE_LOOP ( 'NONE', ( #29551, #7205, #40680, #53091 ) ) ;
#32122=VERTEX_POINT ( 'NONE', #28395 ) ;
#32124=DIRECTION ( 'NONE',  ( 0.3930250316539148359, 0.9195277725514544587, -0.000000000000000000 ) ) ;
#32132=EDGE_CURVE ( 'NONE', #1714, #2078, #41438, .T. ) ;
#32135=EDGE_CURVE ( 'NONE', #25958, #308, #68566, .T. ) ;
#32137=CARTESIAN_POINT ( 'NONE',  ( 12.99074365121454910, -21.50298515537749822, 3.061616997868437868E-16 ) ) ;
#32143=ORIENTED_EDGE ( 'NONE', *, *, #25273, .T. ) ;
#32146=VECTOR ( 'NONE', #38083, 1000.000000000000000 ) ;
#32150=CARTESIAN_POINT ( 'NONE',  ( 38.07387156563210340, -34.92400885808820021, 26.66469104408689006 ) ) ;
#32154=AXIS2_PLACEMENT_3D ( 'NONE', #26102, #27127, #42619 ) ;
#32155=CARTESIAN_POINT ( 'NONE',  ( -37.75148815634407384, 54.92203319703903475, 34.48241823996504252 ) ) ;
#32156=ADVANCED_FACE ( 'NONE', ( #11869 ), #54870, .T. ) ;
#32168=EDGE_CURVE ( 'NONE', #44628, #68305, #8854, .T. ) ;
#32170=B_SPLINE_CURVE_WITH_KNOTS ( 'NONE', 3,
 ( #52644, #64591, #58954, #25927 ),
 .UNSPECIFIED., .F., .F.,
 ( 4, 4 ),
 ( 9.900409499142632672E-07, 0.05658314289920113316 ),
 .UNSPECIFIED. ) ;
#32173=DIRECTION ( 'NONE',  ( -0.04486483035051862939, 0.9989930665413143673, 0.000000000000000000 ) ) ;
#32180=CARTESIAN_POINT ( 'NONE',  ( -2.116120943112233643, 74.98056102853672655, 170.0000000000000000 ) ) ;
#32183=EDGE_CURVE ( 'NONE', #17738, #62756, #46629, .T. ) ;
#32186=LINE ( 'NONE', #5442, #8708 ) ;
#32205=VECTOR ( 'NONE', #44837, 1000.000000000000114 ) ;
#32213=ORIENTED_EDGE ( 'NONE', *, *, #37854, .F. ) ;
#32215=CARTESIAN_POINT ( 'NONE',  ( 0.000000000000000000, 0.000000000000000000, 40.00000000000003553 ) ) ;
#32221=VERTEX_POINT ( 'NONE', #26583 ) ;
#32228=CARTESIAN_POINT ( 'NONE',  ( 0.000000000000000000, 0.000000000000000000, 41.38025477438755928 ) ) ;
#32245=EDGE_CURVE ( 'NONE', #68939, #4283, #20091, .T. ) ;
#32248=LINE ( 'NONE', #21331, #61028 ) ;
#32251=VECTOR ( 'NONE', #44848, 1000.000000000000000 ) ;
#32252=FACE_OUTER_BOUND ( 'NONE', #52609, .T. ) ;
#32260=ORIENTED_EDGE ( 'NONE', *, *, #67454, .T. ) ;
#32269=ADVANCED_FACE ( 'NONE', ( #5119 ), #64914, .T. ) ;
#32275=DIRECTION ( 'NONE',  ( -0.000000000000000000, -0.000000000000000000, -1.000000000000000000 ) ) ;
#32280=DIRECTION ( 'NONE',  ( -1.000000000000000000, 0.000000000000000000, 0.000000000000000000 ) ) ;
#32304=ORIENTED_EDGE ( 'NONE', *, *, #26202, .F. ) ;
#32310=EDGE_CURVE ( 'NONE', #48012, #42925, #33257, .T. ) ;
#32312=DIRECTION ( 'NONE',  ( 1.000000000000000000, 0.000000000000000000, 0.000000000000000000 ) ) ;
#32316=DIRECTION ( 'NONE',  ( -0.000000000000000000, -0.000000000000000000, -1.000000000000000000 ) ) ;
#32331=CARTESIAN_POINT ( 'NONE',  ( -65.36598343705435354, 0.000000000000000000, 41.38025477438755928 ) ) ;
#32336=CARTESIAN_POINT ( 'NONE',  ( 0.000000000000000000, 0.000000000000000000, 41.38025477438755928 ) ) ;
#32340=FACE_OUTER_BOUND ( 'NONE', #28153, .T. ) ;
#32342=CARTESIAN_POINT ( 'NONE',  ( -84.49322488516129681, 0.000000000000000000, 43.58025477438756212 ) ) ;
#32356=EDGE_CURVE ( 'NONE', #35709, #58120, #42526, .T. ) ;
#32361=VECTOR ( 'NONE', #28540, 1000.000000000000000 ) ;
#32364=EDGE_LOOP ( 'NONE', ( #39753, #17011, #47505, #59219 ) ) ;
#32371=CARTESIAN_POINT ( 'NONE',  ( -24.87827947785784133, 3.494138152041632583, 0.000000000000000000 ) ) ;
#32373=LINE ( 'NONE', #27078, #56260 ) ;
#32383=EDGE_CURVE ( 'NONE', #28214, #22131, #23472, .T. ) ;
#32384=ORIENTED_EDGE ( 'NONE', *, *, #55773, .F. ) ;
#32385=EDGE_CURVE ( 'NONE', #16778, #24416, #1237, .T. ) ;
#32388=EDGE_CURVE ( 'NONE', #67298, #9035, #29093, .T. ) ;
#32390=VECTOR ( 'NONE', #19051, 1000.000000000000114 ) ;
#32399=ORIENTED_EDGE ( 'NONE', *, *, #16820, .F. ) ;
#32404=CARTESIAN_POINT ( 'NONE',  ( 0.000000000000000000, 0.000000000000000000, 170.0000000000000000 ) ) ;
#32414=CARTESIAN_POINT ( 'NONE',  ( 50.03867889673374236, -42.05760816978110483, 3.125053320693570611E-16 ) ) ;
#32437=ORIENTED_EDGE ( 'NONE', *, *, #10456, .F. ) ;
#32440=DIRECTION ( 'NONE',  ( 0.000000000000000000, 0.000000000000000000, -1.000000000000000000 ) ) ;
#32441=AXIS2_PLACEMENT_3D ( 'NONE', #53293, #52615, #4440 ) ;
#32447=FACE_OUTER_BOUND ( 'NONE', #65889, .T. ) ;
#32463=EDGE_CURVE ( 'NONE', #57236, #38237, #26814, .T. ) ;
#32470=ORIENTED_EDGE ( 'NONE', *, *, #7255, .T. ) ;
#32477=VERTEX_POINT ( 'NONE', #8256 ) ;
#32479=DIRECTION ( 'NONE',  ( 2.312964634635743450E-16, -0.000000000000000000, 1.000000000000000000 ) ) ;
#32486=CARTESIAN_POINT ( 'NONE',  ( -24.53636015449704644, -60.58612729876431047, 3.125053320693577513E-16 ) ) ;
#32488=VERTEX_POINT ( 'NONE', #61710 ) ;
#32494=CARTESIAN_POINT ( 'NONE',  ( 0.000000000000000000, 0.000000000000000000, 41.38025477438755928 ) ) ;
#32501=ORIENTED_EDGE ( 'NONE', *, *, #10997, .F. ) ;
#32502=ORIENTED_EDGE ( 'NONE', *, *, #2252, .F. ) ;
#32504=DIRECTION ( 'NONE',  ( -0.000000000000000000, 0.000000000000000000, -1.000000000000000000 ) ) ;
#32511=VERTEX_POINT ( 'NONE', #3662 ) ;
#32512=EDGE_LOOP ( 'NONE', ( #22601, #30247, #43036, #42455 ) ) ;
#32514=CARTESIAN_POINT ( 'NONE',  ( 0.000000000000000000, 0.000000000000000000, 0.000000000000000000 ) ) ;
#32517=VECTOR ( 'NONE', #21418, 1000.000000000000000 ) ;
#32528=CYLINDRICAL_SURFACE ( 'NONE', #56662, 65.36598343705435354 ) ;
#32529=FACE_OUTER_BOUND ( 'NONE', #29690, .T. ) ;
#32532=DIRECTION ( 'NONE',  ( -0.000000000000000000, -0.000000000000000000, -1.000000000000000000 ) ) ;
#32537=AXIS2_PLACEMENT_3D ( 'NONE', #61459, #11874, #2037 ) ;
#32541=ADVANCED_FACE ( 'NONE', ( #18119 ), #67356, .T. ) ;
#32547=PLANE ( 'NONE',  #48749 ) ;
#32555=VECTOR ( 'NONE', #52733, 1000.000000000000000 ) ;
#32564=PLANE ( 'NONE',  #19036 ) ;
#32569=ORIENTED_EDGE ( 'NONE', *, *, #59368, .F. ) ;
#32571=AXIS2_PLACEMENT_3D ( 'NONE', #23701, #18418, #49362 ) ;
#32573=EDGE_CURVE ( 'NONE', #26680, #65664, #62595, .T. ) ;
#32577=CARTESIAN_POINT ( 'NONE',  ( -44.26023579658939866, 48.10138582123772721, 43.58025477438756212 ) ) ;
#32593=CARTESIAN_POINT ( 'NONE',  ( 5.722401031430903728, 32.93231310368437903, 6.893343212288939093 ) ) ;
#32609=CARTESIAN_POINT ( 'NONE',  ( -18.24318075359455804, -17.27206262134411574, 0.000000000000000000 ) ) ;
#32610=DIRECTION ( 'NONE',  ( 0.6234898018587318180, 0.7818314824680311359, 0.000000000000000000 ) ) ;
#32621=ORIENTED_EDGE ( 'NONE', *, *, #64468, .F. ) ;
#32623=CIRCLE ( 'NONE', #34900, 74.95140232871122521 ) ;
#32629=ORIENTED_EDGE ( 'NONE', *, *, #67944, .F. ) ;
#32630=LINE ( 'NONE', #53372, #40276 ) ;
#32636=EDGE_CURVE ( 'NONE', #18983, #22088, #20140, .T. ) ;
#32641=ORIENTED_EDGE ( 'NONE', *, *, #27390, .T. ) ;
#32644=ORIENTED_EDGE ( 'NONE', *, *, #26747, .T. ) ;
#32650=VECTOR ( 'NONE', #60632, 1000.000000000000114 ) ;
#32654=CARTESIAN_POINT ( 'NONE',  ( -62.31345272479909880, 18.49415068377641447, 40.00000000000003553 ) ) ;
#32670=CARTESIAN_POINT ( 'NONE',  ( -64.61430802170484355, -7.070445451048284369, 170.0000000000000000 ) ) ;
#32673=DIRECTION ( 'NONE',  ( 0.3513748240813435175, -0.9362348706397369824, 5.102127870520019688E-18 ) ) ;
#32674=LINE ( 'NONE', #16144, #11448 ) ;
#32675=CARTESIAN_POINT ( 'NONE',  ( 43.10136267511096264, 39.31639556316177675, 27.58472369426656812 ) ) ;
#32676=VERTEX_POINT ( 'NONE', #47589 ) ;
#32679=DIRECTION ( 'NONE',  ( 1.000000000000000000, 0.000000000000000000, -0.000000000000000000 ) ) ;
#32691=ORIENTED_EDGE ( 'NONE', *, *, #12817, .T. ) ;
#32698=PLANE ( 'NONE',  #46558 ) ;
#32700=ORIENTED_EDGE ( 'NONE', *, *, #61307, .F. ) ;
#32706=CARTESIAN_POINT ( 'NONE',  ( 29.69502258243350923, 57.82046033912877903, 73.58025477438755502 ) ) ;
#32714=CARTESIAN_POINT ( 'NONE',  ( 0.000000000000000000, 0.000000000000000000, 0.000000000000000000 ) ) ;
#32717=DIRECTION ( 'NONE',  ( 1.000000000000000000, -2.220446049250313081E-14, 0.000000000000000000 ) ) ;
#32721=CARTESIAN_POINT ( 'NONE',  ( 24.34685647902980676, 70.88683439560453792, 41.38025477438755928 ) ) ;
#32734=CARTESIAN_POINT ( 'NONE',  ( 3.904274462092029996, 38.13465922106460226, 13.32819299319724138 ) ) ;
#32736=ORIENTED_EDGE ( 'NONE', *, *, #50252, .T. ) ;
#32738=CARTESIAN_POINT ( 'NONE',  ( -65.36598343705435354, 0.000000000000000000, 41.38025477438755928 ) ) ;
#32739=DIRECTION ( 'NONE',  ( -0.9009688679024218105, 0.4338837391175525693, 0.000000000000000000 ) ) ;
#32743=CARTESIAN_POINT ( 'NONE',  ( 70.60157554497493493, -25.16207943727098950, 41.38025477438755928 ) ) ;
#32749=VECTOR ( 'NONE', #60229, 999.9999999999998863 ) ;
#32752=CARTESIAN_POINT ( 'NONE',  ( -1.683356153842356262, -65.34430428700412108, 41.38025477438755928 ) ) ;
#32755=LINE ( 'NONE', #16572, #25845 ) ;
#32760=DIRECTION ( 'NONE',  ( 1.000000000000000000, 0.000000000000000000, 0.000000000000000000 ) ) ;
#32764=ORIENTED_EDGE ( 'NONE', *, *, #15715, .T. ) ;
#32770=CARTESIAN_POINT ( 'NONE',  ( 26.12852347772543737, 70.00000000000000000, 77.58025477438755502 ) ) ;
#32771=CARTESIAN_POINT ( 'NONE',  ( -9.964117946889912147, 64.24592483216710548, 170.0000000000000000 ) ) ;
#32772=AXIS2_PLACEMENT_3D ( 'NONE', #4236, #19716, #25700 ) ;
#32779=VERTEX_POINT ( 'NONE', #14902 ) ;
#32783=EDGE_CURVE ( 'NONE', #37085, #19763, #37388, .T. ) ;
#32785=DIRECTION ( 'NONE',  ( -0.000000000000000000, -0.000000000000000000, -1.000000000000000000 ) ) ;
#32789=PLANE ( 'NONE',  #1223 ) ;
#32802=AXIS2_PLACEMENT_3D ( 'NONE', #60840, #65789, #49576 ) ;
#32805=CARTESIAN_POINT ( 'NONE',  ( -21.95369412746239846, -11.95973721106846455, 0.000000000000000000 ) ) ;
#32813=DIRECTION ( 'NONE',  ( -0.000000000000000000, -0.000000000000000000, 1.000000000000000000 ) ) ;
#32828=DIRECTION ( 'NONE',  ( -0.9639628606958550172, 0.2660368455666687892, 0.000000000000000000 ) ) ;
#32837=DIRECTION ( 'NONE',  ( -0.000000000000000000, -0.000000000000000000, -1.000000000000000000 ) ) ;
#32842=ORIENTED_EDGE ( 'NONE', *, *, #26599, .T. ) ;
#32843=DIRECTION ( 'NONE',  ( 0.9749279121818259508, -0.2225209339563042066, 2.500042656554809847E-16 ) ) ;
#32844=VERTEX_POINT ( 'NONE', #59528 ) ;
#32860=CONICAL_SURFACE ( 'NONE', #53034, 65.00000000000000000, 0.7853981633974497223 ) ;
#32861=CARTESIAN_POINT ( 'NONE',  ( 53.32245423372560111, 37.19594572654715137, 170.0000000000000000 ) ) ;
#32863=EDGE_CURVE ( 'NONE', #8346, #51470, #13451, .T. ) ;
#32886=DIRECTION ( 'NONE',  ( 0.6234898018587318180, 0.7818314824680311359, 0.000000000000000000 ) ) ;
#32888=EDGE_LOOP ( 'NONE', ( #54365, #38536, #3148, #4262 ) ) ;
#32904=EDGE_LOOP ( 'NONE', ( #31123, #9207, #40171, #54989, #12893, #15963, #28134, #58169, #24724 ) ) ;
#32917=CARTESIAN_POINT ( 'NONE',  ( 0.000000000000000000, 0.000000000000000000, 0.000000000000000000 ) ) ;
#32918=DIRECTION ( 'NONE',  ( -1.000000000000000000, 0.000000000000000000, 0.000000000000000000 ) ) ;
#32925=ORIENTED_EDGE ( 'NONE', *, *, #10165, .T. ) ;
#32932=DIRECTION ( 'NONE',  ( 0.000000000000000000, 0.000000000000000000, 1.000000000000000000 ) ) ;
#32946=CARTESIAN_POINT ( 'NONE',  ( -25.87147652227456263, 100.0000000000000000, 129.5802547743875550 ) ) ;
#32962=AXIS2_PLACEMENT_3D ( 'NONE', #36179, #57639, #41112 ) ;
#32976=CARTESIAN_POINT ( 'NONE',  ( -21.44923284420521625, -47.00251590192956286, 26.66469104408689006 ) ) ;
#32987=ORIENTED_EDGE ( 'NONE', *, *, #26149, .T. ) ;
#32990=VERTEX_POINT ( 'NONE', #39370 ) ;
#32998=DIRECTION ( 'NONE',  ( -0.9989930665413144784, -0.04486483035051863633, 2.500042656554809847E-16 ) ) ;
#33000=VECTOR ( 'NONE', #57366, 1000.000000000000000 ) ;
#33009=CIRCLE ( 'NONE', #21802, 65.00000000000000000 ) ;
#33011=ORIENTED_EDGE ( 'NONE', *, *, #25744, .F. ) ;
#33016=DIRECTION ( 'NONE',  ( -1.000000000000000000, 0.000000000000000000, 0.000000000000000000 ) ) ;
#33035=EDGE_CURVE ( 'NONE', #41523, #43949, #23923, .T. ) ;
#33037=DIRECTION ( 'NONE',  ( -1.000000000000000000, 0.000000000000000000, 0.000000000000000000 ) ) ;
#33038=VERTEX_POINT ( 'NONE', #45375 ) ;
#33044=EDGE_LOOP ( 'NONE', ( #56135, #55933, #27293, #488, #50805, #50628, #30712, #37175, #45505 ) ) ;
#33047=DIRECTION ( 'NONE',  ( 0.000000000000000000, 0.000000000000000000, 1.000000000000000000 ) ) ;
#33052=ORIENTED_EDGE ( 'NONE', *, *, #65129, .F. ) ;
#33057=EDGE_CURVE ( 'NONE', #26875, #10843, #25917, .T. ) ;
#33070=ORIENTED_EDGE ( 'NONE', *, *, #69568, .T. ) ;
#33071=EDGE_LOOP ( 'NONE', ( #40800, #12718, #17154, #40366, #61054, #60187, #47581, #50760, #5984 ) ) ;
#33072=DIRECTION ( 'NONE',  ( 0.6234898018587319291, 0.7818314824680311359, 0.000000000000000000 ) ) ;
#33074=DIRECTION ( 'NONE',  ( -0.000000000000000000, -0.000000000000000000, -1.000000000000000000 ) ) ;
#33079=ORIENTED_EDGE ( 'NONE', *, *, #16439, .F. ) ;
#33081=ORIENTED_EDGE ( 'NONE', *, *, #30143, .T. ) ;
#33089=DIRECTION ( 'NONE',  ( 1.000000000000000000, 0.000000000000000000, 0.000000000000000000 ) ) ;
#33092=AXIS2_PLACEMENT_3D ( 'NONE', #61737, #35018, #55419 ) ;
#33100=DIRECTION ( 'NONE',  ( 1.000000000000000000, 0.000000000000000000, 0.000000000000000000 ) ) ;
#33101=ORIENTED_EDGE ( 'NONE', *, *, #61939, .T. ) ;
#33107=CARTESIAN_POINT ( 'NONE',  ( 23.81581464765719502, -7.603089679099516829, 0.000000000000000000 ) ) ;
#33111=EDGE_CURVE ( 'NONE', #1423, #25478, #9389, .T. ) ;
#33114=AXIS2_PLACEMENT_3D ( 'NONE', #25572, #56889, #56525 ) ;
#33115=CARTESIAN_POINT ( 'NONE',  ( 41.71033659965589635, -1.250000000000021982, 13.79046340968178619 ) ) ;
#33117=ADVANCED_FACE ( 'NONE', ( #35163 ), #20620, .T. ) ;
#33119=ORIENTED_EDGE ( 'NONE', *, *, #46593, .F. ) ;
#33124=EDGE_CURVE ( 'NONE', #14014, #16854, #8087, .T. ) ;
#33136=CARTESIAN_POINT ( 'NONE',  ( -8.651394114442540584, -32.28678521934651258, 6.893343212288941757 ) ) ;
#33137=CARTESIAN_POINT ( 'NONE',  ( -66.97713359923307053, -33.64188291209072190, 41.38025477438755928 ) ) ;
#33141=VERTEX_POINT ( 'NONE', #56623 ) ;
#33150=EDGE_CURVE ( 'NONE', #56752, #43605, #40374, .T. ) ;
#33159=FACE_OUTER_BOUND ( 'NONE', #12894, .T. ) ;
#33162=AXIS2_PLACEMENT_3D ( 'NONE', #46291, #57893, #67769 ) ;
#33166=VERTEX_POINT ( 'NONE', #58257 ) ;
#33168=VECTOR ( 'NONE', #33544, 1000.000000000000227 ) ;
#33172=VERTEX_POINT ( 'NONE', #25581 ) ;
#33173=ORIENTED_EDGE ( 'NONE', *, *, #56278, .T. ) ;
#33179=CARTESIAN_POINT ( 'NONE',  ( 64.08056813503694116, 12.89932471814516290, 3.125053320693556313E-16 ) ) ;
#33181=LINE ( 'NONE', #17335, #59244 ) ;
#33182=EDGE_CURVE ( 'NONE', #24540, #14371, #4793, .T. ) ;
#33184=CARTESIAN_POINT ( 'NONE',  ( -41.31727360890708667, -62.59299402909810084, 0.000000000000000000 ) ) ;
#33199=DIRECTION ( 'NONE',  ( -0.000000000000000000, -0.000000000000000000, -1.000000000000000000 ) ) ;
#33201=ORIENTED_EDGE ( 'NONE', *, *, #42084, .F. ) ;
#33202=CIRCLE ( 'NONE', #25384, 74.95140232871122521 ) ;
#33208=CARTESIAN_POINT ( 'NONE',  ( -62.97854483871554976, -16.08424353203763957, 40.00000000000003553 ) ) ;
#33236=LINE ( 'NONE', #27240, #62330 ) ;
#33239=EDGE_CURVE ( 'NONE', #14014, #45637, #48714, .T. ) ;
#33240=CARTESIAN_POINT ( 'NONE',  ( 0.000000000000000000, 0.000000000000000000, 170.0000000000000000 ) ) ;
#33243=VERTEX_POINT ( 'NONE', #48363 ) ;
#33246=DIRECTION ( 'NONE',  ( -1.000000000000000000, 0.000000000000000000, 0.000000000000000000 ) ) ;
#33247=LINE ( 'NONE', #43425, #4282 ) ;
#33252=DIRECTION ( 'NONE',  ( -0.9195277725514544587, 0.3930250316539148359, 5.102127870520019688E-18 ) ) ;
#33257=LINE ( 'NONE', #21991, #22346 ) ;
#33265=DIRECTION ( 'NONE',  ( -2.312964634635743450E-16, 0.000000000000000000, -1.000000000000000000 ) ) ;
#33279=ORIENTED_EDGE ( 'NONE', *, *, #49191, .T. ) ;
#33281=ADVANCED_FACE ( 'NONE', ( #11101 ), #32564, .T. ) ;
#33284=CARTESIAN_POINT ( 'NONE',  ( 60.74750367560238828, -24.13405452624855130, 43.58025477438756212 ) ) ;
#33285=PLANE ( 'NONE',  #45604 ) ;
#33288=DIRECTION ( 'NONE',  ( 0.6234898018587318180, 0.7818314824680311359, -0.000000000000000000 ) ) ;
#33292=ORIENTED_EDGE ( 'NONE', *, *, #22308, .T. ) ;
#33308=ORIENTED_EDGE ( 'NONE', *, *, #29254, .F. ) ;
#33309=AXIS2_PLACEMENT_3D ( 'NONE', #32771, #16241, #16928 ) ;
#33317=DIRECTION ( 'NONE',  ( -0.9989930665413144784, -0.04486483035051863633, 2.500042656554809847E-16 ) ) ;
#33318=AXIS2_PLACEMENT_3D ( 'NONE', #17029, #39552, #38499 ) ;
#33320=DIRECTION ( 'NONE',  ( -0.5508969814521065267, 0.8345732537212999791, 0.000000000000000000 ) ) ;
#33325=DIRECTION ( 'NONE',  ( -1.000000000000000000, 0.000000000000000000, 0.000000000000000000 ) ) ;
#33327=CARTESIAN_POINT ( 'NONE',  ( -23.03840347525633447, -9.707315041312391202, 0.000000000000000000 ) ) ;
#33331=ORIENTED_EDGE ( 'NONE', *, *, #2380, .F. ) ;
#33343=PLANE ( 'NONE',  #15576 ) ;
#33347=B_SPLINE_CURVE_WITH_KNOTS ( 'NONE', 3,
 ( #11566, #47911, #54478, #28461 ),
 .UNSPECIFIED., .F., .F.,
 ( 4, 4 ),
 ( 0.1259919275528358640, 0.1829744153748747437 ),
 .UNSPECIFIED. ) ;
#33352=CARTESIAN_POINT ( 'NONE',  ( -10.96274578891778084, 22.46815979931508167, 0.000000000000000000 ) ) ;
#33354=ORIENTED_EDGE ( 'NONE', *, *, #20149, .T. ) ;
#33356=AXIS2_PLACEMENT_3D ( 'NONE', #45056, #29574, #17993 ) ;
#33363=DIRECTION ( 'NONE',  ( 0.6234898018587431423, -0.7818314824680220321, 0.000000000000000000 ) ) ;
#33369=AXIS2_PLACEMENT_3D ( 'NONE', #63669, #54108, #5934 ) ;
#33370=DIRECTION ( 'NONE',  ( 1.000000000000000000, 0.000000000000000000, 0.000000000000000000 ) ) ;
#33374=CARTESIAN_POINT ( 'NONE',  ( 0.000000000000000000, 0.000000000000000000, 0.000000000000000000 ) ) ;
#33380=ORIENTED_EDGE ( 'NONE', *, *, #57132, .T. ) ;
#33389=ORIENTED_EDGE ( 'NONE', *, *, #37546, .F. ) ;
#33400=CIRCLE ( 'NONE', #26663, 24.99999999999985434 ) ;
#33415=DIRECTION ( 'NONE',  ( -0.3930250316539148359, -0.9195277725514544587, 0.000000000000000000 ) ) ;
#33416=EDGE_LOOP ( 'NONE', ( #50860, #68782, #16368, #28426 ) ) ;
#33418=CARTESIAN_POINT ( 'NONE',  ( -68.06184294702700299, -31.38946074233465211, 41.38025477438755928 ) ) ;
#33423=CARTESIAN_POINT ( 'NONE',  ( 61.62594073580572740, -21.79346734964916266, 41.38025477438755928 ) ) ;
#33424=EDGE_CURVE ( 'NONE', #44801, #24394, #52552, .T. ) ;
#33426=ORIENTED_EDGE ( 'NONE', *, *, #53257, .T. ) ;
#33429=ORIENTED_EDGE ( 'NONE', *, *, #64103, .T. ) ;
#33434=CARTESIAN_POINT ( 'NONE',  ( -13.24252603915608617, 63.63674649211943546, 170.0000000000000000 ) ) ;
#33438=ORIENTED_EDGE ( 'NONE', *, *, #63141, .F. ) ;
#33455=FACE_OUTER_BOUND ( 'NONE', #24898, .T. ) ;
#33458=EDGE_CURVE ( 'NONE', #7475, #28498, #50524, .T. ) ;
#33461=VECTOR ( 'NONE', #66656, 1000.000000000000227 ) ;
#33464=ADVANCED_FACE ( 'NONE', ( #5051 ), #38451, .T. ) ;
#33479=VERTEX_POINT ( 'NONE', #32137 ) ;
#33490=LINE ( 'NONE', #34183, #55462 ) ;
#33491=ORIENTED_EDGE ( 'NONE', *, *, #16721, .F. ) ;
#33492=ORIENTED_EDGE ( 'NONE', *, *, #13101, .F. ) ;
#33494=CARTESIAN_POINT ( 'NONE',  ( 26.12852347772543737, 70.00000000000000000, 129.5802547743875550 ) ) ;
#33495=CARTESIAN_POINT ( 'NONE',  ( -61.29635759142615115, 21.66977272663494958, 170.0000000000000000 ) ) ;
#33514=LINE ( 'NONE', #6053, #32749 ) ;
#33521=DIRECTION ( 'NONE',  ( -1.000000000000000000, 0.000000000000000000, 0.000000000000000000 ) ) ;
#33522=ADVANCED_FACE ( 'NONE', ( #37751 ), #64491, .T. ) ;
#33524=ORIENTED_EDGE ( 'NONE', *, *, #39470, .F. ) ;
#33531=VERTEX_POINT ( 'NONE', #47953 ) ;
#33542=CARTESIAN_POINT ( 'NONE',  ( 0.000000000000000000, 0.000000000000000000, 41.38025477438755928 ) ) ;
#33544=DIRECTION ( 'NONE',  ( -0.2225209339563184452, 0.9749279121818226201, 0.000000000000000000 ) ) ;
#33545=DIRECTION ( 'NONE',  ( -0.000000000000000000, -0.000000000000000000, -1.000000000000000000 ) ) ;
#33549=EDGE_CURVE ( 'NONE', #476, #2404, #42626, .T. ) ;
#33550=ORIENTED_EDGE ( 'NONE', *, *, #2246, .T. ) ;
#33557=CARTESIAN_POINT ( 'NONE',  ( -61.36325649057843634, 43.03793052543095854, 41.38025477438755928 ) ) ;
#33564=ORIENTED_EDGE ( 'NONE', *, *, #12225, .F. ) ;
#33571=CARTESIAN_POINT ( 'NONE',  ( 7.533997733929802543, -64.93035244659006366, 41.38025477438755928 ) ) ;
#33576=ORIENTED_EDGE ( 'NONE', *, *, #22711, .T. ) ;
#33577=DIRECTION ( 'NONE',  ( -0.000000000000000000, -0.000000000000000000, -1.000000000000000000 ) ) ;
#33584=DIRECTION ( 'NONE',  ( -1.000000000000000000, 0.000000000000000000, 0.000000000000000000 ) ) ;
#33588=DIRECTION ( 'NONE',  ( -1.000000000000000000, 0.000000000000000000, 0.000000000000000000 ) ) ;
#33589=CARTESIAN_POINT ( 'NONE',  ( 32.06997139192793611, -56.95813133885440038, 43.58025477438756212 ) ) ;
#33591=DIRECTION ( 'NONE',  ( -1.000000000000000000, 0.000000000000000000, 0.000000000000000000 ) ) ;
#33598=CARTESIAN_POINT ( 'NONE',  ( -18.89790202299208133, 62.20684691518606257, 3.061616997868437868E-16 ) ) ;
#33599=ORIENTED_EDGE ( 'NONE', *, *, #4239, .F. ) ;
#33610=ORIENTED_EDGE ( 'NONE', *, *, #36250, .F. ) ;
#33612=LINE ( 'NONE', #17407, #2026 ) ;
#33629=ORIENTED_EDGE ( 'NONE', *, *, #2977, .T. ) ;
#33634=ADVANCED_FACE ( 'NONE', ( #33880 ), #6786, .T. ) ;
#33654=ORIENTED_EDGE ( 'NONE', *, *, #27685, .T. ) ;
#33657=CARTESIAN_POINT ( 'NONE',  ( -24.53636015449790264, 60.58612729876396941, 41.38025477438755928 ) ) ;
#33665=VECTOR ( 'NONE', #41638, 1000.000000000000000 ) ;
#33675=EDGE_CURVE ( 'NONE', #41480, #46223, #28238, .T. ) ;
#33676=CARTESIAN_POINT ( 'NONE',  ( 56.48035995027075273, 49.34540444547854321, 43.58025477438756212 ) ) ;
#33689=DIRECTION ( 'NONE',  ( 0.5128992774059071280, -0.8584487936018655452, 0.000000000000000000 ) ) ;
#33692=DIRECTION ( 'NONE',  ( -0.000000000000000000, -0.000000000000000000, -1.000000000000000000 ) ) ;
#33693=ORIENTED_EDGE ( 'NONE', *, *, #5184, .T. ) ;
#33698=AXIS2_PLACEMENT_3D ( 'NONE', #22901, #12350, #38032 ) ;
#33704=ORIENTED_EDGE ( 'NONE', *, *, #8735, .F. ) ;
#33710=DIRECTION ( 'NONE',  ( 1.000000000000000000, 0.000000000000000000, 0.000000000000000000 ) ) ;
#33714=CYLINDRICAL_SURFACE ( 'NONE', #24392, 65.00000000000000000 ) ;
#33719=ORIENTED_EDGE ( 'NONE', *, *, #5392, .T. ) ;
#33720=ORIENTED_EDGE ( 'NONE', *, *, #47604, .T. ) ;
#33724=PLANE ( 'NONE',  #59390 ) ;
#33727=DIRECTION ( 'NONE',  ( 0.6579387259397136978, -0.7530714660036099684, 5.102127870520022769E-18 ) ) ;
#33735=ORIENTED_EDGE ( 'NONE', *, *, #60585, .F. ) ;
#33741=LINE ( 'NONE', #6647, #20273 ) ;
#33742=EDGE_CURVE ( 'NONE', #15020, #21961, #25753, .T. ) ;
#33748=FACE_OUTER_BOUND ( 'NONE', #3894, .T. ) ;
#33753=CARTESIAN_POINT ( 'NONE',  ( -36.84489839129265931, -53.54860840895233309, 170.0000000000000000 ) ) ;
#33758=EDGE_CURVE ( 'NONE', #39418, #44574, #11181, .T. ) ;
#33759=VERTEX_POINT ( 'NONE', #14151 ) ;
#33760=CARTESIAN_POINT ( 'NONE',  ( -30.26163486738143860, 23.53144966999699150, 13.32819397642332859 ) ) ;
#33767=ORIENTED_EDGE ( 'NONE', *, *, #18062, .T. ) ;
#33769=LINE ( 'NONE', #23220, #2081 ) ;
#33770=ORIENTED_EDGE ( 'NONE', *, *, #65510, .T. ) ;
#33776=CARTESIAN_POINT ( 'NONE',  ( 0.000000000000000000, 0.000000000000000000, 40.00000000000003553 ) ) ;
#33779=CARTESIAN_POINT ( 'NONE',  ( 65.33961467711179694, 13.12780797910698816, 34.48241823980619358 ) ) ;
#33786=CARTESIAN_POINT ( 'NONE',  ( -1.683356153843273750, 65.34430428700410687, 41.38025477438755928 ) ) ;
#33789=DIRECTION ( 'NONE',  ( 1.000000000000000000, 0.000000000000000000, 0.000000000000000000 ) ) ;
#33798=VERTEX_POINT ( 'NONE', #13799 ) ;
#33815=CARTESIAN_POINT ( 'NONE',  ( -19.56458807131831890, -15.75959024859417390, 3.061616997868437868E-16 ) ) ;
#33818=CARTESIAN_POINT ( 'NONE',  ( -48.12872802574198516, -43.70867239603780519, 0.000000000000000000 ) ) ;
#33820=CONICAL_SURFACE ( 'NONE', #57410, 74.95140232871122521, 0.8777644062502172329 ) ;
#33823=AXIS2_PLACEMENT_3D ( 'NONE', #51844, #3657, #8604 ) ;
#33829=EDGE_CURVE ( 'NONE', #30922, #35779, #25826, .T. ) ;
#33830=DIRECTION ( 'NONE',  ( -1.807017991507219923E-16, 1.727686100818908852E-16, 1.000000000000000000 ) ) ;
#33836=AXIS2_PLACEMENT_3D ( 'NONE', #59122, #64763, #1094 ) ;
#33843=DIRECTION ( 'NONE',  ( 0.9510565162951545304, -0.3090169943749447312, 5.102127870520021228E-18 ) ) ;
#33854=EDGE_CURVE ( 'NONE', #35286, #49653, #41233, .T. ) ;
#33855=DIRECTION ( 'NONE',  ( 0.000000000000000000, 0.000000000000000000, 1.000000000000000000 ) ) ;
#33860=CARTESIAN_POINT ( 'NONE',  ( -24.51966494718108081, 5.470267094204372960, 3.061616997868437868E-16 ) ) ;
#33861=ORIENTED_EDGE ( 'NONE', *, *, #67999, .T. ) ;
#33862=PLANE ( 'NONE',  #22973 ) ;
#33880=FACE_OUTER_BOUND ( 'NONE', #55166, .T. ) ;
#33888=ORIENTED_EDGE ( 'NONE', *, *, #5526, .T. ) ;
#33889=CARTESIAN_POINT ( 'NONE',  ( 0.000000000000000000, 0.000000000000000000, 41.38025477438755928 ) ) ;
#33892=EDGE_CURVE ( 'NONE', #2402, #37212, #4622, .T. ) ;
#33895=CARTESIAN_POINT ( 'NONE',  ( -27.75784411156621090, 18.62216926092103009, 6.893342936425399081 ) ) ;
#33898=ADVANCED_FACE ( 'NONE', ( #53828 ), #47872, .T. ) ;
#33907=DIRECTION ( 'NONE',  ( -0.2225209339563042066, -0.9749279121818259508, 0.000000000000000000 ) ) ;
#33910=EDGE_LOOP ( 'NONE', ( #18586, #36846, #16402, #50042 ) ) ;
#33912=VERTEX_POINT ( 'NONE', #9915 ) ;
#33913=ORIENTED_EDGE ( 'NONE', *, *, #45998, .T. ) ;
#33925=VERTEX_POINT ( 'NONE', #65102 ) ;
#33943=CARTESIAN_POINT ( 'NONE',  ( 0.000000000000000000, 0.000000000000000000, 43.58025477438756212 ) ) ;
#33946=ORIENTED_EDGE ( 'NONE', *, *, #9008, .F. ) ;
#33950=ORIENTED_EDGE ( 'NONE', *, *, #57470, .T. ) ;
#33958=FACE_OUTER_BOUND ( 'NONE', #11421, .T. ) ;
#33967=VERTEX_POINT ( 'NONE', #64056 ) ;
#33970=VERTEX_POINT ( 'NONE', #15867 ) ;
#33976=CONICAL_SURFACE ( 'NONE', #3643, 74.95140232871122521, 0.8777644062502172329 ) ;
#33978=FACE_OUTER_BOUND ( 'NONE', #24443, .T. ) ;
#33985=FACE_OUTER_BOUND ( 'NONE', #28491, .T. ) ;
#33988=CARTESIAN_POINT ( 'NONE',  ( -59.94154301275570873, 45.09516516490385385, 170.0000000000000000 ) ) ;
#33991=CARTESIAN_POINT ( 'NONE',  ( -30.62628708973388569, 68.47330165179126027, 170.0000000000000000 ) ) ;
#33992=LINE ( 'NONE', #38924, #38189 ) ;
#33997=ORIENTED_EDGE ( 'NONE', *, *, #28759, .F. ) ;
#34000=EDGE_CURVE ( 'NONE', #39038, #62258, #15535, .T. ) ;
#34005=CARTESIAN_POINT ( 'NONE',  ( 64.97411640938653932, -37.36411256620218069, 41.38025477438755928 ) ) ;
#34009=CARTESIAN_POINT ( 'NONE',  ( 22.07550062443481664, 11.73338281062075872, 0.000000000000000000 ) ) ;
#34029=ADVANCED_FACE ( 'NONE', ( #48893 ), #60578, .T. ) ;
#34065=ORIENTED_EDGE ( 'NONE', *, *, #8831, .F. ) ;
#34068=DIRECTION ( 'NONE',  ( 0.9989930665413143673, 0.04486483035051862939, 0.000000000000000000 ) ) ;
#34069=DIRECTION ( 'NONE',  ( 0.9909497617679332571, 0.1342332658176667581, 2.500042656554810340E-16 ) ) ;
#34075=DIRECTION ( 'NONE',  ( -1.469488203625031485E-16, 2.022576995815118308E-16, 1.000000000000000000 ) ) ;
#34081=VERTEX_POINT ( 'NONE', #60165 ) ;
#34085=ADVANCED_FACE ( 'NONE', ( #11984, #33455 ), #12335, .T. ) ;
#34086=FACE_OUTER_BOUND ( 'NONE', #55774, .T. ) ;
#34099=LINE ( 'NONE', #50268, #34227 ) ;
#34111=DIRECTION ( 'NONE',  ( -0.000000000000000000, -0.000000000000000000, -1.000000000000000000 ) ) ;
#34117=ORIENTED_EDGE ( 'NONE', *, *, #21529, .F. ) ;
#34123=CIRCLE ( 'NONE', #7146, 24.99999999999985434 ) ;
#34126=DIRECTION ( 'NONE',  ( 1.000000000000000000, 0.000000000000000000, 0.000000000000000000 ) ) ;
#34131=VECTOR ( 'NONE', #51507, 1000.000000000000000 ) ;
#34141=EDGE_CURVE ( 'NONE', #35908, #45811, #14421, .T. ) ;
#34142=DIRECTION ( 'NONE',  ( -0.000000000000000000, -0.000000000000000000, -1.000000000000000000 ) ) ;
#34149=ADVANCED_FACE ( 'NONE', ( #19340 ), #40796, .T. ) ;
#34154=EDGE_LOOP ( 'NONE', ( #61818, #62423, #15451, #58308 ) ) ;
#34174=DIRECTION ( 'NONE',  ( -0.6910626489868685329, 0.7227948638273878901, 0.000000000000000000 ) ) ;
#34183=CARTESIAN_POINT ( 'NONE',  ( -25.87147652227456263, 70.00000000000000000, 129.5802547743875550 ) ) ;
#34195=ORIENTED_EDGE ( 'NONE', *, *, #57690, .F. ) ;
#34199=LINE ( 'NONE', #23639, #18341 ) ;
#34202=ORIENTED_EDGE ( 'NONE', *, *, #13292, .F. ) ;
#34203=CARTESIAN_POINT ( 'NONE',  ( 13.24564585880038514, 63.65041531508843065, 43.58025477438756923 ) ) ;
#34205=LINE ( 'NONE', #61622, #61091 ) ;
#34211=VERTEX_POINT ( 'NONE', #291 ) ;
#34215=LINE ( 'NONE', #1865, #53222 ) ;
#34227=VECTOR ( 'NONE', #28819, 1000.000000000000000 ) ;
#34230=LINE ( 'NONE', #44059, #26421 ) ;
#34231=VECTOR ( 'NONE', #13873, 1000.000000000000114 ) ;
#34240=VERTEX_POINT ( 'NONE', #15456 ) ;
#34247=DIRECTION ( 'NONE',  ( -1.000000000000000000, 0.000000000000000000, 0.000000000000000000 ) ) ;
#34260=DIRECTION ( 'NONE',  ( 0.000000000000000000, 0.000000000000000000, 1.000000000000000000 ) ) ;
#34263=VERTEX_POINT ( 'NONE', #38993 ) ;
#34265=VECTOR ( 'NONE', #37585, 1000.000000000000000 ) ;
#34266=FACE_OUTER_BOUND ( 'NONE', #10510, .T. ) ;
#34267=DIRECTION ( 'NONE',  ( 2.437361367520478414E-16, 5.563118268672117023E-17, 1.000000000000000000 ) ) ;
#34270=VECTOR ( 'NONE', #14140, 1000.000000000000000 ) ;
#34274=LINE ( 'NONE', #56070, #5323 ) ;
#34291=LINE ( 'NONE', #39215, #16327 ) ;
#34292=DIRECTION ( 'NONE',  ( -1.000000000000000000, 0.000000000000000000, 0.000000000000000000 ) ) ;
#34298=ORIENTED_EDGE ( 'NONE', *, *, #62017, .T. ) ;
#34304=CARTESIAN_POINT ( 'NONE',  ( 64.16679220703369424, 10.37413986118183828, 40.00000000000003553 ) ) ;
#34318=CARTESIAN_POINT ( 'NONE',  ( 73.57152302639913444, -14.62167909564502821, 170.0000000000000000 ) ) ;
#34325=AXIS2_PLACEMENT_3D ( 'NONE', #4922, #25015, #20759 ) ;
#34330=DIRECTION ( 'NONE',  ( 1.000000000000000000, 0.000000000000000000, 0.000000000000000000 ) ) ;
#34338=AXIS2_PLACEMENT_3D ( 'NONE', #38100, #53916, #117 ) ;
#34347=EDGE_CURVE ( 'NONE', #16942, #53544, #67132, .T. ) ;
#34349=DIRECTION ( 'NONE',  ( -0.000000000000000000, -0.000000000000000000, -1.000000000000000000 ) ) ;
#34350=CARTESIAN_POINT ( 'NONE',  ( 26.53820713381362140, 51.95411424136508316, 27.58472369392174173 ) ) ;
#34357=DIRECTION ( 'NONE',  ( -0.000000000000000000, 0.000000000000000000, -1.000000000000000000 ) ) ;
#34369=DIRECTION ( 'NONE',  ( 1.000000000000000000, 0.000000000000000000, -0.000000000000000000 ) ) ;
#34371=CARTESIAN_POINT ( 'NONE',  ( 0.000000000000000000, 0.000000000000000000, 170.0000000000000000 ) ) ;
#34374=AXIS2_PLACEMENT_3D ( 'NONE', #21930, #64504, #15628 ) ;
#34383=ORIENTED_EDGE ( 'NONE', *, *, #60993, .F. ) ;
#34392=VECTOR ( 'NONE', #24388, 1000.000000000000000 ) ;
#34393=CARTESIAN_POINT ( 'NONE',  ( 6.526941389886392386, -24.13294503563501436, 0.000000000000000000 ) ) ;
#34397=DIRECTION ( 'NONE',  ( -1.000000000000000000, 0.000000000000000000, 0.000000000000000000 ) ) ;
#34403=EDGE_CURVE ( 'NONE', #28975, #4035, #65091, .T. ) ;
#34415=ORIENTED_EDGE ( 'NONE', *, *, #49796, .F. ) ;
#34418=VECTOR ( 'NONE', #49613, 1000.000000000000227 ) ;
#34423=ORIENTED_EDGE ( 'NONE', *, *, #58455, .F. ) ;
#34424=VERTEX_POINT ( 'NONE', #9058 ) ;
#34429=EDGE_CURVE ( 'NONE', #2074, #28747, #1074, .T. ) ;
#34431=CARTESIAN_POINT ( 'NONE',  ( -29.49715792695969085, 42.41725740634736042, 26.66469066592268788 ) ) ;
#34436=CARTESIAN_POINT ( 'NONE',  ( 18.07314801315404296, -17.44990292519077002, 0.000000000000000000 ) ) ;
#34444=VECTOR ( 'NONE', #22130, 1000.000000000000000 ) ;
#34446=CARTESIAN_POINT ( 'NONE',  ( 20.89850557012432830, 13.94239061780435662, 3.061616997868437868E-16 ) ) ;
#34447=CARTESIAN_POINT ( 'NONE',  ( 19.62566184736079578, 15.48655536434876900, 0.000000000000000000 ) ) ;
#34448=CARTESIAN_POINT ( 'NONE',  ( -21.27554331373000096, 61.43430442924864820, 0.000000000000000000 ) ) ;
#34455=ORIENTED_EDGE ( 'NONE', *, *, #42106, .F. ) ;
#34457=FACE_OUTER_BOUND ( 'NONE', #58753, .T. ) ;
#34460=CARTESIAN_POINT ( 'NONE',  ( 65.33961433650038941, -13.12780791729416840, 34.48241795236666007 ) ) ;
#34467=VERTEX_POINT ( 'NONE', #26611 ) ;
#34475=EDGE_CURVE ( 'NONE', #36282, #52894, #40394, .T. ) ;
#34483=LINE ( 'NONE', #54861, #20603 ) ;
#34489=CARTESIAN_POINT ( 'NONE',  ( 57.16566366493297835, 11.64445456857528782, 27.58472369370708321 ) ) ;
#34491=CONICAL_SURFACE ( 'NONE', #9771, 65.00000000000000000, 0.7853981633974497223 ) ;
#34493=CARTESIAN_POINT ( 'NONE',  ( 0.000000000000000000, 0.000000000000000000, 0.000000000000000000 ) ) ;
#34495=EDGE_CURVE ( 'NONE', #33912, #9782, #43119, .T. ) ;
#34499=EDGE_CURVE ( 'NONE', #23153, #12593, #52306, .T. ) ;
#34502=DIRECTION ( 'NONE',  ( 0.4738686624729966379, 0.8805955318567391110, -1.096041457762183139E-16 ) ) ;
#34504=CARTESIAN_POINT ( 'NONE',  ( -74.75133697335806460, 5.472689625386069068, 41.38025477438755928 ) ) ;
#34520=LINE ( 'NONE', #23263, #64235 ) ;
#34524=AXIS2_PLACEMENT_3D ( 'NONE', #53085, #48151, #15481 ) ;
#34525=B_SPLINE_CURVE_WITH_KNOTS ( 'NONE', 3,
 ( #55958, #28879, #29220, #51373, #50331, #3190 ),
 .UNSPECIFIED., .F., .F.,
 ( 4, 2, 4 ),
 ( 1.095770181082984128E-06, 0.03239442681617709513, 0.06478775786217309818 ),
 .UNSPECIFIED. ) ;
#34527=ORIENTED_EDGE ( 'NONE', *, *, #21419, .F. ) ;
#34532=CARTESIAN_POINT ( 'NONE',  ( -65.36598343705435354, 0.000000000000000000, 41.38025477438755928 ) ) ;
#34537=VECTOR ( 'NONE', #2082, 999.9999999999998863 ) ;
#34557=EDGE_CURVE ( 'NONE', #56752, #2801, #32170, .T. ) ;
#34558=EDGE_CURVE ( 'NONE', #29614, #23236, #47358, .T. ) ;
#34578=EDGE_CURVE ( 'NONE', #62629, #21254, #35932, .T. ) ;
#34588=AXIS2_PLACEMENT_3D ( 'NONE', #21830, #10582, #15868 ) ;
#34589=DIRECTION ( 'NONE',  ( 1.000000000000000000, 0.000000000000000000, 0.000000000000000000 ) ) ;
#34597=ORIENTED_EDGE ( 'NONE', *, *, #31510, .T. ) ;
#34605=CARTESIAN_POINT ( 'NONE',  ( 0.000000000000000000, 0.000000000000000000, 41.38025477438755928 ) ) ;
#34614=DIRECTION ( 'NONE',  ( -1.000000000000000000, 0.000000000000000000, 0.000000000000000000 ) ) ;
#34627=VECTOR ( 'NONE', #10130, 1000.000000000000227 ) ;
#34628=UNCERTAINTY_MEASURE_WITH_UNIT (LENGTH_MEASURE( 1.000000000000000082E-05 ), #27587, 'distance_accuracy_value', 'NONE');
#34646=VERTEX_POINT ( 'NONE', #48728 ) ;
#34652=DIRECTION ( 'NONE',  ( 0.3090169943749582759, -0.9510565162951499785, 0.000000000000000000 ) ) ;
#34654=FACE_OUTER_BOUND ( 'NONE', #67611, .T. ) ;
#34656=VERTEX_POINT ( 'NONE', #66272 ) ;
#34667=DIRECTION ( 'NONE',  ( -0.9749279121818259508, 0.2225209339563041788, 0.000000000000000000 ) ) ;
#34668=VERTEX_POINT ( 'NONE', #36658 ) ;
#34669=VECTOR ( 'NONE', #6594, 1000.000000000000114 ) ;
#34674=DIRECTION ( 'NONE',  ( -0.000000000000000000, -0.000000000000000000, -1.000000000000000000 ) ) ;
#34677=PLANE ( 'NONE',  #21827 ) ;
#34680=DIRECTION ( 'NONE',  ( 0.000000000000000000, 0.000000000000000000, 1.000000000000000000 ) ) ;
#34685=DIRECTION ( 'NONE',  ( -0.9510565162951500895, -0.3090169943749583314, 5.102127870520021999E-18 ) ) ;
#34689=ORIENTED_EDGE ( 'NONE', *, *, #65166, .F. ) ;
#34692=CARTESIAN_POINT ( 'NONE',  ( -21.77424096535250442, 54.12382820593439448, 27.58472315868181468 ) ) ;
#34700=ORIENTED_EDGE ( 'NONE', *, *, #15175, .F. ) ;
#34712=CARTESIAN_POINT ( 'NONE',  ( -4.180838820196604466, 65.23214221112780820, 43.58025477438756212 ) ) ;
#34716=PLANE ( 'NONE',  #14128 ) ;
#34721=ORIENTED_EDGE ( 'NONE', *, *, #37731, .T. ) ;
#34725=DIRECTION ( 'NONE',  ( 0.7530714660036099684, 0.6579387259397138088, -0.000000000000000000 ) ) ;
#34726=AXIS2_PLACEMENT_3D ( 'NONE', #56250, #54849, #8065 ) ;
#34729=CARTESIAN_POINT ( 'NONE',  ( -4.613603609464498767, -74.86839895266049894, 170.0000000000000000 ) ) ;
#34739=EDGE_CURVE ( 'NONE', #46954, #30352, #32755, .T. ) ;
#34743=DIRECTION ( 'NONE',  ( -0.000000000000000000, -0.000000000000000000, 1.000000000000000000 ) ) ;
#34747=VERTEX_POINT ( 'NONE', #58437 ) ;
#34764=VERTEX_POINT ( 'NONE', #21497 ) ;
#34771=DIRECTION ( 'NONE',  ( -0.000000000000000000, -0.000000000000000000, -1.000000000000000000 ) ) ;
#34778=EDGE_CURVE ( 'NONE', #40870, #23153, #27121, .T. ) ;
#34792=FACE_OUTER_BOUND ( 'NONE', #20930, .T. ) ;
#34794=PLANE ( 'NONE',  #61128 ) ;
#34796=EDGE_CURVE ( 'NONE', #65969, #42777, #48911, .T. ) ;
#34797=CARTESIAN_POINT ( 'NONE',  ( 14.59045944429442443, -20.30070179093305427, 0.000000000000000000 ) ) ;
#34805=CIRCLE ( 'NONE', #57290, 65.00000000000000000 ) ;
#34808=EDGE_LOOP ( 'NONE', ( #13074, #37648, #47388, #61345 ) ) ;
#34811=CARTESIAN_POINT ( 'NONE',  ( 61.28323125814100081, 21.66484633135460669, 170.0000000000000000 ) ) ;
#34823=EDGE_CURVE ( 'NONE', #35154, #64522, #15737, .T. ) ;
#34827=ADVANCED_FACE ( 'NONE', ( #15882 ), #58780, .T. ) ;
#34837=DIRECTION ( 'NONE',  ( -0.000000000000000000, -0.000000000000000000, 1.000000000000000000 ) ) ;
#34848=ORIENTED_EDGE ( 'NONE', *, *, #59243, .F. ) ;
#34852=CIRCLE ( 'NONE', #29218, 25.12245591505646303 ) ;
#34862=ORIENTED_EDGE ( 'NONE', *, *, #54121, .T. ) ;
#34869=CYLINDRICAL_SURFACE ( 'NONE', #23393, 65.36598343705435354 ) ;
#34872=LINE ( 'NONE', #28542, #56879 ) ;
#34875=ORIENTED_EDGE ( 'NONE', *, *, #9851, .F. ) ;
#34876=ORIENTED_EDGE ( 'NONE', *, *, #22726, .T. ) ;
#34877=EDGE_CURVE ( 'NONE', #26757, #2801, #22458, .T. ) ;
#34879=DIRECTION ( 'NONE',  ( -0.000000000000000000, 0.000000000000000000, -1.000000000000000000 ) ) ;
#34888=DIRECTION ( 'NONE',  ( -0.3090169943749582759, 0.9510565162951499785, 0.000000000000000000 ) ) ;
#34894=EDGE_LOOP ( 'NONE', ( #50116, #14143, #18917, #61790 ) ) ;
#34895=LINE ( 'NONE', #34203, #62727 ) ;
#34900=AXIS2_PLACEMENT_3D ( 'NONE', #48835, #682, #58129 ) ;
#34905=DIRECTION ( 'NONE',  ( -0.000000000000000000, -0.000000000000000000, -1.000000000000000000 ) ) ;
#34914=ORIENTED_EDGE ( 'NONE', *, *, #2945, .F. ) ;
#34915=LINE ( 'NONE', #40871, #35259 ) ;
#34924=FACE_OUTER_BOUND ( 'NONE', #31727, .T. ) ;
#34928=VERTEX_POINT ( 'NONE', #55961 ) ;
#34937=VECTOR ( 'NONE', #28686, 1000.000000000000000 ) ;
#34941=VERTEX_POINT ( 'NONE', #6719 ) ;
#34942=EDGE_CURVE ( 'NONE', #62736, #16812, #67444, .T. ) ;
#34971=CARTESIAN_POINT ( 'NONE',  ( -24.02131509525290554, -34.12171010297063845, 13.79046340968177908 ) ) ;
#34973=B_SPLINE_CURVE_WITH_KNOTS ( 'NONE', 3,
 ( #12026, #66214, #65494, #44371, #11311, #33137 ),
 .UNSPECIFIED., .F., .F.,
 ( 4, 2, 4 ),
 ( 0.03218938496963297952, 0.06469835385212996393, 0.09720732273462692752 ),
 .UNSPECIFIED. ) ;
#34977=CIRCLE ( 'NONE', #63030, 24.99999999999985434 ) ;
#34980=CARTESIAN_POINT ( 'NONE',  ( -56.44201257846630426, 32.26641783793562723, 43.58025477438756923 ) ) ;
#34983=EDGE_LOOP ( 'NONE', ( #51339, #51678, #23267, #27879 ) ) ;
#34987=VECTOR ( 'NONE', #37351, 999.9999999999998863 ) ;
#34991=CARTESIAN_POINT ( 'NONE',  ( 0.000000000000000000, 0.000000000000000000, 41.38025477438755928 ) ) ;
#34997=PLANE ( 'NONE',  #10685 ) ;
#35009=ADVANCED_FACE ( 'NONE', ( #2151 ), #58404, .T. ) ;
#35018=DIRECTION ( 'NONE',  ( -0.000000000000000000, -0.000000000000000000, -1.000000000000000000 ) ) ;
#35022=VERTEX_POINT ( 'NONE', #12349 ) ;
#35034=EDGE_LOOP ( 'NONE', ( #44784, #31255, #57016, #44090 ) ) ;
#35038=FACE_OUTER_BOUND ( 'NONE', #39589, .T. ) ;
#35050=DIRECTION ( 'NONE',  ( -0.000000000000000000, -0.000000000000000000, -1.000000000000000000 ) ) ;
#35065=VERTEX_POINT ( 'NONE', #24650 ) ;
#35072=CARTESIAN_POINT ( 'NONE',  ( 51.85299110299440173, 39.21848821248450179, 170.0000000000000000 ) ) ;
#35084=ORIENTED_EDGE ( 'NONE', *, *, #26149, .F. ) ;
#35096=VERTEX_POINT ( 'NONE', #30960 ) ;
#35101=CARTESIAN_POINT ( 'NONE',  ( -22.06416059020191867, 12.01293505575286602, 0.000000000000000000 ) ) ;
#35105=VERTEX_POINT ( 'NONE', #8465 ) ;
#35108=DIRECTION ( 'NONE',  ( -1.000000000000000000, 0.000000000000000000, 0.000000000000000000 ) ) ;
#35111=CARTESIAN_POINT ( 'NONE',  ( 0.000000000000000000, 0.000000000000000000, 41.41421356237313489 ) ) ;
#35112=ADVANCED_FACE ( 'NONE', ( #13732 ), #20384, .T. ) ;
#35114=DIRECTION ( 'NONE',  ( 0.000000000000000000, 0.000000000000000000, 1.000000000000000000 ) ) ;
#35129=CARTESIAN_POINT ( 'NONE',  ( 44.01696072966022655, -47.84694004974146253, 170.0000000000000000 ) ) ;
#35133=CARTESIAN_POINT ( 'NONE',  ( 0.000000000000000000, 0.000000000000000000, 0.000000000000000000 ) ) ;
#35134=AXIS2_PLACEMENT_3D ( 'NONE', #47226, #64101, #20496 ) ;
#35146=DIRECTION ( 'NONE',  ( 1.000000000000000000, 0.000000000000000000, 0.000000000000000000 ) ) ;
#35153=DIRECTION ( 'NONE',  ( -0.000000000000000000, -0.000000000000000000, 1.000000000000000000 ) ) ;
#35154=VERTEX_POINT ( 'NONE', #57342 ) ;
#35156=LINE ( 'NONE', #25996, #26053 ) ;
#35158=EDGE_CURVE ( 'NONE', #42059, #6090, #48819, .T. ) ;
#35163=FACE_OUTER_BOUND ( 'NONE', #49742, .T. ) ;
#35164=LINE ( 'NONE', #18645, #45013 ) ;
#35166=AXIS2_PLACEMENT_3D ( 'NONE', #42104, #5505, #64600 ) ;
#35168=DIRECTION ( 'NONE',  ( 0.000000000000000000, 0.000000000000000000, 1.000000000000000000 ) ) ;
#35179=EDGE_CURVE ( 'NONE', #242, #53998, #5918, .T. ) ;
#35183=ORIENTED_EDGE ( 'NONE', *, *, #24861, .T. ) ;
#35194=LINE ( 'NONE', #35547, #39933 ) ;
#35197=VERTEX_POINT ( 'NONE', #1012 ) ;
#35202=LINE ( 'NONE', #67239, #14794 ) ;
#35210=ORIENTED_EDGE ( 'NONE', *, *, #8894, .F. ) ;
#35220=ORIENTED_EDGE ( 'NONE', *, *, #4239, .T. ) ;
#35221=CARTESIAN_POINT ( 'NONE',  ( -64.61430802170492882, 7.070445451047392638, 40.00000000000003553 ) ) ;
#35226=VECTOR ( 'NONE', #27192, 1000.000000000000114 ) ;
#35228=AXIS2_PLACEMENT_3D ( 'NONE', #7115, #22594, #50381 ) ;
#35231=DIRECTION ( 'NONE',  ( -1.000000000000000000, 0.000000000000000000, 0.000000000000000000 ) ) ;
#35232=DIRECTION ( 'NONE',  ( -0.9639628606958512425, -0.2660368455666826670, 0.000000000000000000 ) ) ;
#35235=CARTESIAN_POINT ( 'NONE',  ( 50.71116719115956073, 28.84239711592981337, 27.58472315868180402 ) ) ;
#35242=DIRECTION ( 'NONE',  ( -1.000000000000000000, 0.000000000000000000, 0.000000000000000000 ) ) ;
#35243=ORIENTED_EDGE ( 'NONE', *, *, #40571, .T. ) ;
#35244=EDGE_CURVE ( 'NONE', #23953, #17123, #65194, .T. ) ;
#35250=DIRECTION ( 'NONE',  ( -0.000000000000000000, -0.000000000000000000, -1.000000000000000000 ) ) ;
#35259=VECTOR ( 'NONE', #56708, 1000.000000000000000 ) ;
#35267=ORIENTED_EDGE ( 'NONE', *, *, #60222, .F. ) ;
#35268=CIRCLE ( 'NONE', #15030, 65.36598343705435354 ) ;
#35270=CARTESIAN_POINT ( 'NONE',  ( -6.214074258788039096, -32.84308722476502140, 6.893342931991226941 ) ) ;
#35274=VECTOR ( 'NONE', #20151, 1000.000000000000000 ) ;
#35275=PLANE ( 'NONE',  #5504 ) ;
#35284=ORIENTED_EDGE ( 'NONE', *, *, #29303, .T. ) ;
#35286=VERTEX_POINT ( 'NONE', #24568 ) ;
#35292=EDGE_CURVE ( 'NONE', #34668, #13679, #30182, .T. ) ;
#35296=EDGE_CURVE ( 'NONE', #36305, #6675, #41077, .T. ) ;
#35298=ORIENTED_EDGE ( 'NONE', *, *, #48882, .T. ) ;
#35316=VERTEX_POINT ( 'NONE', #3785 ) ;
#35322=CARTESIAN_POINT ( 'NONE',  ( -64.18058723658653264, 10.37664328995176888, 41.38025477438755928 ) ) ;
#35324=AXIS2_PLACEMENT_3D ( 'NONE', #38146, #11402, #6131 ) ;
#35327=CARTESIAN_POINT ( 'NONE',  ( -6.774725108395958983, 24.06456107444435233, 0.000000000000000000 ) ) ;
#35335=B_SPLINE_CURVE_WITH_KNOTS ( 'NONE', 3,
 ( #67693, #61704, #40946, #35327 ),
 .UNSPECIFIED., .F., .F.,
 ( 4, 4 ),
 ( 9.900409499073836656E-07, 0.05658314289920116785 ),
 .UNSPECIFIED. ) ;
#35345=EDGE_CURVE ( 'NONE', #43782, #67945, #51636, .T. ) ;
#35346=ORIENTED_EDGE ( 'NONE', *, *, #35179, .F. ) ;
#35351=EDGE_CURVE ( 'NONE', #55351, #28828, #35453, .T. ) ;
#35363=DIRECTION ( 'NONE',  ( 1.000000000000000000, 0.000000000000000000, 0.000000000000000000 ) ) ;
#35369=ORIENTED_EDGE ( 'NONE', *, *, #44601, .F. ) ;
#35372=CARTESIAN_POINT ( 'NONE',  ( 0.000000000000000000, 0.000000000000000000, 170.0000000000000000 ) ) ;
#35373=DIRECTION ( 'NONE',  ( 0.1342332658176667581, -0.9909497617679332571, 0.000000000000000000 ) ) ;
#35381=VECTOR ( 'NONE', #39714, 1000.000000000000000 ) ;
#35387=CARTESIAN_POINT ( 'NONE',  ( 69.72313848477121212, 27.50266661387133738, 41.38025477438755928 ) ) ;
#35388=CARTESIAN_POINT ( 'NONE',  ( -25.87147652227456263, 100.0000000000000000, 77.58025477438755502 ) ) ;
#35404=DIRECTION ( 'NONE',  ( 0.4738686624729966379, 0.8805955318567391110, -0.000000000000000000 ) ) ;
#35408=ADVANCED_FACE ( 'NONE', ( #4139 ), #62537, .T. ) ;
#35414=CARTESIAN_POINT ( 'NONE',  ( 14.77197020583827580, -49.50853448602472895, 26.66469104408690427 ) ) ;
#35419=EDGE_CURVE ( 'NONE', #33531, #13094, #47962, .T. ) ;
#35426=ORIENTED_EDGE ( 'NONE', *, *, #52318, .T. ) ;
#35428=VECTOR ( 'NONE', #69055, 1000.000000000000114 ) ;
#35429=ORIENTED_EDGE ( 'NONE', *, *, #17219, .T. ) ;
#35444=LINE ( 'NONE', #3431, #47089 ) ;
#35453=LINE ( 'NONE', #9070, #24789 ) ;
#35459=ORIENTED_EDGE ( 'NONE', *, *, #51461, .F. ) ;
#35462=CARTESIAN_POINT ( 'NONE',  ( 0.000000000000000000, 0.000000000000000000, 170.0000000000000000 ) ) ;
#35463=ORIENTED_EDGE ( 'NONE', *, *, #29394, .F. ) ;
#35469=DIRECTION ( 'NONE',  ( 5.055952397801357946E-18, -6.848752866791659805E-19, -1.000000000000000000 ) ) ;
#35471=PLANE ( 'NONE',  #60741 ) ;
#35475=DIRECTION ( 'NONE',  ( 0.000000000000000000, 0.000000000000000000, 1.000000000000000000 ) ) ;
#35490=LINE ( 'NONE', #52686, #34627 ) ;
#35500=CARTESIAN_POINT ( 'NONE',  ( 0.000000000000000000, 0.000000000000000000, 40.00000000000003553 ) ) ;
#35507=CARTESIAN_POINT ( 'NONE',  ( -84.49322488516129681, 0.000000000000000000, 43.58025477438756212 ) ) ;
#35508=VERTEX_POINT ( 'NONE', #69517 ) ;
#35521=AXIS2_PLACEMENT_3D ( 'NONE', #41624, #32108, #5372 ) ;
#35522=VECTOR ( 'NONE', #46568, 999.9999999999998863 ) ;
#35530=CIRCLE ( 'NONE', #62498, 63.00000000000000000 ) ;
#35547=CARTESIAN_POINT ( 'NONE',  ( 74.39890044415652426, -7.951074708186081530, 43.58025477438756923 ) ) ;
#35548=ORIENTED_EDGE ( 'NONE', *, *, #51238, .T. ) ;
#35549=CARTESIAN_POINT ( 'NONE',  ( -41.50537345350708307, 50.04124777106294886, 43.58025477438756923 ) ) ;
#35550=VERTEX_POINT ( 'NONE', #33991 ) ;
#35558=EDGE_CURVE ( 'NONE', #24043, #17523, #28133, .T. ) ;
#35564=CARTESIAN_POINT ( 'NONE',  ( 24.86543756664854143, -29.17542814769260318, 13.32819299319723250 ) ) ;
#35566=VECTOR ( 'NONE', #34349, 1000.000000000000000 ) ;
#35568=LINE ( 'NONE', #57028, #2685 ) ;
#35569=VECTOR ( 'NONE', #66718, 1000.000000000000000 ) ;
#35580=EDGE_CURVE ( 'NONE', #36414, #39565, #12888, .T. ) ;
#35581=EDGE_CURVE ( 'NONE', #57236, #65498, #28680, .T. ) ;
#35582=ORIENTED_EDGE ( 'NONE', *, *, #50364, .F. ) ;
#35588=ADVANCED_FACE ( 'NONE', ( #29066 ), #17446, .F. ) ;
#35590=CARTESIAN_POINT ( 'NONE',  ( 60.40479419793764038, 24.00543350795394915, 40.00000000000003553 ) ) ;
#35592=CARTESIAN_POINT ( 'NONE',  ( 18.89356949897823768, 62.19351277735707839, 170.0000000000000000 ) ) ;
#35596=ORIENTED_EDGE ( 'NONE', *, *, #31514, .T. ) ;
#35606=ADVANCED_FACE ( 'NONE', ( #43822 ), #65299, .T. ) ;
#35612=VECTOR ( 'NONE', #65671, 1000.000000000000000 ) ;
#35615=CARTESIAN_POINT ( 'NONE',  ( -45.81425895439360829, -46.10914959592906825, 170.0000000000000000 ) ) ;
#35620=AXIS2_PLACEMENT_3D ( 'NONE', #68049, #57483, #3326 ) ;
#35621=ORIENTED_EDGE ( 'NONE', *, *, #15715, .F. ) ;
#35624=LINE ( 'NONE', #57764, #66027 ) ;
#35628=FACE_OUTER_BOUND ( 'NONE', #62538, .T. ) ;
#35632=FACE_OUTER_BOUND ( 'NONE', #66293, .T. ) ;
#35633=EDGE_LOOP ( 'NONE', ( #47670, #51046, #33550, #23106 ) ) ;
#35639=VERTEX_POINT ( 'NONE', #29400 ) ;
#35642=CARTESIAN_POINT ( 'NONE',  ( 0.000000000000000000, 0.000000000000000000, 41.38025477438755928 ) ) ;
#35650=VERTEX_POINT ( 'NONE', #30441 ) ;
#35652=LINE ( 'NONE', #30367, #63043 ) ;
#35653=CARTESIAN_POINT ( 'NONE',  ( 0.000000000000000000, 0.000000000000000000, 170.0000000000000000 ) ) ;
#35654=B_SPLINE_CURVE_WITH_KNOTS ( 'NONE', 3,
 ( #4090, #4427, #20259, #41717, #47666, #31178 ),
 .UNSPECIFIED., .F., .F.,
 ( 4, 2, 4 ),
 ( 0.03218943375184197403, 0.06469838935233396260, 0.09720734495282595811 ),
 .UNSPECIFIED. ) ;
#35658=CARTESIAN_POINT ( 'NONE',  ( 0.000000000000000000, 0.000000000000000000, 0.000000000000000000 ) ) ;
#35663=CARTESIAN_POINT ( 'NONE',  ( 51.85299110299499148, -39.21848821248373440, 170.0000000000000000 ) ) ;
#35664=EDGE_CURVE ( 'NONE', #49951, #64171, #62800, .T. ) ;
#35665=B_SPLINE_CURVE_WITH_KNOTS ( 'NONE', 3,
 ( #68469, #51264, #14653, #24538 ),
 .UNSPECIFIED., .F., .F.,
 ( 4, 4 ),
 ( 0.1259919275528357530, 0.1829744153748744662 ),
 .UNSPECIFIED. ) ;
#35673=DIRECTION ( 'NONE',  ( -0.9909497617679331460, -0.1342332658176667304, 0.000000000000000000 ) ) ;
#35677=CARTESIAN_POINT ( 'NONE',  ( -26.07811460555694438, -76.21509903021816967, 133.5802547743875550 ) ) ;
#35694=FACE_OUTER_BOUND ( 'NONE', #15553, .T. ) ;
#35701=VERTEX_POINT ( 'NONE', #35728 ) ;
#35703=CARTESIAN_POINT ( 'NONE',  ( 44.01696072965949469, 47.84694004974210912, 0.000000000000000000 ) ) ;
#35709=VERTEX_POINT ( 'NONE', #67393 ) ;
#35712=CARTESIAN_POINT ( 'NONE',  ( -2.374459999240197572, -25.00999262126968148, 0.000000000000000000 ) ) ;
#35720=VERTEX_POINT ( 'NONE', #57177 ) ;
#35725=CARTESIAN_POINT ( 'NONE',  ( -24.17157287525367693, 5.337719384915982763E-15, 2.000000000000001776 ) ) ;
#35726=CARTESIAN_POINT ( 'NONE',  ( 14.66690460840507804, -20.39656099473392814, 0.000000000000000000 ) ) ;
#35728=CARTESIAN_POINT ( 'NONE',  ( -28.32746765835526048, 69.45586423092609607, 133.5802547743875550 ) ) ;
#35733=ORIENTED_EDGE ( 'NONE', *, *, #15901, .T. ) ;
#35734=AXIS2_PLACEMENT_3D ( 'NONE', #13069, #55263, #55615 ) ;
#35750=FACE_OUTER_BOUND ( 'NONE', #69158, .T. ) ;
#35751=EDGE_CURVE ( 'NONE', #35720, #20416, #47634, .T. ) ;
#35754=EDGE_CURVE ( 'NONE', #8487, #60309, #42028, .T. ) ;
#35756=VERTEX_POINT ( 'NONE', #47978 ) ;
#35758=CARTESIAN_POINT ( 'NONE',  ( 61.91366885787816443, -28.42865614898931881, 170.0000000000000000 ) ) ;
#35762=ORIENTED_EDGE ( 'NONE', *, *, #14208, .F. ) ;
#35766=ORIENTED_EDGE ( 'NONE', *, *, #49054, .F. ) ;
#35779=VERTEX_POINT ( 'NONE', #69445 ) ;
#35781=LINE ( 'NONE', #57230, #58669 ) ;
#35798=ORIENTED_EDGE ( 'NONE', *, *, #63761, .T. ) ;
#35800=DIRECTION ( 'NONE',  ( 0.6234898018587431423, -0.7818314824680220321, 0.000000000000000000 ) ) ;
#35801=LINE ( 'NONE', #3780, #51991 ) ;
#35809=EDGE_CURVE ( 'NONE', #8769, #32122, #42710, .T. ) ;
#35812=VERTEX_POINT ( 'NONE', #20226 ) ;
#35814=EDGE_CURVE ( 'NONE', #14487, #34211, #25864, .T. ) ;
#35815=CARTESIAN_POINT ( 'NONE',  ( 25.02868014889590498, -33.38981655027261297, 13.79046340968177731 ) ) ;
#35835=EDGE_CURVE ( 'NONE', #25430, #48110, #44615, .T. ) ;
#35843=ORIENTED_EDGE ( 'NONE', *, *, #7048, .F. ) ;
#35854=LINE ( 'NONE', #2806, #48753 ) ;
#35861=VECTOR ( 'NONE', #16388, 1000.000000000000000 ) ;
#35862=LINE ( 'NONE', #68884, #28654 ) ;
#35868=ORIENTED_EDGE ( 'NONE', *, *, #27312, .F. ) ;
#35876=ORIENTED_EDGE ( 'NONE', *, *, #65850, .T. ) ;
#35882=EDGE_CURVE ( 'NONE', #54393, #26798, #64804, .T. ) ;
#35892=PLANE ( 'NONE',  #11601 ) ;
#35899=CARTESIAN_POINT ( 'NONE',  ( -64.18058723658653264, 10.37664328995176888, 170.0000000000000000 ) ) ;
#35908=VERTEX_POINT ( 'NONE', #33571 ) ;
#35910=DIRECTION ( 'NONE',  ( -0.8090169943749422332, -0.5877852522924802425, 0.000000000000000000 ) ) ;
#35914=LINE ( 'NONE', #18698, #33000 ) ;
#35916=VECTOR ( 'NONE', #51099, 1000.000000000000000 ) ;
#35930=LINE ( 'NONE', #67599, #26478 ) ;
#35932=CIRCLE ( 'NONE', #23581, 65.36598343705435354 ) ;
#35953=CARTESIAN_POINT ( 'NONE',  ( -7.486743542469089796, -64.58150799671139453, 43.58025477438756923 ) ) ;
#35967=EDGE_CURVE ( 'NONE', #14985, #22952, #65216, .T. ) ;
#35976=ORIENTED_EDGE ( 'NONE', *, *, #3964, .F. ) ;
#35978=FACE_OUTER_BOUND ( 'NONE', #52116, .T. ) ;
#35980=EDGE_CURVE ( 'NONE', #6273, #47103, #6815, .T. ) ;
#35981=DIRECTION ( 'NONE',  ( 1.000000000000000000, 0.000000000000000000, 0.000000000000000000 ) ) ;
#35996=EDGE_CURVE ( 'NONE', #1913, #65404, #17733, .T. ) ;
#35998=ADVANCED_FACE ( 'NONE', ( #38125 ), #17362, .F. ) ;
#36000=ORIENTED_EDGE ( 'NONE', *, *, #28263, .F. ) ;
#36001=DIRECTION ( 'NONE',  ( -0.000000000000000000, -0.000000000000000000, -1.000000000000000000 ) ) ;
#36017=DIRECTION ( 'NONE',  ( 0.000000000000000000, -0.000000000000000000, -1.000000000000000000 ) ) ;
#36022=DIRECTION ( 'NONE',  ( 0.8345732537212999791, 0.5508969814521065267, 0.000000000000000000 ) ) ;
#36023=ORIENTED_EDGE ( 'NONE', *, *, #14986, .T. ) ;
#36026=FACE_OUTER_BOUND ( 'NONE', #39949, .T. ) ;
#36028=CARTESIAN_POINT ( 'NONE',  ( -46.06722295615723795, -46.37372919877118704, 6.377659838150142862E-18 ) ) ;
#36029=CARTESIAN_POINT ( 'NONE',  ( 6.564829507346455983, -24.24955267099640110, 0.000000000000000000 ) ) ;
#36032=AXIS2_PLACEMENT_3D ( 'NONE', #29786, #8342, #25217 ) ;
#36033=EDGE_CURVE ( 'NONE', #16881, #68798, #496, .T. ) ;
#36036=CARTESIAN_POINT ( 'NONE',  ( -2.116120943111210906, -74.98056102853675497, 170.0000000000000000 ) ) ;
#36041=CARTESIAN_POINT ( 'NONE',  ( 65.02478361689730946, 37.39438481344068776, 170.0000000000000000 ) ) ;
#36042=CARTESIAN_POINT ( 'NONE',  ( 0.000000000000000000, 0.000000000000000000, 41.38025477438755928 ) ) ;
#36045=ORIENTED_EDGE ( 'NONE', *, *, #17243, .F. ) ;
#36049=CARTESIAN_POINT ( 'NONE',  ( 64.08056813503714011, -12.89932471814424986, 43.58025477438756212 ) ) ;
#36050=CARTESIAN_POINT ( 'NONE',  ( 21.27121078971695312, -61.42097029141944375, 40.00000000000003553 ) ) ;
#36061=CARTESIAN_POINT ( 'NONE',  ( 0.000000000000000000, 0.000000000000000000, 0.000000000000000000 ) ) ;
#36069=ORIENTED_EDGE ( 'NONE', *, *, #38744, .T. ) ;
#36070=ORIENTED_EDGE ( 'NONE', *, *, #623, .T. ) ;
#36071=ORIENTED_EDGE ( 'NONE', *, *, #38589, .F. ) ;
#36080=CARTESIAN_POINT ( 'NONE',  ( -60.67627457812066183, -44.08389392193601708, 43.58025477438756212 ) ) ;
#36084=AXIS2_PLACEMENT_3D ( 'NONE', #6147, #49049, #65612 ) ;
#36098=VECTOR ( 'NONE', #56833, 1000.000000000000000 ) ;
#36099=CARTESIAN_POINT ( 'NONE',  ( -21.27554331372908081, -61.43430442924895374, 170.0000000000000000 ) ) ;
#36118=CARTESIAN_POINT ( 'NONE',  ( -50.12142425878460728, 12.53590371354408894, 26.66469066592269144 ) ) ;
#36122=EDGE_CURVE ( 'NONE', #25478, #6992, #24403, .T. ) ;
#36126=CARTESIAN_POINT ( 'NONE',  ( -29.87147652227456263, -74.98256102853682137, 73.58025477438756923 ) ) ;
#36130=AXIS2_PLACEMENT_3D ( 'NONE', #4369, #15611, #36376 ) ;
#36137=ORIENTED_EDGE ( 'NONE', *, *, #59243, .T. ) ;
#36141=VECTOR ( 'NONE', #19802, 1000.000000000000000 ) ;
#36147=DIRECTION ( 'NONE',  ( -0.1342332658176667304, 0.9909497617679331460, 0.000000000000000000 ) ) ;
#36179=CARTESIAN_POINT ( 'NONE',  ( -65.00200000000002376, -1.250000000000021094, 170.0000000000000000 ) ) ;
#36184=CARTESIAN_POINT ( 'NONE',  ( 0.000000000000000000, 0.000000000000000000, 170.0000000000000000 ) ) ;
#36191=CIRCLE ( 'NONE', #66538, 24.99999999999985434 ) ;
#36192=ORIENTED_EDGE ( 'NONE', *, *, #65862, .T. ) ;
#36207=DIRECTION ( 'NONE',  ( 1.000000000000000000, 0.000000000000000000, 0.000000000000000000 ) ) ;
#36226=VECTOR ( 'NONE', #19938, 1000.000000000000000 ) ;
#36250=EDGE_CURVE ( 'NONE', #22437, #11268, #61874, .T. ) ;
#36253=FACE_OUTER_BOUND ( 'NONE', #10573, .T. ) ;
#36255=CARTESIAN_POINT ( 'NONE',  ( 0.000000000000000000, 0.000000000000000000, 170.0000000000000000 ) ) ;
#36256=B_SPLINE_CURVE_WITH_KNOTS ( 'NONE', 3,
 ( #54990, #22643, #59562, #33208 ),
 .UNSPECIFIED., .F., .F.,
 ( 4, 4 ),
 ( 0.1259919275528365301, 0.1829744153748764923 ),
 .UNSPECIFIED. ) ;
#36258=ORIENTED_EDGE ( 'NONE', *, *, #62688, .T. ) ;
#36259=CYLINDRICAL_SURFACE ( 'NONE', #30045, 65.00000000000000000 ) ;
#36266=ORIENTED_EDGE ( 'NONE', *, *, #41530, .T. ) ;
#36267=CARTESIAN_POINT ( 'NONE',  ( 64.16679220703380793, -10.37413986118096254, 170.0000000000000000 ) ) ;
#36275=ADVANCED_FACE ( 'NONE', ( #16078 ), #33820, .T. ) ;
#36282=VERTEX_POINT ( 'NONE', #48408 ) ;
#36287=EDGE_CURVE ( 'NONE', #33243, #26373, #64669, .T. ) ;
#36288=CIRCLE ( 'NONE', #46414, 24.99999999999985434 ) ;
#36294=DIRECTION ( 'NONE',  ( 0.7530714660036195163, -0.6579387259397027066, 0.000000000000000000 ) ) ;
#36299=CARTESIAN_POINT ( 'NONE',  ( 0.000000000000000000, 0.000000000000000000, 43.58025477438756212 ) ) ;
#36300=ADVANCED_FACE ( 'NONE', ( #44186 ), #11842, .T. ) ;
#36305=VERTEX_POINT ( 'NONE', #39286 ) ;
#36308=CARTESIAN_POINT ( 'NONE',  ( -13.24252603915608617, 63.63674649211943546, 170.0000000000000000 ) ) ;
#36313=FACE_OUTER_BOUND ( 'NONE', #52710, .T. ) ;
#36315=DIRECTION ( 'NONE',  ( 0.4338837391175526248, 0.9009688679024218105, 0.000000000000000000 ) ) ;
#36321=CARTESIAN_POINT ( 'NONE',  ( 0.000000000000000000, 0.000000000000000000, 0.000000000000000000 ) ) ;
#36333=ORIENTED_EDGE ( 'NONE', *, *, #45037, .T. ) ;
#36336=VECTOR ( 'NONE', #17840, 1000.000000000000000 ) ;
#36338=AXIS2_PLACEMENT_3D ( 'NONE', #20177, #25811, #63087 ) ;
#36352=CARTESIAN_POINT ( 'NONE',  ( -29.47687737404360675, -68.96458294135908318, 0.000000000000000000 ) ) ;
#36362=EDGE_CURVE ( 'NONE', #47461, #50613, #55809, .T. ) ;
#36369=ORIENTED_EDGE ( 'NONE', *, *, #16732, .T. ) ;
#36371=LINE ( 'NONE', #57830, #10605 ) ;
#36375=CARTESIAN_POINT ( 'NONE',  ( 9.133089968245061030, -32.15384561068184865, 6.893343212288923993 ) ) ;
#36376=DIRECTION ( 'NONE',  ( 1.000000000000000000, 0.000000000000000000, 0.000000000000000000 ) ) ;
#36378=CARTESIAN_POINT ( 'NONE',  ( -65.36598343705435354, 0.000000000000000000, 41.38025477438755928 ) ) ;
#36389=DIRECTION ( 'NONE',  ( -0.04486483035051862939, 0.9989930665413143673, 0.000000000000000000 ) ) ;
#36392=ORIENTED_EDGE ( 'NONE', *, *, #65209, .T. ) ;
#36393=EDGE_LOOP ( 'NONE', ( #26042, #9557, #12138, #46324 ) ) ;
#36409=CARTESIAN_POINT ( 'NONE',  ( 48.11816970607237209, 43.69944786994017250, 40.00000000000003553 ) ) ;
#36414=VERTEX_POINT ( 'NONE', #39972 ) ;
#36415=VECTOR ( 'NONE', #67715, 1000.000000000000000 ) ;
#36416=CARTESIAN_POINT ( 'NONE',  ( 16.00641379534997455, -64.51123194475178479, 133.5802547743875550 ) ) ;
#36440=PLANE ( 'NONE',  #33162 ) ;
#36441=CARTESIAN_POINT ( 'NONE',  ( -15.67984581961064450, 63.08044415722863363, 133.5802547743875550 ) ) ;
#36443=ORIENTED_EDGE ( 'NONE', *, *, #56327, .T. ) ;
#36445=EDGE_CURVE ( 'NONE', #58070, #12845, #44902, .T. ) ;
#36449=ORIENTED_EDGE ( 'NONE', *, *, #18981, .T. ) ;
#36451=VERTEX_POINT ( 'NONE', #46976 ) ;
#36454=DIRECTION ( 'NONE',  ( 0.000000000000000000, 0.000000000000000000, 1.000000000000000000 ) ) ;
#36461=VERTEX_POINT ( 'NONE', #15314 ) ;
#36469=ORIENTED_EDGE ( 'NONE', *, *, #26104, .F. ) ;
#36475=AXIS2_PLACEMENT_3D ( 'NONE', #65154, #33843, #38412 ) ;
#36480=AXIS2_PLACEMENT_3D ( 'NONE', #58928, #36454, #5473 ) ;
#36482=CARTESIAN_POINT ( 'NONE',  ( -24.39249304643438521, 60.24953346690454481, 170.0000000000000000 ) ) ;
#36485=EDGE_LOOP ( 'NONE', ( #19411, #8634, #3382, #67193 ) ) ;
#36495=EDGE_LOOP ( 'NONE', ( #30892, #49427, #26739, #48473 ) ) ;
#36505=CARTESIAN_POINT ( 'NONE',  ( -53.31111153860250340, -37.18770477615797176, 170.0000000000000000 ) ) ;
#36509=EDGE_CURVE ( 'NONE', #60060, #21253, #46156, .T. ) ;
#36514=CARTESIAN_POINT ( 'NONE',  ( 0.000000000000000000, 0.000000000000000000, 170.0000000000000000 ) ) ;
#36525=CARTESIAN_POINT ( 'NONE',  ( 39.54205320694339321, 51.58901073076764021, 170.0000000000000000 ) ) ;
#36526=CARTESIAN_POINT ( 'NONE',  ( -55.15976438495155776, 34.41253982194033512, 43.58025477438756923 ) ) ;
#36538=CIRCLE ( 'NONE', #63495, 25.12245591505646303 ) ;
#36546=CARTESIAN_POINT ( 'NONE',  ( 75.00000000000000000, 0.000000000000000000, 0.000000000000000000 ) ) ;
#36554=ORIENTED_EDGE ( 'NONE', *, *, #36122, .T. ) ;
#36557=EDGE_CURVE ( 'NONE', #38023, #65787, #25800, .T. ) ;
#36558=ADVANCED_FACE ( 'NONE', ( #30375 ), #46897, .F. ) ;
#36563=DIRECTION ( 'NONE',  ( -1.156482317317871232E-16, 0.000000000000000000, -1.000000000000000000 ) ) ;
#36569=DIRECTION ( 'NONE',  ( -0.000000000000000000, -0.000000000000000000, 1.000000000000000000 ) ) ;
#36584=CARTESIAN_POINT ( 'NONE',  ( -4.364688291132793552, 24.74039788130344419, 0.000000000000000000 ) ) ;
#36596=ORIENTED_EDGE ( 'NONE', *, *, #29454, .T. ) ;
#36598=DIRECTION ( 'NONE',  ( -0.6910626489868685329, 0.7227948638273878901, 0.000000000000000000 ) ) ;
#36599=VERTEX_POINT ( 'NONE', #31414 ) ;
#36609=EDGE_LOOP ( 'NONE', ( #44239, #17252, #22325, #42126 ) ) ;
#36614=ADVANCED_FACE ( 'NONE', ( #32447 ), #32789, .F. ) ;
#36616=CIRCLE ( 'NONE', #69130, 65.36598343705435354 ) ;
#36625=LINE ( 'NONE', #8155, #37712 ) ;
#36635=ORIENTED_EDGE ( 'NONE', *, *, #49395, .T. ) ;
#36640=VERTEX_POINT ( 'NONE', #28201 ) ;
#36653=DIRECTION ( 'NONE',  ( -0.9959742939952382912, -0.08963930890344087854, 0.000000000000000000 ) ) ;
#36657=CARTESIAN_POINT ( 'NONE',  ( 34.76618902119740540, 54.93755186520760958, 170.0000000000000000 ) ) ;
#36658=CARTESIAN_POINT ( 'NONE',  ( 11.29825944729837062, -74.09495289492984682, 41.38025477438755928 ) ) ;
#36671=CARTESIAN_POINT ( 'NONE',  ( 16.54503815046424009, 18.74197728628641002, 0.000000000000000000 ) ) ;
#36672=AXIS2_PLACEMENT_3D ( 'NONE', #6309, #33047, #5948 ) ;
#36673=CARTESIAN_POINT ( 'NONE',  ( 0.000000000000000000, 0.000000000000000000, 41.38025477438755928 ) ) ;
#36676=PLANE ( 'NONE',  #10359 ) ;
#36677=AXIS2_PLACEMENT_3D ( 'NONE', #52271, #62485, #41721 ) ;
#36684=ORIENTED_EDGE ( 'NONE', *, *, #35835, .T. ) ;
#36694=DIRECTION ( 'NONE',  ( -0.9639628606958550172, 0.2660368455666687892, 0.000000000000000000 ) ) ;
#36696=CARTESIAN_POINT ( 'NONE',  ( 74.62299871641508275, -5.461138973197948054, 0.000000000000000000 ) ) ;
#36697=DIRECTION ( 'NONE',  ( 0.000000000000000000, 0.000000000000000000, 1.000000000000000000 ) ) ;
#36704=ORIENTED_EDGE ( 'NONE', *, *, #49118, .F. ) ;
#36713=LINE ( 'NONE', #42995, #41490 ) ;
#36721=CARTESIAN_POINT ( 'NONE',  ( -42.36049017605959932, 61.90437280228238137, 170.0000000000000000 ) ) ;
#36722=VERTEX_POINT ( 'NONE', #12382 ) ;
#36723=VECTOR ( 'NONE', #69207, 999.9999999999998863 ) ;
#36738=CARTESIAN_POINT ( 'NONE',  ( 24.34685647902980676, 70.88683439560453792, 41.38025477438755928 ) ) ;
#36739=VERTEX_POINT ( 'NONE', #24339 ) ;
#36758=CARTESIAN_POINT ( 'NONE',  ( 34.76618902119821541, -54.93755186520709799, 41.38025477438755928 ) ) ;
#36760=CARTESIAN_POINT ( 'NONE',  ( 74.01791526339570737, -12.16185512414842051, 43.58025477438756923 ) ) ;
#36761=ORIENTED_EDGE ( 'NONE', *, *, #498, .F. ) ;
#36764=ORIENTED_EDGE ( 'NONE', *, *, #66672, .T. ) ;
#36766=CARTESIAN_POINT ( 'NONE',  ( 0.000000000000000000, 0.000000000000000000, 41.38025477438755928 ) ) ;
#36779=FACE_OUTER_BOUND ( 'NONE', #10357, .T. ) ;
#36780=DIRECTION ( 'NONE',  ( -1.000000000000000000, 0.000000000000000000, 0.000000000000000000 ) ) ;
#36784=CARTESIAN_POINT ( 'NONE',  ( 34.76618902119820831, -54.93755186520709799, 3.061616997868437868E-16 ) ) ;
#36795=ORIENTED_EDGE ( 'NONE', *, *, #39384, .F. ) ;
#36797=DIRECTION ( 'NONE',  ( 0.000000000000000000, 0.000000000000000000, -1.000000000000000000 ) ) ;
#36804=CARTESIAN_POINT ( 'NONE',  ( 47.73902449248994628, 57.85799893277891215, 170.0000000000000000 ) ) ;
#36809=VECTOR ( 'NONE', #53040, 1000.000000000000000 ) ;
#36811=ORIENTED_EDGE ( 'NONE', *, *, #6745, .T. ) ;
#36812=ORIENTED_EDGE ( 'NONE', *, *, #11660, .F. ) ;
#36820=VERTEX_POINT ( 'NONE', #32706 ) ;
#36824=ORIENTED_EDGE ( 'NONE', *, *, #49458, .T. ) ;
#36829=CARTESIAN_POINT ( 'NONE',  ( -61.29635759142615115, 21.66977272663494958, 43.58025477438756923 ) ) ;
#36832=EDGE_LOOP ( 'NONE', ( #66802, #47574, #51803, #22279 ) ) ;
#36843=VERTEX_POINT ( 'NONE', #65067 ) ;
#36845=ADVANCED_FACE ( 'NONE', ( #16866 ), #700, .T. ) ;
#36846=ORIENTED_EDGE ( 'NONE', *, *, #3203, .F. ) ;
#36852=DIRECTION ( 'NONE',  ( 0.9749279121818227312, 0.2225209339563184729, 5.102127870520021228E-18 ) ) ;
#36861=CARTESIAN_POINT ( 'NONE',  ( -39.40355473380300566, -43.02169567653766080, 27.58472369436602634 ) ) ;
#36868=EDGE_CURVE ( 'NONE', #58577, #24108, #34977, .T. ) ;
#36874=ADVANCED_FACE ( 'NONE', ( #10898 ), #64028, .T. ) ;
#36877=CONICAL_SURFACE ( 'NONE', #6537, 74.95140232871122521, 0.8777644062502172329 ) ;
#36879=ORIENTED_EDGE ( 'NONE', *, *, #42666, .T. ) ;
#36887=DIRECTION ( 'NONE',  ( 0.3513748240813435175, -0.9362348706397369824, 0.000000000000000000 ) ) ;
#36901=CARTESIAN_POINT ( 'NONE',  ( 0.000000000000000000, 0.000000000000000000, 43.58025477438756212 ) ) ;
#36906=EDGE_CURVE ( 'NONE', #44801, #32676, #56309, .T. ) ;
#36918=CARTESIAN_POINT ( 'NONE',  ( -71.96466849523078224, 21.15771699336999845, 170.0000000000000000 ) ) ;
#36919=FACE_OUTER_BOUND ( 'NONE', #56908, .T. ) ;
#36921=DIRECTION ( 'NONE',  ( 0.000000000000000000, 0.000000000000000000, 1.000000000000000000 ) ) ;
#36927=LINE ( 'NONE', #30618, #45364 ) ;
#36931=EDGE_CURVE ( 'NONE', #60956, #69323, #10096, .T. ) ;
#36934=LINE ( 'NONE', #679, #822 ) ;
#36936=EDGE_CURVE ( 'NONE', #67695, #4696, #31604, .T. ) ;
#36941=ORIENTED_EDGE ( 'NONE', *, *, #31145, .T. ) ;
#36950=EDGE_CURVE ( 'NONE', #20231, #55364, #19245, .T. ) ;
#36961=B_SPLINE_CURVE_WITH_KNOTS ( 'NONE', 3,
 ( #58253, #51944, #9044, #10069 ),
 .UNSPECIFIED., .F., .F.,
 ( 4, 4 ),
 ( 0.1259919275528361138, 0.1829744153748754099 ),
 .UNSPECIFIED. ) ;
#36963=AXIS2_PLACEMENT_3D ( 'NONE', #34991, #56433, #56794 ) ;
#36964=VERTEX_POINT ( 'NONE', #49215 ) ;
#36992=DIRECTION ( 'NONE',  ( -0.08963930890344089242, 0.9959742939952384022, 5.102127870520021228E-18 ) ) ;
#37002=CARTESIAN_POINT ( 'NONE',  ( -61.29635759142615115, 21.66977272663494958, 0.000000000000000000 ) ) ;
#37004=ORIENTED_EDGE ( 'NONE', *, *, #39922, .T. ) ;
#37007=ORIENTED_EDGE ( 'NONE', *, *, #29864, .T. ) ;
#37009=CARTESIAN_POINT ( 'NONE',  ( -45.99287096254393248, -23.53639463186987868, 26.66469066592268078 ) ) ;
#37014=CARTESIAN_POINT ( 'NONE',  ( 0.000000000000000000, 0.000000000000000000, 41.38025477438755928 ) ) ;
#37018=CIRCLE ( 'NONE', #50479, 25.12245591505646303 ) ;
#37048=VERTEX_POINT ( 'NONE', #63512 ) ;
#37049=DIRECTION ( 'NONE',  ( 0.9959742939952382912, 0.08963930890344089242, 0.000000000000000000 ) ) ;
#37057=LINE ( 'NONE', #4366, #30863 ) ;
#37060=VECTOR ( 'NONE', #58408, 1000.000000000000000 ) ;
#37064=ADVANCED_FACE ( 'NONE', ( #31847 ), #26569, .T. ) ;
#37071=CARTESIAN_POINT ( 'NONE',  ( 1.667562369267748368, -64.99262834925670518, 3.061616997868437868E-16 ) ) ;
#37085=VERTEX_POINT ( 'NONE', #59949 ) ;
#37087=ORIENTED_EDGE ( 'NONE', *, *, #49796, .T. ) ;
#37098=ORIENTED_EDGE ( 'NONE', *, *, #15473, .T. ) ;
#37102=B_SPLINE_CURVE_WITH_KNOTS ( 'NONE', 3,
 ( #38362, #59462, #5319, #53490, #43280, #5649 ),
 .UNSPECIFIED., .F., .F.,
 ( 4, 2, 4 ),
 ( 1.095770181115393514E-06, 0.03239442681617710901, 0.06478775786217311206 ),
 .UNSPECIFIED. ) ;
#37103=CARTESIAN_POINT ( 'NONE',  ( -6.802008071587034799, -24.18409554641273473, 0.000000000000000000 ) ) ;
#37106=ORIENTED_EDGE ( 'NONE', *, *, #27151, .F. ) ;
#37127=FACE_OUTER_BOUND ( 'NONE', #3334, .T. ) ;
#37131=ORIENTED_EDGE ( 'NONE', *, *, #38334, .T. ) ;
#37134=CARTESIAN_POINT ( 'NONE',  ( 36.85262215550071119, 53.56030941157734304, 3.061616997868437868E-16 ) ) ;
#37137=ADVANCED_FACE ( 'NONE', ( #49737 ), #48682, .T. ) ;
#37139=DIRECTION ( 'NONE',  ( 0.000000000000000000, 0.000000000000000000, 1.000000000000000000 ) ) ;
#37155=LINE ( 'NONE', #9055, #60323 ) ;
#37157=DIRECTION ( 'NONE',  ( -0.000000000000000000, -0.000000000000000000, -1.000000000000000000 ) ) ;
#37161=EDGE_LOOP ( 'NONE', ( #49493, #13240, #2748, #56948 ) ) ;
#37166=CARTESIAN_POINT ( 'NONE',  ( -39.55079474733700096, 51.59997227570983114, 41.38025477438755928 ) ) ;
#37175=ORIENTED_EDGE ( 'NONE', *, *, #14938, .F. ) ;
#37180=DIRECTION ( 'NONE',  ( -0.000000000000000000, -0.000000000000000000, 1.000000000000000000 ) ) ;
#37183=DIRECTION ( 'NONE',  ( -0.8090169943749506709, 0.5877852522924686962, 0.000000000000000000 ) ) ;
#37187=VERTEX_POINT ( 'NONE', #65237 ) ;
#37200=LINE ( 'NONE', #16092, #9369 ) ;
#37212=VERTEX_POINT ( 'NONE', #1567 ) ;
#37216=FACE_OUTER_BOUND ( 'NONE', #56013, .T. ) ;
#37217=ORIENTED_EDGE ( 'NONE', *, *, #66672, .F. ) ;
#37219=EDGE_CURVE ( 'NONE', #20457, #65969, #22326, .T. ) ;
#37239=VERTEX_POINT ( 'NONE', #26908 ) ;
#37248=CARTESIAN_POINT ( 'NONE',  ( 8.828807734114020533, 74.48902371486721563, 170.0000000000000000 ) ) ;
#37255=CARTESIAN_POINT ( 'NONE',  ( 1.667562369266827327, 64.99262834925669097, 170.0000000000000000 ) ) ;
#37259=VECTOR ( 'NONE', #53546, 999.9999999999998863 ) ;
#37262=ORIENTED_EDGE ( 'NONE', *, *, #41443, .T. ) ;
#37266=ORIENTED_EDGE ( 'NONE', *, *, #34942, .T. ) ;
#37269=AXIS2_PLACEMENT_3D ( 'NONE', #16574, #65473, #16227 ) ;
#37272=DIRECTION ( 'NONE',  ( -0.6234898018587431423, 0.7818314824680220321, 0.000000000000000000 ) ) ;
#37275=EDGE_LOOP ( 'NONE', ( #51057, #2290, #30394, #31026 ) ) ;
#37286=EDGE_CURVE ( 'NONE', #36843, #14304, #44113, .T. ) ;
#37289=LINE ( 'NONE', #64035, #1971 ) ;
#37292=DIRECTION ( 'NONE',  ( 0.000000000000000000, 0.000000000000000000, -1.000000000000000000 ) ) ;
#37298=ORIENTED_EDGE ( 'NONE', *, *, #32385, .T. ) ;
#37302=EDGE_CURVE ( 'NONE', #12108, #64034, #45871, .T. ) ;
#37306=EDGE_CURVE ( 'NONE', #59358, #1423, #67342, .T. ) ;
#37309=VECTOR ( 'NONE', #53395, 1000.000000000000000 ) ;
#37315=CARTESIAN_POINT ( 'NONE',  ( 0.000000000000000000, 0.000000000000000000, 41.38025477438755928 ) ) ;
#37320=EDGE_CURVE ( 'NONE', #33172, #53230, #45521, .T. ) ;
#37324=CARTESIAN_POINT ( 'NONE',  ( 22.93737758745385946, -9.943676855698914352, 0.000000000000000000 ) ) ;
#37328=DIRECTION ( 'NONE',  ( -0.000000000000000000, -0.000000000000000000, -1.000000000000000000 ) ) ;
#37330=CARTESIAN_POINT ( 'NONE',  ( -63.33140416796831573, -16.18162651919486095, 41.38025477438755928 ) ) ;
#37335=ORIENTED_EDGE ( 'NONE', *, *, #34823, .F. ) ;
#37337=ORIENTED_EDGE ( 'NONE', *, *, #68060, .F. ) ;
#37339=ORIENTED_EDGE ( 'NONE', *, *, #41634, .T. ) ;
#37341=DIRECTION ( 'NONE',  ( 0.000000000000000000, 0.000000000000000000, 1.000000000000000000 ) ) ;
#37348=EDGE_LOOP ( 'NONE', ( #56989, #41773, #9030, #38875 ) ) ;
#37351=DIRECTION ( 'NONE',  ( -0.3513748240813305279, -0.9362348706397418674, 0.000000000000000000 ) ) ;
#37355=CARTESIAN_POINT ( 'NONE',  ( -1.666933348992582609, 64.97862212458815634, 73.58025477438755502 ) ) ;
#37356=ORIENTED_EDGE ( 'NONE', *, *, #31767, .T. ) ;
#37364=CARTESIAN_POINT ( 'NONE',  ( 30.47484967065694761, -59.26962189778872414, 34.48241795236665297 ) ) ;
#37367=B_SPLINE_CURVE_WITH_KNOTS ( 'NONE', 3,
 ( #29191, #50633, #66151, #1064, #12316, #12664 ),
 .UNSPECIFIED., .F., .F.,
 ( 4, 2, 4 ),
 ( 0.03218932929355812489, 0.06469831333814424212, 0.09720729738273037324 ),
 .UNSPECIFIED. ) ;
#37369=AXIS2_PLACEMENT_3D ( 'NONE', #10040, #59251, #43414 ) ;
#37370=ORIENTED_EDGE ( 'NONE', *, *, #31782, .T. ) ;
#37373=VECTOR ( 'NONE', #8724, 999.9999999999998863 ) ;
#37378=ORIENTED_EDGE ( 'NONE', *, *, #47604, .F. ) ;
#37381=ADVANCED_FACE ( 'NONE', ( #57462 ), #26489, .T. ) ;
#37383=VERTEX_POINT ( 'NONE', #46906 ) ;
#37387=CARTESIAN_POINT ( 'NONE',  ( -25.87147652227456263, 100.0000000000000000, 77.58025477438755502 ) ) ;
#37388=LINE ( 'NONE', #36721, #48177 ) ;
#37389=ORIENTED_EDGE ( 'NONE', *, *, #40906, .F. ) ;
#37393=EDGE_CURVE ( 'NONE', #31642, #55255, #51835, .T. ) ;
#37397=ORIENTED_EDGE ( 'NONE', *, *, #2556, .T. ) ;
#37402=PLANE ( 'NONE',  #22575 ) ;
#37406=ORIENTED_EDGE ( 'NONE', *, *, #11199, .F. ) ;
#37407=VECTOR ( 'NONE', #47539, 1000.000000000000000 ) ;
#37410=ORIENTED_EDGE ( 'NONE', *, *, #66424, .T. ) ;
#37415=AXIS2_PLACEMENT_3D ( 'NONE', #49684, #22978, #7140 ) ;
#37416=DIRECTION ( 'NONE',  ( 1.000000000000000000, 0.000000000000000000, 0.000000000000000000 ) ) ;
#37417=DIRECTION ( 'NONE',  ( 0.000000000000000000, 1.000000000000000000, -0.000000000000000000 ) ) ;
#37422=ORIENTED_EDGE ( 'NONE', *, *, #19381, .F. ) ;
#37440=VERTEX_POINT ( 'NONE', #52183 ) ;
#37465=EDGE_CURVE ( 'NONE', #59098, #48854, #62748, .T. ) ;
#37468=VERTEX_POINT ( 'NONE', #14211 ) ;
#37471=EDGE_CURVE ( 'NONE', #417, #35550, #9629, .T. ) ;
#37475=DIRECTION ( 'NONE',  ( -0.1342332658176522420, -0.9909497617679352555, 0.000000000000000000 ) ) ;
#37492=ORIENTED_EDGE ( 'NONE', *, *, #46593, .T. ) ;
#37494=ORIENTED_EDGE ( 'NONE', *, *, #14142, .F. ) ;
#37500=AXIS2_PLACEMENT_3D ( 'NONE', #6778, #38445, #1504 ) ;
#37508=CARTESIAN_POINT ( 'NONE',  ( 0.000000000000000000, 0.000000000000000000, 170.0000000000000000 ) ) ;
#37545=VERTEX_POINT ( 'NONE', #48600 ) ;
#37546=EDGE_CURVE ( 'NONE', #20826, #50073, #33514, .T. ) ;
#37553=EDGE_LOOP ( 'NONE', ( #64871, #22580, #47044, #57090, #45136, #58921, #45334, #40375, #49915 ) ) ;
#37558=EDGE_CURVE ( 'NONE', #25097, #2530, #438, .T. ) ;
#37560=EDGE_CURVE ( 'NONE', #38758, #44050, #201, .T. ) ;
#37567=CARTESIAN_POINT ( 'NONE',  ( -20.93485882276955579, 13.66498028065538861, 0.000000000000000000 ) ) ;
#37573=VERTEX_POINT ( 'NONE', #5378 ) ;
#37578=CARTESIAN_POINT ( 'NONE',  ( 63.58578643762691485, 0.000000000000000000, 41.41421356237313489 ) ) ;
#37581=CARTESIAN_POINT ( 'NONE',  ( -74.81012118577227454, 5.477980300262931479, 43.58025477438756923 ) ) ;
#37585=DIRECTION ( 'NONE',  ( -8.784520486427686400E-17, -2.340627113153429324E-16, 1.000000000000000000 ) ) ;
#37590=ORIENTED_EDGE ( 'NONE', *, *, #40010, .T. ) ;
#37597=CARTESIAN_POINT ( 'NONE',  ( 18.07314801315378006, 17.44990292519104003, 3.061616997868437868E-16 ) ) ;
#37600=DIRECTION ( 'NONE',  ( 1.000000000000000000, 0.000000000000000000, 0.000000000000000000 ) ) ;
#37615=EDGE_LOOP ( 'NONE', ( #53102, #21005 ) ) ;
#37626=EDGE_CURVE ( 'NONE', #56020, #20206, #8152, .T. ) ;
#37634=LINE ( 'NONE', #16533, #45956 ) ;
#37635=CARTESIAN_POINT ( 'NONE',  ( 0.000000000000000000, 0.000000000000000000, 0.000000000000000000 ) ) ;
#37637=DIRECTION ( 'NONE',  ( 0.9195277725514489076, 0.3930250316539278810, -2.126835218476880762E-16 ) ) ;
#37641=CARTESIAN_POINT ( 'NONE',  ( -62.31345272479883590, -18.49415068377726357, 170.0000000000000000 ) ) ;
#37646=ORIENTED_EDGE ( 'NONE', *, *, #363, .T. ) ;
#37648=ORIENTED_EDGE ( 'NONE', *, *, #47796, .F. ) ;
#37655=CARTESIAN_POINT ( 'NONE',  ( -18.24318075359480318, 17.27206262134385284, 3.061616997868437868E-16 ) ) ;
#37658=VECTOR ( 'NONE', #59682, 1000.000000000000000 ) ;
#37662=DIRECTION ( 'NONE',  ( 1.000000000000000000, 2.042810365310287719E-14, 0.000000000000000000 ) ) ;
#37664=CONICAL_SURFACE ( 'NONE', #32053, 74.95140232871122521, 0.8777644062502172329 ) ;
#37682=LINE ( 'NONE', #53505, #42203 ) ;
#37685=ORIENTED_EDGE ( 'NONE', *, *, #14142, .T. ) ;
#37687=EDGE_LOOP ( 'NONE', ( #39569, #14486, #9855, #69448 ) ) ;
#37688=CARTESIAN_POINT ( 'NONE',  ( -46.06722295615789875, 46.37372919877053334, 43.58025477438756212 ) ) ;
#37692=DIRECTION ( 'NONE',  ( -1.000000000000000000, 0.000000000000000000, 0.000000000000000000 ) ) ;
#37701=LINE ( 'NONE', #59152, #65756 ) ;
#37702=EDGE_CURVE ( 'NONE', #11134, #39147, #52972, .T. ) ;
#37705=CARTESIAN_POINT ( 'NONE',  ( 0.000000000000000000, 0.000000000000000000, 41.38025477438755928 ) ) ;
#37712=VECTOR ( 'NONE', #24349, 1000.000000000000000 ) ;
#37722=VECTOR ( 'NONE', #61828, 1000.000000000000114 ) ;
#37728=CARTESIAN_POINT ( 'NONE',  ( -25.57361536219950082, 28.55671314637929470, 13.32819397642333037 ) ) ;
#37731=EDGE_CURVE ( 'NONE', #24493, #43605, #50017, .T. ) ;
#37733=ORIENTED_EDGE ( 'NONE', *, *, #31784, .F. ) ;
#37738=FACE_OUTER_BOUND ( 'NONE', #30474, .T. ) ;
#37739=DIRECTION ( 'NONE',  ( -0.7818314824680221431, -0.6234898018587431423, 0.000000000000000000 ) ) ;
#37741=ORIENTED_EDGE ( 'NONE', *, *, #8021, .T. ) ;
#37748=ORIENTED_EDGE ( 'NONE', *, *, #21433, .T. ) ;
#37750=AXIS2_PLACEMENT_3D ( 'NONE', #55685, #56038, #7854 ) ;
#37751=FACE_OUTER_BOUND ( 'NONE', #1825, .T. ) ;
#37757=ORIENTED_EDGE ( 'NONE', *, *, #13292, .T. ) ;
#37760=VECTOR ( 'NONE', #68711, 1000.000000000000000 ) ;
#37765=EDGE_CURVE ( 'NONE', #13447, #31009, #28927, .T. ) ;
#37768=AXIS2_PLACEMENT_3D ( 'NONE', #55418, #6884, #66357 ) ;
#37778=ORIENTED_EDGE ( 'NONE', *, *, #5063, .T. ) ;
#37779=CARTESIAN_POINT ( 'NONE',  ( -50.88541732109732862, -55.03078243218159571, 41.38025477438755928 ) ) ;
#37798=DIRECTION ( 'NONE',  ( 0.9839295885986321100, -0.1785568947986229116, 0.000000000000000000 ) ) ;
#37803=DIRECTION ( 'NONE',  ( -1.000000000000000000, 0.000000000000000000, 0.000000000000000000 ) ) ;
#37806=CARTESIAN_POINT ( 'NONE',  ( -51.82969867401435948, -54.20961478705483927, 43.58025477438756212 ) ) ;
#37808=AXIS2_PLACEMENT_3D ( 'NONE', #63223, #10097, #5163 ) ;
#37816=EDGE_CURVE ( 'NONE', #49197, #54158, #19393, .T. ) ;
#37817=DIRECTION ( 'NONE',  ( 1.000000000000000000, 0.000000000000000000, -0.000000000000000000 ) ) ;
#37823=CARTESIAN_POINT ( 'NONE',  ( -2.116120943111210906, -74.98056102853675497, 170.0000000000000000 ) ) ;
#37825=ORIENTED_EDGE ( 'NONE', *, *, #18455, .F. ) ;
#37828=DIRECTION ( 'NONE',  ( -1.000000000000000000, 0.000000000000000000, 0.000000000000000000 ) ) ;
#37831=DIRECTION ( 'NONE',  ( 1.000000000000000000, 0.000000000000000000, 0.000000000000000000 ) ) ;
#37837=ORIENTED_EDGE ( 'NONE', *, *, #33854, .T. ) ;
#37838=VERTEX_POINT ( 'NONE', #51421 ) ;
#37845=ORIENTED_EDGE ( 'NONE', *, *, #25598, .T. ) ;
#37854=EDGE_CURVE ( 'NONE', #16854, #21376, #51756, .T. ) ;
#37858=VERTEX_POINT ( 'NONE', #26410 ) ;
#37859=ORIENTED_EDGE ( 'NONE', *, *, #2786, .F. ) ;
#37864=CARTESIAN_POINT ( 'NONE',  ( -18.89790202299209199, 62.20684691518605547, 43.58025477438756923 ) ) ;
#37868=VECTOR ( 'NONE', #61920, 1000.000000000000227 ) ;
#37884=ADVANCED_FACE ( 'NONE', ( #42580 ), #6330, .F. ) ;
#37885=DIRECTION ( 'NONE',  ( -0.2225209339563042066, -0.9749279121818259508, 0.000000000000000000 ) ) ;
#37890=ORIENTED_EDGE ( 'NONE', *, *, #58215, .F. ) ;
#37891=DIRECTION ( 'NONE',  ( -1.000000000000000000, 0.000000000000000000, 0.000000000000000000 ) ) ;
#37904=VERTEX_POINT ( 'NONE', #53115 ) ;
#37905=CARTESIAN_POINT ( 'NONE',  ( 41.49663191311417165, -50.03028622612021792, 170.0000000000000000 ) ) ;
#37928=LINE ( 'NONE', #43539, #10502 ) ;
#37930=ORIENTED_EDGE ( 'NONE', *, *, #27151, .T. ) ;
#37938=ORIENTED_EDGE ( 'NONE', *, *, #65352, .T. ) ;
#37944=VECTOR ( 'NONE', #55388, 1000.000000000000000 ) ;
#37952=ORIENTED_EDGE ( 'NONE', *, *, #41161, .F. ) ;
#37953=DIRECTION ( 'NONE',  ( 1.000000000000000000, 0.000000000000000000, -0.000000000000000000 ) ) ;
#37963=DIRECTION ( 'NONE',  ( 0.000000000000000000, 0.000000000000000000, 1.000000000000000000 ) ) ;
#37969=FACE_OUTER_BOUND ( 'NONE', #20954, .T. ) ;
#37971=VERTEX_POINT ( 'NONE', #27787 ) ;
#37976=VECTOR ( 'NONE', #7609, 1000.000000000000000 ) ;
#37979=ORIENTED_EDGE ( 'NONE', *, *, #28759, .T. ) ;
#37989=B_SPLINE_CURVE_WITH_KNOTS ( 'NONE', 3,
 ( #38437, #64474, #48612, #59526 ),
 .UNSPECIFIED., .F., .F.,
 ( 4, 4 ),
 ( 0.1259919275528358362, 0.1829744153748746327 ),
 .UNSPECIFIED. ) ;
#37992=ORIENTED_EDGE ( 'NONE', *, *, #34796, .F. ) ;
#37998=VERTEX_POINT ( 'NONE', #5 ) ;
#38001=CARTESIAN_POINT ( 'NONE',  ( 32.64241757152704793, 7.194141534430333884, 6.893342931793793760 ) ) ;
#38003=AXIS2_PLACEMENT_3D ( 'NONE', #41294, #51839, #9277 ) ;
#38012=EDGE_CURVE ( 'NONE', #2785, #49177, #54146, .T. ) ;
#38013=FACE_OUTER_BOUND ( 'NONE', #4497, .T. ) ;
#38017=CARTESIAN_POINT ( 'NONE',  ( -51.84164840787185113, 39.21024726209461875, 170.0000000000000000 ) ) ;
#38019=CARTESIAN_POINT ( 'NONE',  ( 63.00000000000000000, 7.715274834628325378E-15, 40.82842712474622004 ) ) ;
#38023=VERTEX_POINT ( 'NONE', #43251 ) ;
#38026=CARTESIAN_POINT ( 'NONE',  ( -61.29635759142615115, 21.66977272663494958, 41.38025477438755928 ) ) ;
#38029=CARTESIAN_POINT ( 'NONE',  ( 35.54014968547473785, 66.04466488925542933, 0.000000000000000000 ) ) ;
#38032=DIRECTION ( 'NONE',  ( -1.000000000000000000, 0.000000000000000000, 0.000000000000000000 ) ) ;
#38034=FACE_OUTER_BOUND ( 'NONE', #68349, .T. ) ;
#38041=EDGE_CURVE ( 'NONE', #36640, #30444, #59437, .T. ) ;
#38050=VERTEX_POINT ( 'NONE', #22167 ) ;
#38051=EDGE_LOOP ( 'NONE', ( #11014, #55234, #62885, #3760 ) ) ;
#38078=LINE ( 'NONE', #12400, #31443 ) ;
#38083=DIRECTION ( 'NONE',  ( 0.7818314824680311359, -0.6234898018587319291, 0.000000000000000000 ) ) ;
#38089=CARTESIAN_POINT ( 'NONE',  ( 63.72039997003709999, 12.83396383267841401, 170.0000000000000000 ) ) ;
#38095=DIRECTION ( 'NONE',  ( 0.000000000000000000, -0.000000000000000000, -1.000000000000000000 ) ) ;
#38098=B_SPLINE_CURVE_WITH_KNOTS ( 'NONE', 3,
 ( #45499, #60988, #66630, #50439 ),
 .UNSPECIFIED., .F., .F.,
 ( 4, 4 ),
 ( 9.900409499167601085E-07, 0.05658314289920116785 ),
 .UNSPECIFIED. ) ;
#38100=CARTESIAN_POINT ( 'NONE',  ( 0.000000000000000000, 0.000000000000000000, 40.00000000000003553 ) ) ;
#38101=DIRECTION ( 'NONE',  ( -0.000000000000000000, -0.000000000000000000, -1.000000000000000000 ) ) ;
#38104=ADVANCED_FACE ( 'NONE', ( #54857 ), #23908, .T. ) ;
#38108=DIRECTION ( 'NONE',  ( 0.04486483035051862939, -0.9989930665413143673, -1.037707659396819425E-17 ) ) ;
#38112=CARTESIAN_POINT ( 'NONE',  ( 0.000000000000000000, 0.000000000000000000, 133.5802547743875550 ) ) ;
#38118=EDGE_CURVE ( 'NONE', #53998, #61117, #1372, .T. ) ;
#38120=LINE ( 'NONE', #54645, #40557 ) ;
#38124=EDGE_CURVE ( 'NONE', #8304, #3538, #14873, .T. ) ;
#38125=FACE_OUTER_BOUND ( 'NONE', #53777, .T. ) ;
#38129=ORIENTED_EDGE ( 'NONE', *, *, #52416, .T. ) ;
#38146=CARTESIAN_POINT ( 'NONE',  ( 0.000000000000000000, 0.000000000000000000, 170.0000000000000000 ) ) ;
#38147=PLANE ( 'NONE',  #31007 ) ;
#38151=DIRECTION ( 'NONE',  ( 0.7530714660036196273, -0.6579387259397027066, 0.000000000000000000 ) ) ;
#38153=DIRECTION ( 'NONE',  ( -1.000000000000000000, 0.000000000000000000, 0.000000000000000000 ) ) ;
#38155=AXIS2_PLACEMENT_3D ( 'NONE', #68135, #29797, #8351 ) ;
#38166=DIRECTION ( 'NONE',  ( 1.000000000000000000, 0.000000000000000000, 0.000000000000000000 ) ) ;
#38173=CARTESIAN_POINT ( 'NONE',  ( -74.58602291351368763, 7.967916035251061402, 170.0000000000000000 ) ) ;
#38177=ORIENTED_EDGE ( 'NONE', *, *, #41241, .T. ) ;
#38189=VECTOR ( 'NONE', #7949, 1000.000000000000000 ) ;
#38207=EDGE_CURVE ( 'NONE', #26073, #30106, #22709, .T. ) ;
#38228=ORIENTED_EDGE ( 'NONE', *, *, #60925, .F. ) ;
#38230=DIRECTION ( 'NONE',  ( 0.2225209339563184452, -0.9749279121818226201, 0.000000000000000000 ) ) ;
#38237=VERTEX_POINT ( 'NONE', #60141 ) ;
#38243=CARTESIAN_POINT ( 'NONE',  ( -68.06184294702700299, -31.38946074233465211, 41.38025477438755928 ) ) ;
#38250=DIRECTION ( 'NONE',  ( 1.000000000000000000, -4.174438572590588592E-14, 0.000000000000000000 ) ) ;
#38255=CARTESIAN_POINT ( 'NONE',  ( -29.70166638324966968, 57.83280658984257627, 170.0000000000000000 ) ) ;
#38258=DIRECTION ( 'NONE',  ( 0.000000000000000000, 0.000000000000000000, 1.000000000000000000 ) ) ;
#38261=ORIENTED_EDGE ( 'NONE', *, *, #65597, .T. ) ;
#38264=EDGE_CURVE ( 'NONE', #62436, #54950, #52697, .T. ) ;
#38265=CARTESIAN_POINT ( 'NONE',  ( 63.72039997003725631, -12.83396383267754182, 170.0000000000000000 ) ) ;
#38268=VECTOR ( 'NONE', #24505, 1000.000000000000114 ) ;
#38274=CARTESIAN_POINT ( 'NONE',  ( -39.87467016056562841, -12.30144018097216119, 13.79046412299627455 ) ) ;
#38279=ORIENTED_EDGE ( 'NONE', *, *, #9196, .F. ) ;
#38281=ORIENTED_EDGE ( 'NONE', *, *, #4240, .F. ) ;
#38282=VECTOR ( 'NONE', #54183, 1000.000000000000000 ) ;
#38291=LINE ( 'NONE', #5250, #32517 ) ;
#38298=LINE ( 'NONE', #49181, #50933 ) ;
#38301=CARTESIAN_POINT ( 'NONE',  ( -28.32746765835526048, 69.45586423092609607, 43.58025477438756212 ) ) ;
#38306=ORIENTED_EDGE ( 'NONE', *, *, #6580, .F. ) ;
#38308=CARTESIAN_POINT ( 'NONE',  ( -7.486743542469090684, -64.58150799671139453, 170.0000000000000000 ) ) ;
#38309=EDGE_LOOP ( 'NONE', ( #62646, #42555, #27903, #33429 ) ) ;
#38310=CARTESIAN_POINT ( 'NONE',  ( 29.86848256228606502, -58.14280299503694494, 41.38025477438755928 ) ) ;
#38317=VECTOR ( 'NONE', #40586, 999.9999999999998863 ) ;
#38321=ORIENTED_EDGE ( 'NONE', *, *, #58649, .F. ) ;
#38330=VECTOR ( 'NONE', #31370, 1000.000000000000000 ) ;
#38331=DIRECTION ( 'NONE',  ( 0.000000000000000000, 0.000000000000000000, 1.000000000000000000 ) ) ;
#38334=EDGE_CURVE ( 'NONE', #9333, #36739, #68547, .T. ) ;
#38335=DIRECTION ( 'NONE',  ( -0.000000000000000000, -0.000000000000000000, 1.000000000000000000 ) ) ;
#38354=PLANE ( 'NONE',  #48347 ) ;
#38357=DIRECTION ( 'NONE',  ( -0.5128992774058949156, -0.8584487936018728726, 5.102127870520020458E-18 ) ) ;
#38362=CARTESIAN_POINT ( 'NONE',  ( 70.60157554497457966, 25.16207943727196295, 41.38025477438755928 ) ) ;
#38373=DIRECTION ( 'NONE',  ( 0.000000000000000000, 0.000000000000000000, 1.000000000000000000 ) ) ;
#38377=EDGE_CURVE ( 'NONE', #52626, #48419, #63619, .T. ) ;
#38378=CARTESIAN_POINT ( 'NONE',  ( 55.14772863908675049, -34.40534879854660488, 40.00000000000003553 ) ) ;
#38388=DIRECTION ( 'NONE',  ( 1.000000000000000000, 0.000000000000000000, 0.000000000000000000 ) ) ;
#38398=ORIENTED_EDGE ( 'NONE', *, *, #2696, .T. ) ;
#38399=VERTEX_POINT ( 'NONE', #53041 ) ;
#38411=B_SPLINE_CURVE_WITH_KNOTS ( 'NONE', 3,
 ( #9529, #3552, #2868, #2522, #24680, #24337 ),
 .UNSPECIFIED., .F., .F.,
 ( 4, 2, 4 ),
 ( 1.095770181098114466E-06, 0.03239442681617710901, 0.06478775786217311206 ),
 .UNSPECIFIED. ) ;
#38412=DIRECTION ( 'NONE',  ( 0.3090169943749446757, 0.9510565162951544194, 0.000000000000000000 ) ) ;
#38419=ORIENTED_EDGE ( 'NONE', *, *, #380, .T. ) ;
#38431=CARTESIAN_POINT ( 'NONE',  ( 65.35403040894466642, 1.250000000000021982, 3.125053320693567160E-16 ) ) ;
#38433=VECTOR ( 'NONE', #40061, 1000.000000000000227 ) ;
#38434=CIRCLE ( 'NONE', #8117, 63.00000000000000000 ) ;
#38437=CARTESIAN_POINT ( 'NONE',  ( 0.1285234777254253835, 24.99966963213046611, 0.000000000000000000 ) ) ;
#38439=EDGE_CURVE ( 'NONE', #65498, #37573, #39591, .T. ) ;
#38441=EDGE_CURVE ( 'NONE', #22088, #24194, #17135, .T. ) ;
#38444=VERTEX_POINT ( 'NONE', #44927 ) ;
#38445=DIRECTION ( 'NONE',  ( -0.000000000000000000, -0.000000000000000000, -1.000000000000000000 ) ) ;
#38451=PLANE ( 'NONE',  #12309 ) ;
#38452=B_SPLINE_CURVE_WITH_KNOTS ( 'NONE', 3,
 ( #58632, #53351, #60021, #48759 ),
 .UNSPECIFIED., .F., .F.,
 ( 4, 4 ),
 ( 0.1259919275528360583, 0.1829744153748753543 ),
 .UNSPECIFIED. ) ;
#38462=CARTESIAN_POINT ( 'NONE',  ( 48.11816970607299027, -43.69944786993949748, 40.00000000000003553 ) ) ;
#38466=DIRECTION ( 'NONE',  ( -0.000000000000000000, -0.000000000000000000, 1.000000000000000000 ) ) ;
#38467=CARTESIAN_POINT ( 'NONE',  ( 0.000000000000000000, 0.000000000000000000, 170.0000000000000000 ) ) ;
#38474=PLANE ( 'NONE',  #46227 ) ;
#38481=ORIENTED_EDGE ( 'NONE', *, *, #39579, .F. ) ;
#38491=ORIENTED_EDGE ( 'NONE', *, *, #60364, .T. ) ;
#38499=DIRECTION ( 'NONE',  ( 1.000000000000000000, 0.000000000000000000, 0.000000000000000000 ) ) ;
#38517=DIRECTION ( 'NONE',  ( 1.000000000000000000, 0.000000000000000000, 0.000000000000000000 ) ) ;
#38526=VECTOR ( 'NONE', #16749, 1000.000000000000114 ) ;
#38536=ORIENTED_EDGE ( 'NONE', *, *, #15570, .F. ) ;
#38539=ORIENTED_EDGE ( 'NONE', *, *, #35980, .T. ) ;
#38547=CARTESIAN_POINT ( 'NONE',  ( -21.95369412746257254, 11.95973721106814835, 0.000000000000000000 ) ) ;
#38555=DIRECTION ( 'NONE',  ( -1.000000000000000000, 0.000000000000000000, 0.000000000000000000 ) ) ;
#38558=CARTESIAN_POINT ( 'NONE',  ( 0.000000000000000000, 0.000000000000000000, 170.0000000000000000 ) ) ;
#38572=CARTESIAN_POINT ( 'NONE',  ( -65.36598343705435354, 0.000000000000000000, 41.38025477438755928 ) ) ;
#38573=CONICAL_SURFACE ( 'NONE', #28485, 65.00000000000000000, 0.7853981633974497223 ) ;
#38575=VECTOR ( 'NONE', #28723, 1000.000000000000227 ) ;
#38577=CARTESIAN_POINT ( 'NONE',  ( -46.95151367498729655, -47.29862477898760176, 34.48241795236666718 ) ) ;
#38585=DIRECTION ( 'NONE',  ( 0.7227948638273978821, -0.6910626489868580968, 2.500042656554810340E-16 ) ) ;
#38587=CARTESIAN_POINT ( 'NONE',  ( 49.76301652092226391, -41.81676920493045202, 40.00000000000003553 ) ) ;
#38589=EDGE_CURVE ( 'NONE', #33967, #34424, #45630, .T. ) ;
#38591=EDGE_LOOP ( 'NONE', ( #32038, #27561, #5903, #45807 ) ) ;
#38596=DIRECTION ( 'NONE',  ( -0.000000000000000000, 0.000000000000000000, -1.000000000000000000 ) ) ;
#38604=DIRECTION ( 'NONE',  ( -1.000000000000000000, 0.000000000000000000, 0.000000000000000000 ) ) ;
#38605=ADVANCED_FACE ( 'NONE', ( #29793 ), #20494, .T. ) ;
#38620=CIRCLE ( 'NONE', #48735, 65.36598343705435354 ) ;
#38622=ORIENTED_EDGE ( 'NONE', *, *, #62766, .F. ) ;
#38627=ORIENTED_EDGE ( 'NONE', *, *, #48017, .T. ) ;
#38633=VECTOR ( 'NONE', #56608, 1000.000000000000114 ) ;
#38636=ORIENTED_EDGE ( 'NONE', *, *, #30665, .F. ) ;
#38651=ADVANCED_FACE ( 'NONE', ( #17683 ), #3681, .T. ) ;
#38661=PLANE ( 'NONE',  #38895 ) ;
#38666=DIRECTION ( 'NONE',  ( -0.000000000000000000, -0.000000000000000000, 1.000000000000000000 ) ) ;
#38667=ORIENTED_EDGE ( 'NONE', *, *, #35754, .F. ) ;
#38678=EDGE_LOOP ( 'NONE', ( #47343, #48973, #30945, #21754 ) ) ;
#38682=CARTESIAN_POINT ( 'NONE',  ( 0.000000000000000000, 0.000000000000000000, 41.38025477438755928 ) ) ;
#38689=VERTEX_POINT ( 'NONE', #44403 ) ;
#38695=DIRECTION ( 'NONE',  ( 1.000000000000000000, 0.000000000000000000, -0.000000000000000000 ) ) ;
#38699=CARTESIAN_POINT ( 'NONE',  ( -41.50537345350708307, 50.04124777106294886, 0.000000000000000000 ) ) ;
#38700=ADVANCED_FACE ( 'NONE', ( #31522 ), #45255, .T. ) ;
#38703=EDGE_CURVE ( 'NONE', #65008, #3292, #48022, .T. ) ;
#38707=EDGE_LOOP ( 'NONE', ( #46746, #57844, #6303, #68519 ) ) ;
#38709=VERTEX_POINT ( 'NONE', #52618 ) ;
#38711=CARTESIAN_POINT ( 'NONE',  ( 7.484861546145031852, 64.56761454192836425, 40.00000000000003553 ) ) ;
#38714=DIRECTION ( 'NONE',  ( 0.6910626489868580968, 0.7227948638273978821, -0.000000000000000000 ) ) ;
#38717=VECTOR ( 'NONE', #27810, 1000.000000000000000 ) ;
#38731=CARTESIAN_POINT ( 'NONE',  ( 51.00231672172485275, 42.89951318340155240, 34.48241795236666718 ) ) ;
#38732=CARTESIAN_POINT ( 'NONE',  ( 0.000000000000000000, 0.000000000000000000, 41.38025477438755928 ) ) ;
#38733=LINE ( 'NONE', #60177, #34418 ) ;
#38735=AXIS2_PLACEMENT_3D ( 'NONE', #49195, #58716, #6651 ) ;
#38742=ORIENTED_EDGE ( 'NONE', *, *, #60364, .F. ) ;
#38743=B_SPLINE_CURVE_WITH_KNOTS ( 'NONE', 3,
 ( #62261, #56641, #7770, #7427 ),
 .UNSPECIFIED., .F., .F.,
 ( 4, 4 ),
 ( 9.900409499076797036E-07, 0.05658314289920116785 ),
 .UNSPECIFIED. ) ;
#38744=EDGE_CURVE ( 'NONE', #937, #58062, #42069, .T. ) ;
#38753=CARTESIAN_POINT ( 'NONE',  ( -15.76129977463529563, 63.43731725181438463, 41.38025477438755928 ) ) ;
#38758=VERTEX_POINT ( 'NONE', #48352 ) ;
#38778=CIRCLE ( 'NONE', #66860, 65.00000000000000000 ) ;
#38782=CONICAL_SURFACE ( 'NONE', #15225, 74.95140232871122521, 0.8777644062502172329 ) ;
#38787=AXIS2_PLACEMENT_3D ( 'NONE', #53632, #59951, #33246 ) ;
#38792=VECTOR ( 'NONE', #4200, 1000.000000000000000 ) ;
#38800=ORIENTED_EDGE ( 'NONE', *, *, #10248, .F. ) ;
#38801=ORIENTED_EDGE ( 'NONE', *, *, #3364, .F. ) ;
#38802=CARTESIAN_POINT ( 'NONE',  ( 2.112947028648761272, 24.91054906769654664, 0.000000000000000000 ) ) ;
#38814=ORIENTED_EDGE ( 'NONE', *, *, #21285, .F. ) ;
#38831=CARTESIAN_POINT ( 'NONE',  ( 74.62299871641508275, -5.461138973197948943, 43.58025477438756923 ) ) ;
#38833=EDGE_LOOP ( 'NONE', ( #47826, #18051, #19539, #26595, #50482, #14247, #2061, #13967, #46435 ) ) ;
#38841=CYLINDRICAL_SURFACE ( 'NONE', #15752, 63.00000000000000000 ) ;
#38845=VECTOR ( 'NONE', #36389, 1000.000000000000114 ) ;
#38854=EDGE_CURVE ( 'NONE', #22781, #9333, #47696, .T. ) ;
#38858=VERTEX_POINT ( 'NONE', #61630 ) ;
#38866=DIRECTION ( 'NONE',  ( 0.000000000000000000, 0.000000000000000000, 1.000000000000000000 ) ) ;
#38867=ORIENTED_EDGE ( 'NONE', *, *, #56052, .T. ) ;
#38871=CARTESIAN_POINT ( 'NONE',  ( -8.712114576423529044, -23.56346432108879441, 3.061616997868437868E-16 ) ) ;
#38875=ORIENTED_EDGE ( 'NONE', *, *, #40667, .F. ) ;
#38885=CARTESIAN_POINT ( 'NONE',  ( 56.42997683260148278, -32.25922681454192542, 170.0000000000000000 ) ) ;
#38887=DIRECTION ( 'NONE',  ( 0.8345732537213079727, -0.5508969814520945363, 2.500042656554809847E-16 ) ) ;
#38888=AXIS2_PLACEMENT_3D ( 'NONE', #16785, #59351, #42818 ) ;
#38889=VECTOR ( 'NONE', #57654, 999.9999999999998863 ) ;
#38895=AXIS2_PLACEMENT_3D ( 'NONE', #60106, #44636, #66120 ) ;
#38902=EDGE_CURVE ( 'NONE', #61262, #51470, #42972, .T. ) ;
#38908=EDGE_CURVE ( 'NONE', #48854, #65404, #8165, .T. ) ;
#38912=ADVANCED_FACE ( 'NONE', ( #13784 ), #29970, .F. ) ;
#38913=CARTESIAN_POINT ( 'NONE',  ( -19.56458807131831890, -15.75959024859417390, 3.061616997868437868E-16 ) ) ;
#38915=VERTEX_POINT ( 'NONE', #51432 ) ;
#38920=DIRECTION ( 'NONE',  ( -0.000000000000000000, -0.000000000000000000, -1.000000000000000000 ) ) ;
#38924=CARTESIAN_POINT ( 'NONE',  ( 39.54205320694412507, -51.58901073076707888, 170.0000000000000000 ) ) ;
#38930=ORIENTED_EDGE ( 'NONE', *, *, #59049, .T. ) ;
#38954=ORIENTED_EDGE ( 'NONE', *, *, #54703, .T. ) ;
#38959=LINE ( 'NONE', #12566, #40034 ) ;
#38962=CARTESIAN_POINT ( 'NONE',  ( 56.42997683260104225, 32.25922681454270702, 170.0000000000000000 ) ) ;
#38965=DIRECTION ( 'NONE',  ( -1.000000000000000000, 0.000000000000000000, 0.000000000000000000 ) ) ;
#38972=ORIENTED_EDGE ( 'NONE', *, *, #64380, .F. ) ;
#38974=CARTESIAN_POINT ( 'NONE',  ( 0.000000000000000000, 0.000000000000000000, 0.000000000000000000 ) ) ;
#38980=VECTOR ( 'NONE', #6928, 1000.000000000000114 ) ;
#38983=DIRECTION ( 'NONE',  ( -0.000000000000000000, -0.000000000000000000, -1.000000000000000000 ) ) ;
#38991=AXIS2_PLACEMENT_3D ( 'NONE', #57163, #4040, #46947 ) ;
#38993=CARTESIAN_POINT ( 'NONE',  ( 32.06997139192709056, 56.95813133885486934, 41.38025477438755928 ) ) ;
#38997=ORIENTED_EDGE ( 'NONE', *, *, #41939, .T. ) ;
#39002=FACE_OUTER_BOUND ( 'NONE', #58351, .T. ) ;
#39013=CARTESIAN_POINT ( 'NONE',  ( 49.42891955109325153, 30.98851943060457614, 27.58472369397437163 ) ) ;
#39023=ORIENTED_EDGE ( 'NONE', *, *, #5625, .F. ) ;
#39025=FACE_OUTER_BOUND ( 'NONE', #52803, .T. ) ;
#39028=CARTESIAN_POINT ( 'NONE',  ( -24.51966494718099909, -5.470267094204724678, 0.000000000000000000 ) ) ;
#39031=CARTESIAN_POINT ( 'NONE',  ( 19.71799482800335923, -15.56722426018171035, 3.061616997868437868E-16 ) ) ;
#39036=DIRECTION ( 'NONE',  ( -1.000000000000000000, 0.000000000000000000, 0.000000000000000000 ) ) ;
#39038=VERTEX_POINT ( 'NONE', #11259 ) ;
#39045=DIRECTION ( 'NONE',  ( 1.000000000000000000, 0.000000000000000000, 0.000000000000000000 ) ) ;
#39060=ORIENTED_EDGE ( 'NONE', *, *, #34578, .F. ) ;
#39066=CARTESIAN_POINT ( 'NONE',  ( -9.964117946889912147, 64.24592483216710548, 170.0000000000000000 ) ) ;
#39070=EDGE_CURVE ( 'NONE', #26725, #9754, #52758, .T. ) ;
#39083=VECTOR ( 'NONE', #7565, 1000.000000000000114 ) ;
#39085=ORIENTED_EDGE ( 'NONE', *, *, #38439, .F. ) ;
#39088=AXIS2_PLACEMENT_3D ( 'NONE', #56360, #61299, #13796 ) ;
#39094=CARTESIAN_POINT ( 'NONE',  ( 10.73115448446713494, 22.57968829347503714, 0.000000000000000000 ) ) ;
#39096=DIRECTION ( 'NONE',  ( 1.000000000000000000, 0.000000000000000000, -0.000000000000000000 ) ) ;
#39097=CARTESIAN_POINT ( 'NONE',  ( 25.09133896793782981, -1.250000000000021982, 0.000000000000000000 ) ) ;
#39112=ADVANCED_FACE ( 'NONE', ( #64248 ), #53329, .T. ) ;
#39116=ORIENTED_EDGE ( 'NONE', *, *, #57723, .T. ) ;
#39119=LINE ( 'NONE', #33494, #43373 ) ;
#39121=CARTESIAN_POINT ( 'NONE',  ( 64.38365952014046911, -38.46744580544211800, 43.58025477438756212 ) ) ;
#39132=AXIS2_PLACEMENT_3D ( 'NONE', #36352, #13268, #42319 ) ;
#39134=CIRCLE ( 'NONE', #42481, 65.00000000000000000 ) ;
#39144=DIRECTION ( 'NONE',  ( 0.000000000000000000, 0.000000000000000000, 1.000000000000000000 ) ) ;
#39147=VERTEX_POINT ( 'NONE', #27648 ) ;
#39154=DIRECTION ( 'NONE',  ( -1.000000000000000000, 0.000000000000000000, 0.000000000000000000 ) ) ;
#39157=CARTESIAN_POINT ( 'NONE',  ( -84.49322488516129681, 0.000000000000000000, 43.58025477438756212 ) ) ;
#39165=DIRECTION ( 'NONE',  ( -1.000000000000000000, 0.000000000000000000, 0.000000000000000000 ) ) ;
#39166=EDGE_CURVE ( 'NONE', #11439, #38858, #14922, .T. ) ;
#39175=CARTESIAN_POINT ( 'NONE',  ( -44.26023579658873075, -48.10138582123835249, 41.38025477438755928 ) ) ;
#39181=CARTESIAN_POINT ( 'NONE',  ( -3.364862276287834408, -74.92447999059862696, 0.000000000000000000 ) ) ;
#39184=AXIS2_PLACEMENT_3D ( 'NONE', #28045, #49841, #61108 ) ;
#39195=ORIENTED_EDGE ( 'NONE', *, *, #7472, .T. ) ;
#39197=LINE ( 'NONE', #22654, #43945 ) ;
#39212=EDGE_LOOP ( 'NONE', ( #34876, #27499, #59433, #37979 ) ) ;
#39215=CARTESIAN_POINT ( 'NONE',  ( 4.549306917177319498, -73.43672186181514405, 133.5802547743875550 ) ) ;
#39219=PRODUCT_DEFINITION ( 'UNKNOWN', '', #4042, #59846 ) ;
#39220=ORIENTED_EDGE ( 'NONE', *, *, #65705, .T. ) ;
#39222=EDGE_CURVE ( 'NONE', #33172, #52626, #32248, .T. ) ;
#39224=ORIENTED_EDGE ( 'NONE', *, *, #60836, .T. ) ;
#39227=DIRECTION ( 'NONE',  ( 0.000000000000000000, 0.000000000000000000, 1.000000000000000000 ) ) ;
#39240=ORIENTED_EDGE ( 'NONE', *, *, #46454, .T. ) ;
#39246=PLANE ( 'NONE',  #56718 ) ;
#39248=ORIENTED_EDGE ( 'NONE', *, *, #60618, .F. ) ;
#39262=ORIENTED_EDGE ( 'NONE', *, *, #1043, .T. ) ;
#39266=AXIS2_PLACEMENT_3D ( 'NONE', #33374, #50236, #22802 ) ;
#39273=DIRECTION ( 'NONE',  ( -1.000000000000000000, 0.000000000000000000, 0.000000000000000000 ) ) ;
#39274=ORIENTED_EDGE ( 'NONE', *, *, #9797, .T. ) ;
#39279=CARTESIAN_POINT ( 'NONE',  ( 7.533997733928869067, 64.93035244659017735, 41.38025477438755928 ) ) ;
#39286=CARTESIAN_POINT ( 'NONE',  ( -37.04655464516766727, -53.85410457537912521, 43.58025477438756212 ) ) ;
#39326=ORIENTED_EDGE ( 'NONE', *, *, #68893, .T. ) ;
#39338=ORIENTED_EDGE ( 'NONE', *, *, #5474, .F. ) ;
#39339=ORIENTED_EDGE ( 'NONE', *, *, #8676, .T. ) ;
#39347=LINE ( 'NONE', #12614, #56417 ) ;
#39367=CARTESIAN_POINT ( 'NONE',  ( 0.1285234777257801275, -24.99966963213046611, 0.000000000000000000 ) ) ;
#39368=DIRECTION ( 'NONE',  ( 0.000000000000000000, -0.000000000000000000, -1.000000000000000000 ) ) ;
#39370=CARTESIAN_POINT ( 'NONE',  ( -59.89379335984659747, -45.06047301136921135, 41.38025477438755928 ) ) ;
#39377=CARTESIAN_POINT ( 'NONE',  ( 24.39800339187844003, 60.26242556095705538, 170.0000000000000000 ) ) ;
#39378=ORIENTED_EDGE ( 'NONE', *, *, #4681, .T. ) ;
#39384=EDGE_CURVE ( 'NONE', #22341, #14469, #21179, .T. ) ;
#39388=EDGE_LOOP ( 'NONE', ( #38814, #34914, #43692, #58320, #29668, #68818, #15484, #19334, #62132 ) ) ;
#39390=CARTESIAN_POINT ( 'NONE',  ( 0.000000000000000000, 0.000000000000000000, 0.000000000000000000 ) ) ;
#39391=PLANE ( 'NONE',  #12843 ) ;
#39393=EDGE_CURVE ( 'NONE', #50834, #28516, #67766, .T. ) ;
#39395=VERTEX_POINT ( 'NONE', #69360 ) ;
#39403=ORIENTED_EDGE ( 'NONE', *, *, #65884, .T. ) ;
#39405=CARTESIAN_POINT ( 'NONE',  ( 26.69682282325707945, 59.27986298182226221, 170.0000000000000000 ) ) ;
#39408=DIRECTION ( 'NONE',  ( -1.000000000000000000, 0.000000000000000000, 0.000000000000000000 ) ) ;
#39415=ORIENTED_EDGE ( 'NONE', *, *, #2380, .T. ) ;
#39418=VERTEX_POINT ( 'NONE', #37688 ) ;
#39422=CARTESIAN_POINT ( 'NONE',  ( 55.14772863908626732, 34.40534879854737227, 40.00000000000003553 ) ) ;
#39430=ORIENTED_EDGE ( 'NONE', *, *, #57130, .T. ) ;
#39439=VECTOR ( 'NONE', #33907, 1000.000000000000000 ) ;
#39446=ORIENTED_EDGE ( 'NONE', *, *, #60345, .T. ) ;
#39451=CIRCLE ( 'NONE', #60834, 10.00000000000000000 ) ;
#39460=CYLINDRICAL_SURFACE ( 'NONE', #19542, 65.36598343705435354 ) ;
#39469=CARTESIAN_POINT ( 'NONE',  ( 63.74253542338254164, 39.54050679744534591, 170.0000000000000000 ) ) ;
#39470=EDGE_CURVE ( 'NONE', #16594, #54975, #63749, .T. ) ;
#39472=CARTESIAN_POINT ( 'NONE',  ( 51.04335988554098691, -7.992588018875752098, 26.66469066592269144 ) ) ;
#39479=LINE ( 'NONE', #44765, #62232 ) ;
#39480=CARTESIAN_POINT ( 'NONE',  ( -54.64247910309503453, -38.15499993216875652, 34.48241795236666007 ) ) ;
#39483=EDGE_CURVE ( 'NONE', #38758, #4696, #4072, .T. ) ;
#39486=ORIENTED_EDGE ( 'NONE', *, *, #45037, .F. ) ;
#39491=ADVANCED_FACE ( 'NONE', ( #10265 ), #9356, .T. ) ;
#39495=CIRCLE ( 'NONE', #65349, 65.36598343705435354 ) ;
#39520=FACE_OUTER_BOUND ( 'NONE', #28580, .T. ) ;
#39523=CARTESIAN_POINT ( 'NONE',  ( -64.97888516016269023, -7.103257987406330187, 3.125053320693569132E-16 ) ) ;
#39530=ORIENTED_EDGE ( 'NONE', *, *, #28336, .F. ) ;
#39531=ORIENTED_EDGE ( 'NONE', *, *, #61218, .F. ) ;
#39533=ADVANCED_FACE ( 'NONE', ( #68665 ), #31798, .T. ) ;
#39534=CARTESIAN_POINT ( 'NONE',  ( 53.32245423372616244, -37.19594572654634845, 43.58025477438756923 ) ) ;
#39541=LINE ( 'NONE', #17018, #58813 ) ;
#39543=CARTESIAN_POINT ( 'NONE',  ( 21.27121078971695312, -61.42097029141944375, 170.0000000000000000 ) ) ;
#39546=DIRECTION ( 'NONE',  ( -0.5877852522924802425, 0.8090169943749422332, 0.000000000000000000 ) ) ;
#39547=CARTESIAN_POINT ( 'NONE',  ( 6.381648866512449558, -37.79907605652034874, 13.32819299319722539 ) ) ;
#39552=DIRECTION ( 'NONE',  ( 0.000000000000000000, 0.000000000000000000, 1.000000000000000000 ) ) ;
#39563=CARTESIAN_POINT ( 'NONE',  ( 73.57152302639913444, -14.62167909564502821, 170.0000000000000000 ) ) ;
#39565=VERTEX_POINT ( 'NONE', #12008 ) ;
#39568=VERTEX_POINT ( 'NONE', #33815 ) ;
#39569=ORIENTED_EDGE ( 'NONE', *, *, #27350, .T. ) ;
#39574=LINE ( 'NONE', #1586, #37944 ) ;
#39579=EDGE_CURVE ( 'NONE', #49951, #59826, #23272, .T. ) ;
#39580=FACE_OUTER_BOUND ( 'NONE', #47638, .T. ) ;
#39583=ORIENTED_EDGE ( 'NONE', *, *, #55831, .F. ) ;
#39584=CARTESIAN_POINT ( 'NONE',  ( 13.56909401489539846, -65.06753427964257241, 73.58025477438755502 ) ) ;
#39589=EDGE_LOOP ( 'NONE', ( #32501, #27177, #132, #44797, #4144, #53380, #60108, #16741, #6904 ) ) ;
#39591=CIRCLE ( 'NONE', #9259, 74.95140232871122521 ) ;
#39592=EDGE_LOOP ( 'NONE', ( #8998, #16237, #4608, #30060 ) ) ;
#39596=CARTESIAN_POINT ( 'NONE',  ( 29.86848256228520526, 58.14280299503737837, 3.125053320693577513E-16 ) ) ;
#39616=ORIENTED_EDGE ( 'NONE', *, *, #68784, .F. ) ;
#39636=ADVANCED_FACE ( 'NONE', ( #54904 ), #28174, .T. ) ;
#39644=DIRECTION ( 'NONE',  ( 0.3090169943749446757, 0.9510565162951544194, 0.000000000000000000 ) ) ;
#39649=VECTOR ( 'NONE', #27320, 1000.000000000000114 ) ;
#39651=CIRCLE ( 'NONE', #35134, 25.12245591505646303 ) ;
#39661=EDGE_CURVE ( 'NONE', #57513, #2845, #41891, .T. ) ;
#39668=EDGE_LOOP ( 'NONE', ( #63063, #17368, #852, #64172 ) ) ;
#39678=FACE_OUTER_BOUND ( 'NONE', #64159, .T. ) ;
#39685=CARTESIAN_POINT ( 'NONE',  ( -64.18058723658640474, -10.37664328995274055, 170.0000000000000000 ) ) ;
#39690=CIRCLE ( 'NONE', #68892, 24.99999999999985434 ) ;
#39691=EDGE_CURVE ( 'NONE', #35756, #66616, #6018, .T. ) ;
#39692=CARTESIAN_POINT ( 'NONE',  ( 55.61348889667009132, -50.24791103897046440, 41.38025477438755928 ) ) ;
#39695=ORIENTED_EDGE ( 'NONE', *, *, #22422, .F. ) ;
#39701=VECTOR ( 'NONE', #25465, 1000.000000000000000 ) ;
#39707=AXIS2_PLACEMENT_3D ( 'NONE', #46183, #68007, #2592 ) ;
#39710=ORIENTED_EDGE ( 'NONE', *, *, #19321, .T. ) ;
#39714=DIRECTION ( 'NONE',  ( -0.8090169943749422332, -0.5877852522924802425, 0.000000000000000000 ) ) ;
#39716=DIRECTION ( 'NONE',  ( -0.9959742939952384022, -0.08963930890344089242, 0.000000000000000000 ) ) ;
#39718=LINE ( 'NONE', #30211, #50223 ) ;
#39723=EDGE_CURVE ( 'NONE', #67765, #16637, #68843, .T. ) ;
#39732=PLANE ( 'NONE',  #66532 ) ;
#39734=CARTESIAN_POINT ( 'NONE',  ( -17.90772993695113868, 72.84144224619130625, 170.0000000000000000 ) ) ;
#39736=CARTESIAN_POINT ( 'NONE',  ( -65.20298343242131978, -4.613322252418188718, 41.38025477438755928 ) ) ;
#39740=DIRECTION ( 'NONE',  ( -0.5508969814520944253, -0.8345732537213078617, 0.000000000000000000 ) ) ;
#39752=VECTOR ( 'NONE', #36598, 1000.000000000000114 ) ;
#39753=ORIENTED_EDGE ( 'NONE', *, *, #12621, .T. ) ;
#39781=CARTESIAN_POINT ( 'NONE',  ( -35.66505483122875120, 56.29927536160143831, 34.48241795236666007 ) ) ;
#39783=ORIENTED_EDGE ( 'NONE', *, *, #55416, .F. ) ;
#39801=DIRECTION ( 'NONE',  ( -0.000000000000000000, -0.000000000000000000, 1.000000000000000000 ) ) ;
#39808=EDGE_LOOP ( 'NONE', ( #38281, #10191, #10365, #47507, #19731, #36761, #32736, #54689, #46650 ) ) ;
#39813=CARTESIAN_POINT ( 'NONE',  ( 0.000000000000000000, 0.000000000000000000, 40.00000000000003553 ) ) ;
#39816=DIRECTION ( 'NONE',  ( 0.2225209339563042066, 0.9749279121818259508, -0.000000000000000000 ) ) ;
#39832=EDGE_LOOP ( 'NONE', ( #52393, #54427, #3004, #64580 ) ) ;
#39836=CIRCLE ( 'NONE', #57815, 74.95140232871122521 ) ;
#39844=DIRECTION ( 'NONE',  ( -0.000000000000000000, -0.000000000000000000, -1.000000000000000000 ) ) ;
#39858=EDGE_CURVE ( 'NONE', #67200, #33912, #38298, .T. ) ;
#39873=CYLINDRICAL_SURFACE ( 'NONE', #39707, 63.00000000000000000 ) ;
#39897=CARTESIAN_POINT ( 'NONE',  ( 73.51344971438143716, -14.61114034329455258, 41.38025477438755928 ) ) ;
#39907=DIRECTION ( 'NONE',  ( -1.000000000000000000, 0.000000000000000000, 0.000000000000000000 ) ) ;
#39910=ORIENTED_EDGE ( 'NONE', *, *, #38902, .T. ) ;
#39922=EDGE_CURVE ( 'NONE', #13679, #1714, #54459, .T. ) ;
#39933=VECTOR ( 'NONE', #51382, 999.9999999999998863 ) ;
#39934=AXIS2_PLACEMENT_3D ( 'NONE', #64900, #43076, #38153 ) ;
#39935=ORIENTED_EDGE ( 'NONE', *, *, #29471, .T. ) ;
#39941=CARTESIAN_POINT ( 'NONE',  ( -31.90315521289150524, 56.64813493366005304, 170.0000000000000000 ) ) ;
#39942=ADVANCED_FACE ( 'NONE', ( #44627 ), #59401, .F. ) ;
#39949=EDGE_LOOP ( 'NONE', ( #9483, #69491, #28259, #65574 ) ) ;
#39950=ADVANCED_FACE ( 'NONE', ( #27044 ), #11552, .T. ) ;
#39953=CARTESIAN_POINT ( 'NONE',  ( -28.30427060690108476, 69.40159203110296460, 41.38025477438755928 ) ) ;
#39960=ORIENTED_EDGE ( 'NONE', *, *, #12616, .T. ) ;
#39970=EDGE_CURVE ( 'NONE', #66476, #23762, #24577, .T. ) ;
#39972=CARTESIAN_POINT ( 'NONE',  ( -14.79841479960619921, -20.14961338137257840, 0.000000000000000000 ) ) ;
#39974=CARTESIAN_POINT ( 'NONE',  ( 4.590321433069001422, -24.57496590315233931, 0.000000000000000000 ) ) ;
#39975=CARTESIAN_POINT ( 'NONE',  ( 25.09133896793783336, 1.250000000000021982, 3.061616997868437868E-16 ) ) ;
#39977=ADVANCED_FACE ( 'NONE', ( #12622 ), #55521, .T. ) ;
#39978=CARTESIAN_POINT ( 'NONE',  ( -16.68907004672388084, 73.11959341363670717, 43.58025477438756212 ) ) ;
#39995=CARTESIAN_POINT ( 'NONE',  ( 36.64089410029568228, 65.45232906116417837, 170.0000000000000000 ) ) ;
#39996=VECTOR ( 'NONE', #11207, 1000.000000000000000 ) ;
#40002=CARTESIAN_POINT ( 'NONE',  ( -4.164416015345870470, 64.86646004871185767, 170.0000000000000000 ) ) ;
#40010=EDGE_CURVE ( 'NONE', #28072, #16942, #34123, .T. ) ;
#40012=CARTESIAN_POINT ( 'NONE',  ( 73.79471914489722906, 13.39176710989777952, 0.000000000000000000 ) ) ;
#40013=VERTEX_POINT ( 'NONE', #19625 ) ;
#40022=B_SPLINE_CURVE_WITH_KNOTS ( 'NONE', 3,
 ( #63870, #53639, #16365, #535 ),
 .UNSPECIFIED., .F., .F.,
 ( 4, 4 ),
 ( 0.1259919275528361138, 0.1829744153748753543 ),
 .UNSPECIFIED. ) ;
#40032=EDGE_LOOP ( 'NONE', ( #33576, #63367, #44175, #65950 ) ) ;
#40034=VECTOR ( 'NONE', #44918, 1000.000000000000000 ) ;
#40036=CARTESIAN_POINT ( 'NONE',  ( 48.79594039481688128, -16.97828768250229103, 26.66469066592269144 ) ) ;
#40040=CARTESIAN_POINT ( 'NONE',  ( 69.77839676787858991, 27.52340539440040956, 170.0000000000000000 ) ) ;
#40044=ORIENTED_EDGE ( 'NONE', *, *, #39166, .T. ) ;
#40049=CARTESIAN_POINT ( 'NONE',  ( 0.000000000000000000, 0.000000000000000000, 2.000000000000001776 ) ) ;
#40056=EDGE_CURVE ( 'NONE', #12081, #21604, #8172, .T. ) ;
#40061=DIRECTION ( 'NONE',  ( -0.9959742939952382912, -0.08963930890344087854, 0.000000000000000000 ) ) ;
#40062=FACE_OUTER_BOUND ( 'NONE', #64147, .T. ) ;
#40070=EDGE_LOOP ( 'NONE', ( #31217, #60907, #14773, #40203, #47344, #68678, #44904, #58827, #62545 ) ) ;
#40091=CONICAL_SURFACE ( 'NONE', #25490, 74.95140232871122521, 0.8777644062502172329 ) ;
#40097=ORIENTED_EDGE ( 'NONE', *, *, #38124, .F. ) ;
#40098=VECTOR ( 'NONE', #5233, 1000.000000000000000 ) ;
#40100=ADVANCED_FACE ( 'NONE', ( #47048 ), #4488, .T. ) ;
#40106=DIRECTION ( 'NONE',  ( -0.000000000000000000, -0.000000000000000000, 1.000000000000000000 ) ) ;
#40107=ORIENTED_EDGE ( 'NONE', *, *, #14208, .T. ) ;
#40116=VERTEX_POINT ( 'NONE', #15730 ) ;
#40119=ADVANCED_FACE ( 'NONE', ( #63233 ), #38573, .T. ) ;
#40124=DIRECTION ( 'NONE',  ( 0.8090169943749506709, -0.5877852522924686962, 0.000000000000000000 ) ) ;
#40127=CARTESIAN_POINT ( 'NONE',  ( 0.000000000000000000, 0.000000000000000000, 73.58025477438756923 ) ) ;
#40135=CARTESIAN_POINT ( 'NONE',  ( 0.000000000000000000, 0.000000000000000000, 43.58025477438756212 ) ) ;
#40145=DIRECTION ( 'NONE',  ( 2.477416674922665047E-16, -3.355888904727913208E-17, 1.000000000000000000 ) ) ;
#40149=FACE_OUTER_BOUND ( 'NONE', #15597, .T. ) ;
#40162=ORIENTED_EDGE ( 'NONE', *, *, #35882, .F. ) ;
#40163=DIRECTION ( 'NONE',  ( 0.1342332658176667304, -0.9909497617679331460, 0.000000000000000000 ) ) ;
#40164=DIRECTION ( 'NONE',  ( -0.000000000000000000, -0.000000000000000000, -1.000000000000000000 ) ) ;
#40171=ORIENTED_EDGE ( 'NONE', *, *, #66424, .F. ) ;
#40176=AXIS2_PLACEMENT_3D ( 'NONE', #65673, #22400, #6571 ) ;
#40197=ADVANCED_FACE ( 'NONE', ( #49102 ), #43124, .T. ) ;
#40203=ORIENTED_EDGE ( 'NONE', *, *, #61493, .T. ) ;
#40205=CARTESIAN_POINT ( 'NONE',  ( 74.94097818310312675, -1.250000000000021760, 41.38025477438755928 ) ) ;
#40209=DIRECTION ( 'NONE',  ( 0.000000000000000000, 0.000000000000000000, 1.000000000000000000 ) ) ;
#40214=ORIENTED_EDGE ( 'NONE', *, *, #35580, .T. ) ;
#40215=DIRECTION ( 'NONE',  ( 0.000000000000000000, 0.000000000000000000, 1.000000000000000000 ) ) ;
#40222=DIRECTION ( 'NONE',  ( 1.000000000000000000, 0.000000000000000000, 0.000000000000000000 ) ) ;
#40228=VERTEX_POINT ( 'NONE', #6910 ) ;
#40231=CARTESIAN_POINT ( 'NONE',  ( -17.90772993695113868, 72.84144224619130625, 170.0000000000000000 ) ) ;
#40235=UNCERTAINTY_MEASURE_WITH_UNIT (LENGTH_MEASURE( 1.000000000000000082E-05 ), #47079, 'distance_accuracy_value', 'NONE');
#40246=CARTESIAN_POINT ( 'NONE',  ( 64.52696037203368462, -10.43950074664762262, 3.125053320693559764E-16 ) ) ;
#40254=CARTESIAN_POINT ( 'NONE',  ( -24.75616454008743972, 3.483147608716851806, 0.000000000000000000 ) ) ;
#40255=LINE ( 'NONE', #50114, #65912 ) ;
#40258=EDGE_CURVE ( 'NONE', #43258, #54206, #14888, .T. ) ;
#40259=ORIENTED_EDGE ( 'NONE', *, *, #28925, .F. ) ;
#40264=ORIENTED_EDGE ( 'NONE', *, *, #6902, .F. ) ;
#40265=LINE ( 'NONE', #56435, #58144 ) ;
#40276=VECTOR ( 'NONE', #10822, 1000.000000000000000 ) ;
#40289=CARTESIAN_POINT ( 'NONE',  ( 26.69682282325707945, 59.27986298182226221, 170.0000000000000000 ) ) ;
#40300=CARTESIAN_POINT ( 'NONE',  ( -30.62628708973392122, 68.47330165179127448, 43.58025477438756923 ) ) ;
#40334=EDGE_LOOP ( 'NONE', ( #18726, #27477, #41702, #11099, #28631, #4228, #51302, #830, #67447 ) ) ;
#40343=ORIENTED_EDGE ( 'NONE', *, *, #28772, .T. ) ;
#40344=LINE ( 'NONE', #57905, #66054 ) ;
#40350=CARTESIAN_POINT ( 'NONE',  ( 15.68296563925498965, 63.09411298019766434, 3.061616997868437868E-16 ) ) ;
#40356=EDGE_CURVE ( 'NONE', #11740, #20027, #26274, .T. ) ;
#40359=ORIENTED_EDGE ( 'NONE', *, *, #20532, .F. ) ;
#40363=EDGE_CURVE ( 'NONE', #242, #57624, #38620, .T. ) ;
#40366=ORIENTED_EDGE ( 'NONE', *, *, #13583, .T. ) ;
#40373=VERTEX_POINT ( 'NONE', #52916 ) ;
#40374=CIRCLE ( 'NONE', #53802, 65.00000000000000000 ) ;
#40375=ORIENTED_EDGE ( 'NONE', *, *, #26205, .F. ) ;
#40391=CARTESIAN_POINT ( 'NONE',  ( -1.683356153842345604, -65.34430428700412108, 3.125053320693568639E-16 ) ) ;
#40394=CIRCLE ( 'NONE', #10063, 74.95140232871122521 ) ;
#40399=DIRECTION ( 'NONE',  ( -0.000000000000000000, 0.000000000000000000, -1.000000000000000000 ) ) ;
#40407=EDGE_CURVE ( 'NONE', #21788, #671, #30447, .T. ) ;
#40409=ORIENTED_EDGE ( 'NONE', *, *, #38441, .F. ) ;
#40410=AXIS2_PLACEMENT_3D ( 'NONE', #58698, #32673, #43206 ) ;
#40414=ORIENTED_EDGE ( 'NONE', *, *, #67158, .T. ) ;
#40419=EDGE_CURVE ( 'NONE', #59923, #4530, #41355, .T. ) ;
#40421=EDGE_CURVE ( 'NONE', #23357, #68876, #14952, .T. ) ;
#40428=LINE ( 'NONE', #45359, #7208 ) ;
#40430=CARTESIAN_POINT ( 'NONE',  ( -12.71198166530320606, 21.52685583500265665, 0.000000000000000000 ) ) ;
#40436=DIRECTION ( 'NONE',  ( 1.000000000000000000, 8.881784197001252323E-16, 0.000000000000000000 ) ) ;
#40444=EDGE_CURVE ( 'NONE', #937, #42059, #66768, .T. ) ;
#40448=CARTESIAN_POINT ( 'NONE',  ( -74.75133697335800775, -5.472689625387135770, 41.38025477438755928 ) ) ;
#40486=CARTESIAN_POINT ( 'NONE',  ( -23.03840347525633447, -9.707315041312391202, 0.000000000000000000 ) ) ;
#40488=EDGE_CURVE ( 'NONE', #59075, #48432, #12456, .T. ) ;
#40493=DIRECTION ( 'NONE',  ( -2.377681859532289471E-16, -7.725556675377533209E-17, 1.000000000000000000 ) ) ;
#40503=CARTESIAN_POINT ( 'NONE',  ( -55.15976438495108169, -34.41253982194112382, 41.38025477438755928 ) ) ;
#40512=ORIENTED_EDGE ( 'NONE', *, *, #56797, .T. ) ;
#40522=ORIENTED_EDGE ( 'NONE', *, *, #29394, .T. ) ;
#40527=EDGE_CURVE ( 'NONE', #49554, #61455, #5654, .T. ) ;
#40557=VECTOR ( 'NONE', #6107, 1000.000000000000114 ) ;
#40564=ORIENTED_EDGE ( 'NONE', *, *, #45878, .F. ) ;
#40569=ADVANCED_FACE ( 'NONE', ( #51134 ), #67326, .T. ) ;
#40571=EDGE_CURVE ( 'NONE', #62016, #49197, #58136, .T. ) ;
#40580=CARTESIAN_POINT ( 'NONE',  ( -33.17493578845583357, -47.98885271304750688, 27.58472315868180402 ) ) ;
#40585=EDGE_CURVE ( 'NONE', #66914, #24361, #4930, .T. ) ;
#40586=DIRECTION ( 'NONE',  ( 0.3513748240813435175, -0.9362348706397369824, 0.000000000000000000 ) ) ;
#40603=ORIENTED_EDGE ( 'NONE', *, *, #28408, .F. ) ;
#40612=ORIENTED_EDGE ( 'NONE', *, *, #6580, .T. ) ;
#40613=LINE ( 'NONE', #39584, #60417 ) ;
#40617=LINE ( 'NONE', #24800, #6239 ) ;
#40623=DIRECTION ( 'NONE',  ( -0.000000000000000000, -0.000000000000000000, -1.000000000000000000 ) ) ;
#40624=CARTESIAN_POINT ( 'NONE',  ( -65.00000000000000000, 0.000000000000000000, 40.00000000000003553 ) ) ;
#40632=AXIS2_PLACEMENT_3D ( 'NONE', #58400, #47845, #11250 ) ;
#40635=CARTESIAN_POINT ( 'NONE',  ( 0.000000000000000000, 0.000000000000000000, 170.0000000000000000 ) ) ;
#40636=VECTOR ( 'NONE', #18900, 1000.000000000000227 ) ;
#40643=ADVANCED_FACE ( 'NONE', ( #26124 ), #30368, .T. ) ;
#40654=ADVANCED_FACE ( 'NONE', ( #68012 ), #24752, .T. ) ;
#40660=CARTESIAN_POINT ( 'NONE',  ( 65.78600691410852619, -10.66798400760944610, 34.48241823980617227 ) ) ;
#40667=EDGE_CURVE ( 'NONE', #4738, #67298, #19819, .T. ) ;
#40673=LINE ( 'NONE', #52608, #44502 ) ;
#40678=VERTEX_POINT ( 'NONE', #52166 ) ;
#40679=CARTESIAN_POINT ( 'NONE',  ( 10.65073780419444738, -36.82468537061276237, 13.32819397642333215 ) ) ;
#40680=ORIENTED_EDGE ( 'NONE', *, *, #7793, .T. ) ;
#40684=CARTESIAN_POINT ( 'NONE',  ( 0.000000000000000000, 0.000000000000000000, 0.000000000000000000 ) ) ;
#40687=LINE ( 'NONE', #47011, #19602 ) ;
#40703=EDGE_CURVE ( 'NONE', #24540, #57182, #68592, .T. ) ;
#40709=DIRECTION ( 'NONE',  ( 1.000000000000000000, 0.000000000000000000, -0.000000000000000000 ) ) ;
#40715=DIRECTION ( 'NONE',  ( -1.000000000000000000, 0.000000000000000000, 0.000000000000000000 ) ) ;
#40717=CARTESIAN_POINT ( 'NONE',  ( -30.62628708973294422, -68.47330165179167238, 43.58025477438756212 ) ) ;
#40718=CARTESIAN_POINT ( 'NONE',  ( -29.55217180659046861, 15.61897120291162011, 6.893343212288939981 ) ) ;
#40720=ADVANCED_FACE ( 'NONE', ( #9608 ), #31071, .T. ) ;
#40726=EDGE_CURVE ( 'NONE', #21605, #16881, #22837, .T. ) ;
#40732=FACE_OUTER_BOUND ( 'NONE', #67618, .T. ) ;
#40738=EDGE_CURVE ( 'NONE', #42819, #2042, #33347, .T. ) ;
#40748=CARTESIAN_POINT ( 'NONE',  ( 73.51344971438143716, -14.61114034329455258, 41.38025477438755928 ) ) ;
#40751=AXIS2_PLACEMENT_3D ( 'NONE', #17831, #60391, #22752 ) ;
#40753=EDGE_CURVE ( 'NONE', #57123, #24108, #52638, .T. ) ;
#40772=DIRECTION ( 'NONE',  ( -1.000000000000000000, 0.000000000000000000, 0.000000000000000000 ) ) ;
#40775=EDGE_LOOP ( 'NONE', ( #59422, #36000, #18207, #35183, #21344, #42938, #47275, #18115, #57556 ) ) ;
#40788=ORIENTED_EDGE ( 'NONE', *, *, #16743, .F. ) ;
#40796=CYLINDRICAL_SURFACE ( 'NONE', #2197, 65.00000000000000000 ) ;
#40800=ORIENTED_EDGE ( 'NONE', *, *, #26128, .F. ) ;
#40804=CIRCLE ( 'NONE', #12743, 25.12245591505646303 ) ;
#40808=CARTESIAN_POINT ( 'NONE',  ( 0.000000000000000000, 0.000000000000000000, 41.38025477438755928 ) ) ;
#40820=EDGE_CURVE ( 'NONE', #7248, #13790, #11933, .T. ) ;
#40821=DIRECTION ( 'NONE',  ( 0.8584487936018655452, 0.5128992774059070170, 0.000000000000000000 ) ) ;
#40830=VERTEX_POINT ( 'NONE', #39028 ) ;
#40833=CARTESIAN_POINT ( 'NONE',  ( 33.18066468065407548, -39.60239314731277460, 26.66469066592268433 ) ) ;
#40834=CARTESIAN_POINT ( 'NONE',  ( 24.36509522348982060, 70.94296747916789059, 133.5802547743875550 ) ) ;
#40840=ADVANCED_FACE ( 'NONE', ( #40062 ), #49548, .T. ) ;
#40846=VECTOR ( 'NONE', #17006, 1000.000000000000114 ) ;
#40864=EDGE_LOOP ( 'NONE', ( #35298, #37422, #8292, #39486 ) ) ;
#40867=CARTESIAN_POINT ( 'NONE',  ( -39.55079474733699385, 51.59997227570983824, 3.061616997868437868E-16 ) ) ;
#40868=FACE_OUTER_BOUND ( 'NONE', #29698, .T. ) ;
#40869=ORIENTED_EDGE ( 'NONE', *, *, #31510, .F. ) ;
#40870=VERTEX_POINT ( 'NONE', #62202 ) ;
#40871=CARTESIAN_POINT ( 'NONE',  ( -29.87147652227456263, -74.98256102853682137, 73.58025477438756923 ) ) ;
#40872=DIRECTION ( 'NONE',  ( -1.000000000000000000, 0.000000000000000000, 0.000000000000000000 ) ) ;
#40874=ORIENTED_EDGE ( 'NONE', *, *, #33892, .F. ) ;
#40878=AXIS2_PLACEMENT_3D ( 'NONE', #2110, #23901, #49922 ) ;
#40883=VERTEX_POINT ( 'NONE', #14373 ) ;
#40886=CIRCLE ( 'NONE', #56609, 74.95140232871122521 ) ;
#40890=DIRECTION ( 'NONE',  ( -0.000000000000000000, -0.000000000000000000, -1.000000000000000000 ) ) ;
#40892=VECTOR ( 'NONE', #10869, 1000.000000000000114 ) ;
#40894=EDGE_CURVE ( 'NONE', #17237, #44366, #44984, .T. ) ;
#40903=ADVANCED_FACE ( 'NONE', ( #34457 ), #8403, .T. ) ;
#40906=EDGE_CURVE ( 'NONE', #3054, #28358, #68521, .T. ) ;
#40919=CARTESIAN_POINT ( 'NONE',  ( -4.613603609465520172, 74.86839895266042788, 170.0000000000000000 ) ) ;
#40926=DIRECTION ( 'NONE',  ( -0.9959742939952397345, 0.08963930890342655666, 0.000000000000000000 ) ) ;
#40931=CARTESIAN_POINT ( 'NONE',  ( -37.75148796553126829, -54.92203290797168336, 34.48241795236666007 ) ) ;
#40932=EDGE_CURVE ( 'NONE', #65795, #27252, #20608, .T. ) ;
#40942=CARTESIAN_POINT ( 'NONE',  ( 50.03867889673373526, -42.05760816978109773, 43.58025477438756212 ) ) ;
#40946=CARTESIAN_POINT ( 'NONE',  ( -9.744241279244798548, 37.07486149500672923, 13.32819299319724138 ) ) ;
#40949=ORIENTED_EDGE ( 'NONE', *, *, #47466, .T. ) ;
#40952=DIRECTION ( 'NONE',  ( 0.000000000000000000, 0.000000000000000000, 1.000000000000000000 ) ) ;
#40954=DIRECTION ( 'NONE',  ( -0.8584487936018728726, 0.5128992774058949156, 0.000000000000000000 ) ) ;
#40959=LINE ( 'NONE', #36028, #27559 ) ;
#40967=EDGE_CURVE ( 'NONE', #58719, #41480, #16069, .T. ) ;
#40969=LINE ( 'NONE', #35703, #34937 ) ;
#40971=DIRECTION ( 'NONE',  ( -1.000000000000000000, 0.000000000000000000, 0.000000000000000000 ) ) ;
#40972=VERTEX_POINT ( 'NONE', #64622 ) ;
#40974=ORIENTED_EDGE ( 'NONE', *, *, #55129, .F. ) ;
#40987=ORIENTED_EDGE ( 'NONE', *, *, #9797, .F. ) ;
#40989=DIRECTION ( 'NONE',  ( 1.000000000000000000, 0.000000000000000000, 0.000000000000000000 ) ) ;
#40995=AXIS2_PLACEMENT_3D ( 'NONE', #55066, #34685, #23435 ) ;
#41036=ORIENTED_EDGE ( 'NONE', *, *, #14894, .F. ) ;
#41043=VECTOR ( 'NONE', #48402, 1000.000000000000000 ) ;
#41050=ADVANCED_FACE ( 'NONE', ( #43152 ), #12552, .T. ) ;
#41052=ORIENTED_EDGE ( 'NONE', *, *, #3924, .F. ) ;
#41058=ORIENTED_EDGE ( 'NONE', *, *, #25273, .F. ) ;
#41059=FACE_OUTER_BOUND ( 'NONE', #49235, .T. ) ;
#41063=ORIENTED_EDGE ( 'NONE', *, *, #39166, .F. ) ;
#41074=CARTESIAN_POINT ( 'NONE',  ( -23.73638277007033182, -7.847555861075553807, 0.000000000000000000 ) ) ;
#41077=LINE ( 'NONE', #3106, #15782 ) ;
#41081=VERTEX_POINT ( 'NONE', #18872 ) ;
#41084=CIRCLE ( 'NONE', #6264, 65.36598343705435354 ) ;
#41089=FACE_OUTER_BOUND ( 'NONE', #46551, .T. ) ;
#41091=VECTOR ( 'NONE', #40821, 1000.000000000000114 ) ;
#41095=CARTESIAN_POINT ( 'NONE',  ( -2.116120943112233643, 74.98056102853672655, 170.0000000000000000 ) ) ;
#41099=CARTESIAN_POINT ( 'NONE',  ( 0.000000000000000000, 0.000000000000000000, 170.0000000000000000 ) ) ;
#41101=CARTESIAN_POINT ( 'NONE',  ( -13.24252603915608617, 63.63674649211943546, 73.58025477438756923 ) ) ;
#41106=CIRCLE ( 'NONE', #56876, 65.36598343705435354 ) ;
#41107=DIRECTION ( 'NONE',  ( -1.000000000000000000, 0.000000000000000000, 0.000000000000000000 ) ) ;
#41112=DIRECTION ( 'NONE',  ( 0.000000000000000000, -5.102127870520020458E-18, -1.000000000000000000 ) ) ;
#41116=ORIENTED_EDGE ( 'NONE', *, *, #23269, .T. ) ;
#41121=DIRECTION ( 'NONE',  ( 0.000000000000000000, 0.000000000000000000, 1.000000000000000000 ) ) ;
#41122=VERTEX_POINT ( 'NONE', #2353 ) ;
#41132=AXIS2_PLACEMENT_3D ( 'NONE', #40, #37328, #69348 ) ;
#41142=AXIS2_PLACEMENT_3D ( 'NONE', #1571, #23039, #39907 ) ;
#41149=DIRECTION ( 'NONE',  ( 0.5508969814521065267, -0.8345732537212999791, 0.000000000000000000 ) ) ;
#41151=CARTESIAN_POINT ( 'NONE',  ( 0.000000000000000000, 0.000000000000000000, 43.58025477438756212 ) ) ;
#41152=CARTESIAN_POINT ( 'NONE',  ( -9.964117946889912147, 64.24592483216710548, 41.38025477438755928 ) ) ;
#41155=EDGE_CURVE ( 'NONE', #7827, #53047, #21734, .T. ) ;
#41156=ORIENTED_EDGE ( 'NONE', *, *, #69324, .F. ) ;
#41161=EDGE_CURVE ( 'NONE', #52056, #30082, #45789, .T. ) ;
#41183=ORIENTED_EDGE ( 'NONE', *, *, #34739, .F. ) ;
#41188=VECTOR ( 'NONE', #68910, 1000.000000000000000 ) ;
#41190=VECTOR ( 'NONE', #33830, 1000.000000000000000 ) ;
#41194=ORIENTED_EDGE ( 'NONE', *, *, #46995, .T. ) ;
#41198=ADVANCED_FACE ( 'NONE', ( #50873 ), #29766, .F. ) ;
#41202=CIRCLE ( 'NONE', #62547, 65.36598343705435354 ) ;
#41223=VERTEX_POINT ( 'NONE', #62471 ) ;
#41233=LINE ( 'NONE', #62694, #65130 ) ;
#41235=ADVANCED_FACE ( 'NONE', ( #15317 ), #52595, .T. ) ;
#41236=LINE ( 'NONE', #35953, #68030 ) ;
#41238=DIRECTION ( 'NONE',  ( -0.6910626489868685329, 0.7227948638273878901, 0.000000000000000000 ) ) ;
#41240=EDGE_CURVE ( 'NONE', #59777, #21604, #1511, .T. ) ;
#41241=EDGE_CURVE ( 'NONE', #37573, #38237, #50902, .T. ) ;
#41262=CARTESIAN_POINT ( 'NONE',  ( 0.000000000000000000, 0.000000000000000000, 0.000000000000000000 ) ) ;
#41272=DIRECTION ( 'NONE',  ( 0.000000000000000000, 0.000000000000000000, 1.000000000000000000 ) ) ;
#41284=CARTESIAN_POINT ( 'NONE',  ( -36.84489839129265931, -53.54860840895233309, 170.0000000000000000 ) ) ;
#41285=AXIS2_PLACEMENT_3D ( 'NONE', #7092, #28552, #66213 ) ;
#41292=CARTESIAN_POINT ( 'NONE',  ( -1.740765657700568569, -66.62262621221535142, 34.48241823979275722 ) ) ;
#41294=CARTESIAN_POINT ( 'NONE',  ( 0.000000000000000000, 0.000000000000000000, 41.38025477438755928 ) ) ;
#41299=ADVANCED_FACE ( 'NONE', ( #515 ), #46979, .F. ) ;
#41301=ORIENTED_EDGE ( 'NONE', *, *, #28692, .T. ) ;
#41304=DIRECTION ( 'NONE',  ( 1.000000000000000000, 0.000000000000000000, -0.000000000000000000 ) ) ;
#41307=EDGE_LOOP ( 'NONE', ( #13669, #2024, #24210, #54844 ) ) ;
#41309=EDGE_CURVE ( 'NONE', #69425, #43897, #1215, .T. ) ;
#41336=CARTESIAN_POINT ( 'NONE',  ( 75.00000000000000000, -1.250000000000021982, 43.58025477438756212 ) ) ;
#41355=LINE ( 'NONE', #63841, #52130 ) ;
#41383=EDGE_LOOP ( 'NONE', ( #63028, #48361, #44936, #43376 ) ) ;
#41387=VERTEX_POINT ( 'NONE', #12465 ) ;
#41388=VECTOR ( 'NONE', #14886, 1000.000000000000000 ) ;
#41399=DIRECTION ( 'NONE',  ( -0.000000000000000000, -0.000000000000000000, -1.000000000000000000 ) ) ;
#41400=CARTESIAN_POINT ( 'NONE',  ( 0.000000000000000000, 0.000000000000000000, 0.000000000000000000 ) ) ;
#41419=ORIENTED_EDGE ( 'NONE', *, *, #39691, .F. ) ;
#41420=EDGE_LOOP ( 'NONE', ( #46697, #12378, #8077, #51788 ) ) ;
#41428=DIRECTION ( 'NONE',  ( -0.000000000000000000, -0.000000000000000000, -1.000000000000000000 ) ) ;
#41436=CARTESIAN_POINT ( 'NONE',  ( 55.65793654284683356, -50.28674377798225237, 170.0000000000000000 ) ) ;
#41438=CIRCLE ( 'NONE', #27918, 65.36598343705435354 ) ;
#41443=EDGE_CURVE ( 'NONE', #67530, #53526, #50019, .T. ) ;
#41445=ORIENTED_EDGE ( 'NONE', *, *, #68368, .F. ) ;
#41450=DIRECTION ( 'NONE',  ( 0.000000000000000000, 0.000000000000000000, 1.000000000000000000 ) ) ;
#41459=EDGE_LOOP ( 'NONE', ( #4612, #56200, #55871, #21163, #47325, #55785, #36369, #55057, #54023 ) ) ;
#41471=EDGE_CURVE ( 'NONE', #32990, #8876, #20852, .T. ) ;
#41473=EDGE_LOOP ( 'NONE', ( #37938, #15208, #44991, #66325 ) ) ;
#41480=VERTEX_POINT ( 'NONE', #19828 ) ;
#41487=ORIENTED_EDGE ( 'NONE', *, *, #25901, .T. ) ;
#41490=VECTOR ( 'NONE', #20515, 1000.000000000000114 ) ;
#41492=ORIENTED_EDGE ( 'NONE', *, *, #58079, .F. ) ;
#41493=FACE_OUTER_BOUND ( 'NONE', #37161, .T. ) ;
#41514=DIRECTION ( 'NONE',  ( -0.6234898018587431423, 0.7818314824680220321, 0.000000000000000000 ) ) ;
#41523=VERTEX_POINT ( 'NONE', #20165 ) ;
#41530=EDGE_CURVE ( 'NONE', #38858, #62756, #27158, .T. ) ;
#41545=ORIENTED_EDGE ( 'NONE', *, *, #12069, .T. ) ;
#41550=DIRECTION ( 'NONE',  ( 1.000000000000000000, 0.000000000000000000, 0.000000000000000000 ) ) ;
#41555=DIRECTION ( 'NONE',  ( -0.2225209339563184452, 0.9749279121818226201, 0.000000000000000000 ) ) ;
#41567=ORIENTED_EDGE ( 'NONE', *, *, #24952, .F. ) ;
#41575=VECTOR ( 'NONE', #30154, 1000.000000000000000 ) ;
#41576=DIRECTION ( 'NONE',  ( 0.6910626489868580968, 0.7227948638273978821, 0.000000000000000000 ) ) ;
#41579=PLANE ( 'NONE',  #17700 ) ;
#41584=CARTESIAN_POINT ( 'NONE',  ( 0.000000000000000000, 0.000000000000000000, 41.38025477438755928 ) ) ;
#41585=CARTESIAN_POINT ( 'NONE',  ( 55.46196446482079523, 34.59309596431375411, 41.38025477438755928 ) ) ;
#41592=DIRECTION ( 'NONE',  ( 1.000000000000000000, 0.000000000000000000, 0.000000000000000000 ) ) ;
#41596=DIRECTION ( 'NONE',  ( -0.000000000000000000, -0.000000000000000000, -1.000000000000000000 ) ) ;
#41609=CARTESIAN_POINT ( 'NONE',  ( 63.72039997003709288, 12.83396383267841223, 40.00000000000003553 ) ) ;
#41610=CARTESIAN_POINT ( 'NONE',  ( -47.07758031033817048, 21.28397246211312321, 26.66469066592268788 ) ) ;
#41613=EDGE_CURVE ( 'NONE', #55532, #67200, #34199, .T. ) ;
#41617=DIRECTION ( 'NONE',  ( -0.000000000000000000, -0.000000000000000000, -1.000000000000000000 ) ) ;
#41620=CARTESIAN_POINT ( 'NONE',  ( 0.000000000000000000, 0.000000000000000000, 170.0000000000000000 ) ) ;
#41624=CARTESIAN_POINT ( 'NONE',  ( 0.000000000000000000, 0.000000000000000000, 40.00000000000003553 ) ) ;
#41626=VERTEX_POINT ( 'NONE', #2525 ) ;
#41627=CARTESIAN_POINT ( 'NONE',  ( -12.71191156098292652, -50.07707454696033977, 26.66469104408690782 ) ) ;
#41634=EDGE_CURVE ( 'NONE', #43258, #44455, #30747, .T. ) ;
#41638=DIRECTION ( 'NONE',  ( 3.356887510711447811E-18, -3.842266915190389043E-18, -1.000000000000000000 ) ) ;
#41640=VERTEX_POINT ( 'NONE', #51061 ) ;
#41682=CARTESIAN_POINT ( 'NONE',  ( 10.06749493632500503, -74.32123213259498584, 0.000000000000000000 ) ) ;
#41702=ORIENTED_EDGE ( 'NONE', *, *, #10735, .F. ) ;
#41717=CARTESIAN_POINT ( 'NONE',  ( -31.08850300935970878, -49.36609570479362930, 27.58472369403420643 ) ) ;
#41720=ADVANCED_FACE ( 'NONE', ( #55993 ), #39460, .T. ) ;
#41721=DIRECTION ( 'NONE',  ( -1.000000000000000000, 0.000000000000000000, 0.000000000000000000 ) ) ;
#41722=ORIENTED_EDGE ( 'NONE', *, *, #13678, .T. ) ;
#41749=CARTESIAN_POINT ( 'NONE',  ( 0.000000000000000000, 0.000000000000000000, 43.58025477438756212 ) ) ;
#41754=AXIS2_PLACEMENT_3D ( 'NONE', #36255, #57711, #31663 ) ;
#41764=LINE ( 'NONE', #37166, #69405 ) ;
#41773=ORIENTED_EDGE ( 'NONE', *, *, #67158, .F. ) ;
#41777=DIRECTION ( 'NONE',  ( -0.7530714660036195163, 0.6579387259397027066, 0.000000000000000000 ) ) ;
#41779=DIRECTION ( 'NONE',  ( -1.000000000000000000, 0.000000000000000000, 0.000000000000000000 ) ) ;
#41785=CARTESIAN_POINT ( 'NONE',  ( -38.27142476814294980, 2.189438101076349508, 13.32819299319723783 ) ) ;
#41788=VERTEX_POINT ( 'NONE', #53794 ) ;
#41799=AXIS2_PLACEMENT_3D ( 'NONE', #28484, #50630, #56255 ) ;
#41815=AXIS2_PLACEMENT_3D ( 'NONE', #10497, #42173, #15449 ) ;
#41835=DIRECTION ( 'NONE',  ( 0.000000000000000000, 0.000000000000000000, 1.000000000000000000 ) ) ;
#41839=ORIENTED_EDGE ( 'NONE', *, *, #31315, .T. ) ;
#41841=ADVANCED_FACE ( 'NONE', ( #66139 ), #61185, .T. ) ;
#41845=ORIENTED_EDGE ( 'NONE', *, *, #44211, .F. ) ;
#41851=VECTOR ( 'NONE', #47352, 1000.000000000000000 ) ;
#41854=B_SPLINE_CURVE_WITH_KNOTS ( 'NONE', 3,
 ( #6577, #5192, #27322, #65323 ),
 .UNSPECIFIED., .F., .F.,
 ( 4, 4 ),
 ( 0.1259919275528364746, 0.1829744153748763535 ),
 .UNSPECIFIED. ) ;
#41871=CARTESIAN_POINT ( 'NONE',  ( 21.96921518829188358, 71.65937688154191676, 41.38025477438755928 ) ) ;
#41878=CARTESIAN_POINT ( 'NONE',  ( 6.526941389886392386, -24.13294503563501436, 0.000000000000000000 ) ) ;
#41882=ORIENTED_EDGE ( 'NONE', *, *, #29262, .F. ) ;
#41886=CARTESIAN_POINT ( 'NONE',  ( -63.33140416796853600, 16.18162651919394435, 3.125053320693577513E-16 ) ) ;
#41888=ORIENTED_EDGE ( 'NONE', *, *, #50896, .F. ) ;
#41891=CIRCLE ( 'NONE', #11536, 65.00000000000000000 ) ;
#41916=DIRECTION ( 'NONE',  ( -0.000000000000000000, -0.000000000000000000, -1.000000000000000000 ) ) ;
#41917=LINE ( 'NONE', #35615, #38330 ) ;
#41920=ORIENTED_EDGE ( 'NONE', *, *, #35980, .F. ) ;
#41921=EDGE_CURVE ( 'NONE', #26782, #24447, #22608, .T. ) ;
#41926=CARTESIAN_POINT ( 'NONE',  ( 0.000000000000000000, 0.000000000000000000, 170.0000000000000000 ) ) ;
#41934=AXIS2_PLACEMENT_3D ( 'NONE', #26560, #63504, #36780 ) ;
#41939=EDGE_CURVE ( 'NONE', #9754, #27253, #60594, .T. ) ;
#41941=AXIS2_PLACEMENT_3D ( 'NONE', #32342, #53769, #37953 ) ;
#41950=DIRECTION ( 'NONE',  ( -0.9195277725514489076, -0.3930250316539278810, 2.500042656554810340E-16 ) ) ;
#41957=DIRECTION ( 'NONE',  ( 0.000000000000000000, 0.000000000000000000, -1.000000000000000000 ) ) ;
#41958=VECTOR ( 'NONE', #54503, 1000.000000000000000 ) ;
#41975=LINE ( 'NONE', #14891, #3796 ) ;
#41979=DIRECTION ( 'NONE',  ( -0.000000000000000000, -0.000000000000000000, -1.000000000000000000 ) ) ;
#41983=VECTOR ( 'NONE', #66588, 1000.000000000000000 ) ;
#42001=CIRCLE ( 'NONE', #11665, 65.00000000000000000 ) ;
#42012=LINE ( 'NONE', #14927, #14294 ) ;
#42019=VERTEX_POINT ( 'NONE', #44412 ) ;
#42020=ORIENTED_EDGE ( 'NONE', *, *, #53796, .T. ) ;
#42021=EDGE_CURVE ( 'NONE', #1085, #60210, #49856, .T. ) ;
#42028=LINE ( 'NONE', #26198, #7916 ) ;
#42032=EDGE_LOOP ( 'NONE', ( #23725, #68131, #23094, #29199 ) ) ;
#42049=CARTESIAN_POINT ( 'NONE',  ( -18.89790202299212396, 62.20684691518604836, 170.0000000000000000 ) ) ;
#42055=LINE ( 'NONE', #69119, #28440 ) ;
#42059=VERTEX_POINT ( 'NONE', #38802 ) ;
#42069=LINE ( 'NONE', #5470, #49706 ) ;
#42073=CARTESIAN_POINT ( 'NONE',  ( 0.000000000000000000, 0.000000000000000000, 41.38025477438755928 ) ) ;
#42074=EDGE_LOOP ( 'NONE', ( #49111, #41052, #25451, #61879, #1401, #12509, #25031, #14689, #44001 ) ) ;
#42075=EDGE_CURVE ( 'NONE', #48718, #45468, #67863, .T. ) ;
#42079=ORIENTED_EDGE ( 'NONE', *, *, #54238, .T. ) ;
#42081=VECTOR ( 'NONE', #46767, 1000.000000000000000 ) ;
#42082=DIRECTION ( 'NONE',  ( -0.9959742939952397345, 0.08963930890342655666, 0.000000000000000000 ) ) ;
#42084=EDGE_CURVE ( 'NONE', #68160, #43082, #19414, .T. ) ;
#42089=CARTESIAN_POINT ( 'NONE',  ( -1.666933348991701536, -64.97862212458817055, 170.0000000000000000 ) ) ;
#42091=ORIENTED_EDGE ( 'NONE', *, *, #52263, .F. ) ;
#42092=FACE_OUTER_BOUND ( 'NONE', #27097, .T. ) ;
#42093=VECTOR ( 'NONE', #61799, 1000.000000000000000 ) ;
#42098=CARTESIAN_POINT ( 'NONE',  ( -39.87466933223296905, 12.30143995236625365, 13.79046340968177553 ) ) ;
#42104=CARTESIAN_POINT ( 'NONE',  ( 0.000000000000000000, 0.000000000000000000, 0.000000000000000000 ) ) ;
#42106=EDGE_CURVE ( 'NONE', #30275, #64382, #34915, .T. ) ;
#42112=CARTESIAN_POINT ( 'NONE',  ( -28.32746765835429414, -69.45586423092650818, 43.58025477438756923 ) ) ;
#42126=ORIENTED_EDGE ( 'NONE', *, *, #53887, .T. ) ;
#42127=CARTESIAN_POINT ( 'NONE',  ( -65.36598343705435354, 0.000000000000000000, 41.38025477438755928 ) ) ;
#42128=ORIENTED_EDGE ( 'NONE', *, *, #6664, .F. ) ;
#42129=CARTESIAN_POINT ( 'NONE',  ( 0.000000000000000000, 0.000000000000000000, 41.38025477438755928 ) ) ;
#42138=AXIS2_PLACEMENT_3D ( 'NONE', #68984, #36992, #36653 ) ;
#42141=DIRECTION ( 'NONE',  ( -0.000000000000000000, -0.000000000000000000, 1.000000000000000000 ) ) ;
#42144=ORIENTED_EDGE ( 'NONE', *, *, #47643, .T. ) ;
#42145=CIRCLE ( 'NONE', #34325, 25.12245591505646303 ) ;
#42152=EDGE_CURVE ( 'NONE', #24493, #35316, #63370, .T. ) ;
#42153=CONICAL_SURFACE ( 'NONE', #43277, 65.00000000000000000, 0.7853981633974497223 ) ;
#42160=DIRECTION ( 'NONE',  ( 2.312964634635743450E-16, -0.000000000000000000, 1.000000000000000000 ) ) ;
#42167=EDGE_CURVE ( 'NONE', #27278, #4891, #55576, .T. ) ;
#42171=ORIENTED_EDGE ( 'NONE', *, *, #12155, .F. ) ;
#42173=DIRECTION ( 'NONE',  ( -0.000000000000000000, -0.000000000000000000, 1.000000000000000000 ) ) ;
#42174=CARTESIAN_POINT ( 'NONE',  ( 41.72486082342823011, -50.31647622756197080, 41.38025477438755928 ) ) ;
#42175=ORIENTED_EDGE ( 'NONE', *, *, #54938, .T. ) ;
#42185=ORIENTED_EDGE ( 'NONE', *, *, #9396, .T. ) ;
#42191=CIRCLE ( 'NONE', #17485, 65.00000000000000000 ) ;
#42196=EDGE_CURVE ( 'NONE', #56134, #5466, #367, .T. ) ;
#42200=LINE ( 'NONE', #54099, #39996 ) ;
#42201=ORIENTED_EDGE ( 'NONE', *, *, #65296, .F. ) ;
#42203=VECTOR ( 'NONE', #47888, 1000.000000000000000 ) ;
#42204=ORIENTED_EDGE ( 'NONE', *, *, #47643, .F. ) ;
#42221=CARTESIAN_POINT ( 'NONE',  ( -65.00200000000002376, -1.250000000000021094, 170.0000000000000000 ) ) ;
#42233=CONICAL_SURFACE ( 'NONE', #65854, 74.95140232871122521, 0.8777644062502172329 ) ;
#42235=ORIENTED_EDGE ( 'NONE', *, *, #38908, .F. ) ;
#42241=DIRECTION ( 'NONE',  ( 0.7818314824680311359, -0.6234898018587319291, 0.000000000000000000 ) ) ;
#42248=DIRECTION ( 'NONE',  ( -0.04486483035051862939, 0.9989930665413143673, 0.000000000000000000 ) ) ;
#42250=AXIS2_PLACEMENT_3D ( 'NONE', #52474, #4299, #31032 ) ;
#42255=CIRCLE ( 'NONE', #11915, 65.00000000000000000 ) ;
#42259=ORIENTED_EDGE ( 'NONE', *, *, #38377, .T. ) ;
#42277=DIRECTION ( 'NONE',  ( 1.000000000000000000, 0.000000000000000000, -0.000000000000000000 ) ) ;
#42292=PLANE ( 'NONE',  #52430 ) ;
#42300=ORIENTED_EDGE ( 'NONE', *, *, #46855, .F. ) ;
#42301=ORIENTED_EDGE ( 'NONE', *, *, #19951, .F. ) ;
#42302=CARTESIAN_POINT ( 'NONE',  ( 37.47470330837911945, 8.071072105428767074, 13.32819299319724138 ) ) ;
#42304=DIRECTION ( 'NONE',  ( -0.2225209339563042066, -0.9749279121818259508, 0.000000000000000000 ) ) ;
#42309=CARTESIAN_POINT ( 'NONE',  ( 0.000000000000000000, 0.000000000000000000, 0.000000000000000000 ) ) ;
#42312=CARTESIAN_POINT ( 'NONE',  ( 53.32245423372562243, 37.19594572654712294, 41.38025477438755928 ) ) ;
#42315=CARTESIAN_POINT ( 'NONE',  ( 26.12852347772543737, 100.0000000000000000, 77.58025477438755502 ) ) ;
#42319=DIRECTION ( 'NONE',  ( 0.000000000000000000, -0.000000000000000000, -1.000000000000000000 ) ) ;
#42329=ORIENTED_EDGE ( 'NONE', *, *, #66197, .F. ) ;
#42336=ORIENTED_EDGE ( 'NONE', *, *, #42152, .T. ) ;
#42337=VECTOR ( 'NONE', #55103, 1000.000000000000227 ) ;
#42352=CARTESIAN_POINT ( 'NONE',  ( 19.21260300789856501, 55.08522701181888692, 27.58472315868180402 ) ) ;
#42353=ORIENTED_EDGE ( 'NONE', *, *, #40421, .T. ) ;
#42359=DIRECTION ( 'NONE',  ( -1.000000000000000000, 0.000000000000000000, 0.000000000000000000 ) ) ;
#42365=VERTEX_POINT ( 'NONE', #1691 ) ;
#42371=AXIS2_PLACEMENT_3D ( 'NONE', #7812, #61271, #2531 ) ;
#42372=CARTESIAN_POINT ( 'NONE',  ( 17.98081503251148661, 17.36923402935782690, 0.000000000000000000 ) ) ;
#42373=CARTESIAN_POINT ( 'NONE',  ( 18.89356949897824123, 62.19351277735709260, 170.0000000000000000 ) ) ;
#42375=ORIENTED_EDGE ( 'NONE', *, *, #68898, .F. ) ;
#42382=VECTOR ( 'NONE', #53789, 999.9999999999998863 ) ;
#42383=LINE ( 'NONE', #32180, #59565 ) ;
#42385=VERTEX_POINT ( 'NONE', #54081 ) ;
#42386=CIRCLE ( 'NONE', #21058, 65.36598343705435354 ) ;
#42390=DIRECTION ( 'NONE',  ( -0.000000000000000000, 0.000000000000000000, -1.000000000000000000 ) ) ;
#42392=DIRECTION ( 'NONE',  ( -1.000000000000000000, 0.000000000000000000, 0.000000000000000000 ) ) ;
#42403=DIRECTION ( 'NONE',  ( -1.000000000000000000, 0.000000000000000000, 0.000000000000000000 ) ) ;
#42413=EDGE_CURVE ( 'NONE', #47971, #30365, #11885, .T. ) ;
#42418=EDGE_CURVE ( 'NONE', #39568, #68560, #45401, .T. ) ;
#42421=CARTESIAN_POINT ( 'NONE',  ( -28.32746765835526048, 69.45586423092609607, 170.0000000000000000 ) ) ;
#42424=ORIENTED_EDGE ( 'NONE', *, *, #6338, .F. ) ;
#42427=DIRECTION ( 'NONE',  ( 1.282270072030906146E-16, -2.146158602472679632E-16, 1.000000000000000000 ) ) ;
#42434=AXIS2_PLACEMENT_3D ( 'NONE', #26167, #21235, #42682 ) ;
#42439=CARTESIAN_POINT ( 'NONE',  ( 64.52696037203355672, 10.43950074664854633, 43.58025477438756212 ) ) ;
#42440=CARTESIAN_POINT ( 'NONE',  ( 0.000000000000000000, 0.000000000000000000, 41.38025477438755928 ) ) ;
#42455=ORIENTED_EDGE ( 'NONE', *, *, #936, .T. ) ;
#42456=DIRECTION ( 'NONE',  ( -1.000000000000000000, 0.000000000000000000, 0.000000000000000000 ) ) ;
#42460=CARTESIAN_POINT ( 'NONE',  ( -48.12872802574267439, 43.70867239603707333, 170.0000000000000000 ) ) ;
#42469=VERTEX_POINT ( 'NONE', #50569 ) ;
#42481=AXIS2_PLACEMENT_3D ( 'NONE', #35500, #68208, #14041 ) ;
#42490=DIRECTION ( 'NONE',  ( -0.2225209339563184452, 0.9749279121818226201, 0.000000000000000000 ) ) ;
#42492=CARTESIAN_POINT ( 'NONE',  ( -15.76129977463530274, 63.43731725181437042, 3.125053320693565680E-16 ) ) ;
#42511=DIRECTION ( 'NONE',  ( 0.000000000000000000, 0.000000000000000000, 1.000000000000000000 ) ) ;
#42525=ORIENTED_EDGE ( 'NONE', *, *, #39384, .T. ) ;
#42526=CIRCLE ( 'NONE', #17837, 65.00000000000000000 ) ;
#42530=CARTESIAN_POINT ( 'NONE',  ( -17.54261607806453327, -37.86253161628560093, 13.79046340968177908 ) ) ;
#42537=DIRECTION ( 'NONE',  ( 2.477416674922665047E-16, -3.355888904727913208E-17, 1.000000000000000000 ) ) ;
#42539=EDGE_LOOP ( 'NONE', ( #23839, #45837, #60138, #58764 ) ) ;
#42541=CYLINDRICAL_SURFACE ( 'NONE', #44242, 65.00000000000000000 ) ;
#42546=DIRECTION ( 'NONE',  ( 0.000000000000000000, 0.000000000000000000, 1.000000000000000000 ) ) ;
#42555=ORIENTED_EDGE ( 'NONE', *, *, #6969, .F. ) ;
#42556=ADVANCED_FACE ( 'NONE', ( #41059 ), #9052, .T. ) ;
#42558=CARTESIAN_POINT ( 'NONE',  ( -61.41100614348687969, 43.07262267896646790, 170.0000000000000000 ) ) ;
#42559=DIRECTION ( 'NONE',  ( 0.000000000000000000, 0.000000000000000000, 1.000000000000000000 ) ) ;
#42562=CARTESIAN_POINT ( 'NONE',  ( -39.55079474733702227, 51.59997227570980982, 170.0000000000000000 ) ) ;
#42571=DIRECTION ( 'NONE',  ( 1.000000000000000000, 0.000000000000000000, 0.000000000000000000 ) ) ;
#42573=LINE ( 'NONE', #31673, #56514 ) ;
#42574=DIRECTION ( 'NONE',  ( -0.000000000000000000, -0.000000000000000000, -1.000000000000000000 ) ) ;
#42579=DIRECTION ( 'NONE',  ( -0.9959742939952382912, -0.08963930890344087854, 0.000000000000000000 ) ) ;
#42580=FACE_OUTER_BOUND ( 'NONE', #5571, .T. ) ;
#42587=VECTOR ( 'NONE', #4940, 1000.000000000000000 ) ;
#42589=ORIENTED_EDGE ( 'NONE', *, *, #42778, .T. ) ;
#42599=VERTEX_POINT ( 'NONE', #48369 ) ;
#42610=CARTESIAN_POINT ( 'NONE',  ( 31.89651141207536256, 56.63578868294628421, 170.0000000000000000 ) ) ;
#42619=DIRECTION ( 'NONE',  ( -1.000000000000000000, 0.000000000000000000, 0.000000000000000000 ) ) ;
#42624=DIRECTION ( 'NONE',  ( -1.000000000000000000, 0.000000000000000000, 0.000000000000000000 ) ) ;
#42626=CIRCLE ( 'NONE', #15668, 65.00000000000000000 ) ;
#42634=LINE ( 'NONE', #47551, #65609 ) ;
#42636=ORIENTED_EDGE ( 'NONE', *, *, #56859, .F. ) ;
#42641=CARTESIAN_POINT ( 'NONE',  ( 13.24564585880038159, 63.65041531508843065, 0.000000000000000000 ) ) ;
#42642=CARTESIAN_POINT ( 'NONE',  ( -9.291678301352703784, 76.94361032721405991, 73.58025477438756923 ) ) ;
#42643=EDGE_CURVE ( 'NONE', #47508, #55364, #58944, .T. ) ;
#42645=AXIS2_PLACEMENT_3D ( 'NONE', #22188, #16900, #21483 ) ;
#42658=LINE ( 'NONE', #34729, #41388 ) ;
#42666=EDGE_CURVE ( 'NONE', #43978, #7110, #64934, .T. ) ;
#42669=ORIENTED_EDGE ( 'NONE', *, *, #31073, .T. ) ;
#42682=DIRECTION ( 'NONE',  ( -1.000000000000000000, 0.000000000000000000, 0.000000000000000000 ) ) ;
#42687=DIRECTION ( 'NONE',  ( 0.000000000000000000, 0.000000000000000000, 1.000000000000000000 ) ) ;
#42691=ADVANCED_FACE ( 'NONE', ( #18827 ), #34677, .T. ) ;
#42694=PLANE ( 'NONE',  #55864 ) ;
#42701=EDGE_CURVE ( 'NONE', #35154, #38444, #56643, .T. ) ;
#42706=EDGE_CURVE ( 'NONE', #14371, #35720, #48727, .T. ) ;
#42710=LINE ( 'NONE', #36758, #59548 ) ;
#42711=LINE ( 'NONE', #16672, #68533 ) ;
#42713=ORIENTED_EDGE ( 'NONE', *, *, #3964, .T. ) ;
#42729=DIRECTION ( 'NONE',  ( -0.9195277725514489076, -0.3930250316539278810, 0.000000000000000000 ) ) ;
#42734=VERTEX_POINT ( 'NONE', #16211 ) ;
#42740=LINE ( 'NONE', #27601, #7461 ) ;
#42742=ORIENTED_EDGE ( 'NONE', *, *, #60981, .T. ) ;
#42750=CARTESIAN_POINT ( 'NONE',  ( -11.75099048680784364, -77.43714764088365143, 133.5802547743875550 ) ) ;
#42756=LINE ( 'NONE', #16029, #48845 ) ;
#42762=CARTESIAN_POINT ( 'NONE',  ( -59.42430146430388049, -27.22983999535795618, 6.377659838150141321E-18 ) ) ;
#42764=ORIENTED_EDGE ( 'NONE', *, *, #57099, .T. ) ;
#42766=EDGE_LOOP ( 'NONE', ( #16089, #30844, #38997, #12061 ) ) ;
#42777=VERTEX_POINT ( 'NONE', #26776 ) ;
#42778=EDGE_CURVE ( 'NONE', #9035, #63750, #24802, .T. ) ;
#42790=ORIENTED_EDGE ( 'NONE', *, *, #50252, .F. ) ;
#42795=ADVANCED_FACE ( 'NONE', ( #64398 ), #9307, .T. ) ;
#42802=ORIENTED_EDGE ( 'NONE', *, *, #7801, .F. ) ;
#42803=CARTESIAN_POINT ( 'NONE',  ( -39.55079474733624068, -51.59997227571039957, 41.38025477438755928 ) ) ;
#42805=DIRECTION ( 'NONE',  ( 0.000000000000000000, 0.000000000000000000, 1.000000000000000000 ) ) ;
#42818=DIRECTION ( 'NONE',  ( -1.000000000000000000, 0.000000000000000000, 0.000000000000000000 ) ) ;
#42819=VERTEX_POINT ( 'NONE', #21828 ) ;
#42829=DIRECTION ( 'NONE',  ( -1.000000000000000000, 0.000000000000000000, 0.000000000000000000 ) ) ;
#42831=AXIS2_PLACEMENT_3D ( 'NONE', #28678, #33265, #17411 ) ;
#42834=CARTESIAN_POINT ( 'NONE',  ( 0.000000000000000000, 0.000000000000000000, 41.38025477438755928 ) ) ;
#42844=DIRECTION ( 'NONE',  ( 1.000000000000000000, 0.000000000000000000, 0.000000000000000000 ) ) ;
#42847=CARTESIAN_POINT ( 'NONE',  ( 41.72486082342823721, -50.31647622756196370, 3.125053320693569132E-16 ) ) ;
#42853=EDGE_LOOP ( 'NONE', ( #57738, #43648, #56935, #23898, #64358, #12355, #3672, #43603, #48748 ) ) ;
#42856=EDGE_CURVE ( 'NONE', #23240, #14014, #7052, .T. ) ;
#42865=VERTEX_POINT ( 'NONE', #54529 ) ;
#42867=ORIENTED_EDGE ( 'NONE', *, *, #38012, .F. ) ;
#42871=CYLINDRICAL_SURFACE ( 'NONE', #26474, 65.36598343705435354 ) ;
#42875=VECTOR ( 'NONE', #4350, 1000.000000000000114 ) ;
#42876=CARTESIAN_POINT ( 'NONE',  ( 0.000000000000000000, 0.000000000000000000, 2.000000000000001776 ) ) ;
#42880=ORIENTED_EDGE ( 'NONE', *, *, #66000, .T. ) ;
#42882=CARTESIAN_POINT ( 'NONE',  ( 49.76301652092165995, 41.81676920493114835, 170.0000000000000000 ) ) ;
#42885=VERTEX_POINT ( 'NONE', #30253 ) ;
#42894=VERTEX_POINT ( 'NONE', #25330 ) ;
#42896=ORIENTED_EDGE ( 'NONE', *, *, #14153, .T. ) ;
#42900=CARTESIAN_POINT ( 'NONE',  ( -33.15588700722115334, 4.239136313921378907, 6.893343212288942645 ) ) ;
#42909=CARTESIAN_POINT ( 'NONE',  ( 23.17627457812186620, -71.32923872213625316, 0.000000000000000000 ) ) ;
#42925=VERTEX_POINT ( 'NONE', #67892 ) ;
#42926=EDGE_CURVE ( 'NONE', #69067, #10198, #31990, .T. ) ;
#42928=EDGE_CURVE ( 'NONE', #68299, #39568, #30596, .T. ) ;
#42934=DIRECTION ( 'NONE',  ( 0.4738686624730094610, -0.8805955318567321166, 0.000000000000000000 ) ) ;
#42938=ORIENTED_EDGE ( 'NONE', *, *, #31321, .T. ) ;
#42945=DIRECTION ( 'NONE',  ( 4.573512162503259427E-19, 5.081588203714612465E-18, -1.000000000000000000 ) ) ;
#42959=PLANE ( 'NONE',  #33309 ) ;
#42971=CARTESIAN_POINT ( 'NONE',  ( 26.12852347772543737, 100.0000000000000000, 129.5802547743875550 ) ) ;
#42972=CIRCLE ( 'NONE', #68793, 63.00000000000000000 ) ;
#42986=ORIENTED_EDGE ( 'NONE', *, *, #30873, .T. ) ;
#42989=AXIS2_PLACEMENT_3D ( 'NONE', #39181, #17000, #12440 ) ;
#42995=CARTESIAN_POINT ( 'NONE',  ( 36.85262215550149278, -53.56030941157680303, 170.0000000000000000 ) ) ;
#43003=ORIENTED_EDGE ( 'NONE', *, *, #66795, .F. ) ;
#43009=EDGE_CURVE ( 'NONE', #57368, #43248, #21406, .T. ) ;
#43014=EDGE_CURVE ( 'NONE', #14760, #50465, #59032, .T. ) ;
#43035=DIRECTION ( 'NONE',  ( 1.000000000000000000, 0.000000000000000000, 0.000000000000000000 ) ) ;
#43036=ORIENTED_EDGE ( 'NONE', *, *, #56793, .T. ) ;
#43040=ORIENTED_EDGE ( 'NONE', *, *, #37560, .F. ) ;
#43046=EDGE_CURVE ( 'NONE', #57672, #30275, #55499, .T. ) ;
#43049=EDGE_CURVE ( 'NONE', #67765, #33172, #59721, .T. ) ;
#43057=CARTESIAN_POINT ( 'NONE',  ( 24.39800339187844003, 60.26242556095705538, 0.000000000000000000 ) ) ;
#43058=LINE ( 'NONE', #5093, #26249 ) ;
#43065=LINE ( 'NONE', #59584, #60053 ) ;
#43071=ORIENTED_EDGE ( 'NONE', *, *, #33742, .T. ) ;
#43075=CYLINDRICAL_SURFACE ( 'NONE', #56562, 65.00000000000000000 ) ;
#43076=DIRECTION ( 'NONE',  ( -0.000000000000000000, -0.000000000000000000, -1.000000000000000000 ) ) ;
#43082=VERTEX_POINT ( 'NONE', #11530 ) ;
#43084=EDGE_CURVE ( 'NONE', #8339, #6977, #28633, .T. ) ;
#43091=VECTOR ( 'NONE', #48859, 1000.000000000000000 ) ;
#43097=DIRECTION ( 'NONE',  ( -0.000000000000000000, -0.000000000000000000, -1.000000000000000000 ) ) ;
#43099=CARTESIAN_POINT ( 'NONE',  ( 0.000000000000000000, 0.000000000000000000, 41.38025477438755928 ) ) ;
#43115=DIRECTION ( 'NONE',  ( -0.3930250316539148359, -0.9195277725514544587, 0.000000000000000000 ) ) ;
#43117=DIRECTION ( 'NONE',  ( -0.9639628606958550172, 0.2660368455666687892, 0.000000000000000000 ) ) ;
#43119=LINE ( 'NONE', #36829, #49359 ) ;
#43124=CONICAL_SURFACE ( 'NONE', #29636, 65.00000000000000000, 0.7853981633974497223 ) ;
#43131=CARTESIAN_POINT ( 'NONE',  ( 10.18313837588858384, 65.86279856773080610, 34.48241795236666718 ) ) ;
#43152=FACE_OUTER_BOUND ( 'NONE', #46812, .T. ) ;
#43166=ORIENTED_EDGE ( 'NONE', *, *, #31987, .T. ) ;
#43168=CARTESIAN_POINT ( 'NONE',  ( -66.47744216009887452, -4.728025614004670807, 34.48241795236666718 ) ) ;
#43179=CYLINDRICAL_SURFACE ( 'NONE', #3852, 65.36598343705435354 ) ;
#43181=VECTOR ( 'NONE', #32610, 1000.000000000000114 ) ;
#43186=EDGE_CURVE ( 'NONE', #10198, #69476, #9402, .T. ) ;
#43191=CARTESIAN_POINT ( 'NONE',  ( 13.24564585880132839, -63.65041531508827433, 43.58025477438756923 ) ) ;
#43199=ORIENTED_EDGE ( 'NONE', *, *, #23843, .T. ) ;
#43206=DIRECTION ( 'NONE',  ( 0.9362348706397369824, 0.3513748240813435175, 0.000000000000000000 ) ) ;
#43209=VERTEX_POINT ( 'NONE', #42439 ) ;
#43212=ORIENTED_EDGE ( 'NONE', *, *, #25901, .F. ) ;
#43216=VECTOR ( 'NONE', #17618, 1000.000000000000000 ) ;
#43225=EDGE_CURVE ( 'NONE', #32511, #20457, #63213, .T. ) ;
#43226=CYLINDRICAL_SURFACE ( 'NONE', #38735, 10.00000000000000000 ) ;
#43228=ORIENTED_EDGE ( 'NONE', *, *, #58649, .T. ) ;
#43248=VERTEX_POINT ( 'NONE', #47703 ) ;
#43251=CARTESIAN_POINT ( 'NONE',  ( -4.164416015345870470, 64.86646004871185767, 133.5802547743875550 ) ) ;
#43254=EDGE_CURVE ( 'NONE', #3570, #54048, #69164, .T. ) ;
#43256=ORIENTED_EDGE ( 'NONE', *, *, #12616, .F. ) ;
#43258=VERTEX_POINT ( 'NONE', #38547 ) ;
#43264=ORIENTED_EDGE ( 'NONE', *, *, #40726, .F. ) ;
#43266=ADVANCED_FACE ( 'NONE', ( #26948 ), #64943, .T. ) ;
#43271=AXIS2_PLACEMENT_3D ( 'NONE', #61359, #45176, #23398 ) ;
#43277=AXIS2_PLACEMENT_3D ( 'NONE', #47519, #48545, #9917 ) ;
#43280=CARTESIAN_POINT ( 'NONE',  ( 31.71171429570986788, 10.56647038281439954, 6.893343212288932875 ) ) ;
#43281=DIRECTION ( 'NONE',  ( 0.000000000000000000, 0.000000000000000000, 1.000000000000000000 ) ) ;
#43284=ORIENTED_EDGE ( 'NONE', *, *, #60610, .T. ) ;
#43295=LINE ( 'NONE', #37002, #9561 ) ;
#43299=ORIENTED_EDGE ( 'NONE', *, *, #62319, .F. ) ;
#43303=CARTESIAN_POINT ( 'NONE',  ( 29.86848256228521237, 58.14280299503739258, 43.58025477438756212 ) ) ;
#43320=VECTOR ( 'NONE', #58629, 1000.000000000000000 ) ;
#43322=ORIENTED_EDGE ( 'NONE', *, *, #15075, .F. ) ;
#43333=EDGE_CURVE ( 'NONE', #25277, #60956, #9553, .T. ) ;
#43337=CONICAL_SURFACE ( 'NONE', #15292, 65.00000000000000000, 0.7853981633974497223 ) ;
#43339=ORIENTED_EDGE ( 'NONE', *, *, #56385, .T. ) ;
#43352=DIRECTION ( 'NONE',  ( -0.9362348706397369824, -0.3513748240813435175, 0.000000000000000000 ) ) ;
#43369=DIRECTION ( 'NONE',  ( -0.3930250316539278255, 0.9195277725514487965, 0.000000000000000000 ) ) ;
#43373=VECTOR ( 'NONE', #11663, 1000.000000000000000 ) ;
#43376=ORIENTED_EDGE ( 'NONE', *, *, #9993, .T. ) ;
#43377=CONICAL_SURFACE ( 'NONE', #33318, 74.95140232871122521, 0.8777644062502172329 ) ;
#43382=DIRECTION ( 'NONE',  ( 0.000000000000000000, 0.000000000000000000, 1.000000000000000000 ) ) ;
#43383=CARTESIAN_POINT ( 'NONE',  ( 0.000000000000000000, 0.000000000000000000, 41.38025477438755928 ) ) ;
#43386=PLANE ( 'NONE',  #27517 ) ;
#43388=ORIENTED_EDGE ( 'NONE', *, *, #22305, .T. ) ;
#43391=ORIENTED_EDGE ( 'NONE', *, *, #25685, .F. ) ;
#43402=VERTEX_POINT ( 'NONE', #69074 ) ;
#43414=DIRECTION ( 'NONE',  ( 1.000000000000000000, 0.000000000000000000, 0.000000000000000000 ) ) ;
#43417=DIRECTION ( 'NONE',  ( -0.000000000000000000, -0.000000000000000000, -1.000000000000000000 ) ) ;
#43420=ORIENTED_EDGE ( 'NONE', *, *, #14616, .T. ) ;
#43425=CARTESIAN_POINT ( 'NONE',  ( 4.165045035620146940, 64.88046627338042072, 43.58025477438756923 ) ) ;
#43428=VECTOR ( 'NONE', #54596, 1000.000000000000000 ) ;
#43435=ORIENTED_EDGE ( 'NONE', *, *, #56326, .F. ) ;
#43446=EDGE_CURVE ( 'NONE', #25227, #37904, #10343, .T. ) ;
#43451=FACE_OUTER_BOUND ( 'NONE', #54576, .T. ) ;
#43455=CARTESIAN_POINT ( 'NONE',  ( 55.14772863908626732, 34.40534879854737227, 170.0000000000000000 ) ) ;
#43460=CARTESIAN_POINT ( 'NONE',  ( -49.77357484059130854, -41.82599373102874551, 3.061616997868437868E-16 ) ) ;
#43469=CIRCLE ( 'NONE', #13228, 74.95140232871122521 ) ;
#43478=CIRCLE ( 'NONE', #69304, 25.12245591505646303 ) ;
#43481=DIRECTION ( 'NONE',  ( 0.000000000000000000, 0.000000000000000000, 1.000000000000000000 ) ) ;
#43487=VECTOR ( 'NONE', #28968, 1000.000000000000114 ) ;
#43489=CARTESIAN_POINT ( 'NONE',  ( -21.95369412746257254, 11.95973721106814835, 0.000000000000000000 ) ) ;
#43497=ORIENTED_EDGE ( 'NONE', *, *, #11730, .F. ) ;
#43521=VERTEX_POINT ( 'NONE', #11374 ) ;
#43529=EDGE_CURVE ( 'NONE', #2204, #21329, #52226, .T. ) ;
#43531=EDGE_LOOP ( 'NONE', ( #37859, #61008, #23311, #54867 ) ) ;
#43532=ORIENTED_EDGE ( 'NONE', *, *, #26231, .F. ) ;
#43533=VECTOR ( 'NONE', #35800, 1000.000000000000114 ) ;
#43536=DIRECTION ( 'NONE',  ( 0.7071067811865485719, 0.000000000000000000, 0.7071067811865465735 ) ) ;
#43537=ORIENTED_EDGE ( 'NONE', *, *, #67999, .F. ) ;
#43539=CARTESIAN_POINT ( 'NONE',  ( -15.67984581960975632, -63.08044415722883969, 170.0000000000000000 ) ) ;
#43542=CARTESIAN_POINT ( 'NONE',  ( -55.89173064941029878, -16.72186800183967748, 27.58472369374500843 ) ) ;
#43543=DIRECTION ( 'NONE',  ( 0.9362348706397369824, 0.3513748240813435175, -0.000000000000000000 ) ) ;
#43549=ORIENTED_EDGE ( 'NONE', *, *, #9957, .T. ) ;
#43551=EDGE_CURVE ( 'NONE', #12492, #31642, #48825, .T. ) ;
#43559=EDGE_CURVE ( 'NONE', #6090, #37545, #59854, .T. ) ;
#43570=CARTESIAN_POINT ( 'NONE',  ( -3.364862276287834408, -74.92447999059862696, 43.58025477438756212 ) ) ;
#43573=DIRECTION ( 'NONE',  ( 0.6234898018587431423, -0.7818314824680220321, 0.000000000000000000 ) ) ;
#43574=EDGE_CURVE ( 'NONE', #14487, #16778, #38778, .T. ) ;
#43579=DIRECTION ( 'NONE',  ( 1.000000000000000000, 0.000000000000000000, 0.000000000000000000 ) ) ;
#43580=ORIENTED_EDGE ( 'NONE', *, *, #34557, .F. ) ;
#43589=VECTOR ( 'NONE', #22645, 1000.000000000000114 ) ;
#43590=DIRECTION ( 'NONE',  ( 0.9749279121818226201, 0.2225209339563184452, -0.000000000000000000 ) ) ;
#43603=ORIENTED_EDGE ( 'NONE', *, *, #49402, .F. ) ;
#43605=VERTEX_POINT ( 'NONE', #66612 ) ;
#43614=ORIENTED_EDGE ( 'NONE', *, *, #38124, .T. ) ;
#43618=VECTOR ( 'NONE', #30569, 999.9999999999998863 ) ;
#43622=CIRCLE ( 'NONE', #47009, 65.36598343705435354 ) ;
#43623=CARTESIAN_POINT ( 'NONE',  ( 44.01696072966020523, -47.84694004974148385, 43.58025477438756923 ) ) ;
#43642=FACE_OUTER_BOUND ( 'NONE', #48874, .T. ) ;
#43648=ORIENTED_EDGE ( 'NONE', *, *, #30143, .F. ) ;
#43650=EDGE_LOOP ( 'NONE', ( #33201, #45741, #13115, #64369 ) ) ;
#43677=CARTESIAN_POINT ( 'NONE',  ( 18.89356949897907967, -62.19351277735682970, 170.0000000000000000 ) ) ;
#43686=DIRECTION ( 'NONE',  ( 0.9362348706397369824, 0.3513748240813435175, 0.000000000000000000 ) ) ;
#43692=ORIENTED_EDGE ( 'NONE', *, *, #30331, .F. ) ;
#43697=ORIENTED_EDGE ( 'NONE', *, *, #54438, .T. ) ;
#43698=ORIENTED_EDGE ( 'NONE', *, *, #2444, .F. ) ;
#43711=AXIS2_PLACEMENT_3D ( 'NONE', #15696, #30850, #42082 ) ;
#43717=VERTEX_POINT ( 'NONE', #25429 ) ;
#43722=ADVANCED_FACE ( 'NONE', ( #35632 ), #57084, .T. ) ;
#43726=LINE ( 'NONE', #66275, #67967 ) ;
#43732=DIRECTION ( 'NONE',  ( -0.6234898018587318180, -0.7818314824680311359, 0.000000000000000000 ) ) ;
#43743=ORIENTED_EDGE ( 'NONE', *, *, #36936, .F. ) ;
#43749=DIRECTION ( 'NONE',  ( 0.9989930665413144784, 0.04486483035051863633, 5.102127870520020458E-18 ) ) ;
#43750=AXIS2_PLACEMENT_3D ( 'NONE', #51797, #61994, #51111 ) ;
#43758=( NAMED_UNIT ( * ) SI_UNIT ( $, .STERADIAN. ) SOLID_ANGLE_UNIT ( ) );
#43760=DIRECTION ( 'NONE',  ( -0.000000000000000000, 0.000000000000000000, -1.000000000000000000 ) ) ;
#43770=FACE_OUTER_BOUND ( 'NONE', #24940, .T. ) ;
#43773=ORIENTED_EDGE ( 'NONE', *, *, #3920, .F. ) ;
#43777=FACE_OUTER_BOUND ( 'NONE', #33071, .T. ) ;
#43782=VERTEX_POINT ( 'NONE', #9069 ) ;
#43793=DIRECTION ( 'NONE',  ( -0.000000000000000000, 1.000000000000000000, 2.500042656554809847E-16 ) ) ;
#43797=VERTEX_POINT ( 'NONE', #40717 ) ;
#43811=CARTESIAN_POINT ( 'NONE',  ( 41.72486082342749825, 50.31647622756256766, 43.58025477438756212 ) ) ;
#43822=FACE_OUTER_BOUND ( 'NONE', #5157, .T. ) ;
#43833=CARTESIAN_POINT ( 'NONE',  ( -36.84489839129339828, 53.54860840895182150, 170.0000000000000000 ) ) ;
#43836=DIRECTION ( 'NONE',  ( -0.000000000000000000, -0.000000000000000000, 1.000000000000000000 ) ) ;
#43839=DIRECTION ( 'NONE',  ( 2.437361367520478414E-16, 5.563118268672117023E-17, 1.000000000000000000 ) ) ;
#43858=ORIENTED_EDGE ( 'NONE', *, *, #46140, .T. ) ;
#43859=LINE ( 'NONE', #17124, #34669 ) ;
#43868=DIRECTION ( 'NONE',  ( 0.000000000000000000, 0.000000000000000000, 1.000000000000000000 ) ) ;
#43881=VECTOR ( 'NONE', #36697, 1000.000000000000000 ) ;
#43882=CARTESIAN_POINT ( 'NONE',  ( 0.000000000000000000, 0.000000000000000000, 41.38025477438755928 ) ) ;
#43887=EDGE_CURVE ( 'NONE', #47103, #6327, #68498, .T. ) ;
#43894=ORIENTED_EDGE ( 'NONE', *, *, #37306, .F. ) ;
#43896=ORIENTED_EDGE ( 'NONE', *, *, #39393, .T. ) ;
#43897=VERTEX_POINT ( 'NONE', #47369 ) ;
#43901=DIRECTION ( 'NONE',  ( -0.000000000000000000, 0.000000000000000000, -1.000000000000000000 ) ) ;
#43919=ORIENTED_EDGE ( 'NONE', *, *, #10683, .F. ) ;
#43922=VERTEX_POINT ( 'NONE', #62765 ) ;
#43931=ORIENTED_EDGE ( 'NONE', *, *, #37854, .T. ) ;
#43945=VECTOR ( 'NONE', #33577, 1000.000000000000000 ) ;
#43948=ORIENTED_EDGE ( 'NONE', *, *, #40820, .T. ) ;
#43949=VERTEX_POINT ( 'NONE', #51175 ) ;
#43956=EDGE_LOOP ( 'NONE', ( #11147, #6456, #6479, #5226, #35463, #68386, #9661, #23859, #59724 ) ) ;
#43960=ORIENTED_EDGE ( 'NONE', *, *, #48640, .F. ) ;
#43963=ADVANCED_FACE ( 'NONE', ( #35694 ), #34997, .T. ) ;
#43969=CARTESIAN_POINT ( 'NONE',  ( 44.01696072965949469, 47.84694004974210912, 43.58025477438756923 ) ) ;
#43977=FACE_OUTER_BOUND ( 'NONE', #30305, .T. ) ;
#43978=VERTEX_POINT ( 'NONE', #51858 ) ;
#43982=EDGE_LOOP ( 'NONE', ( #6287, #37370, #20773, #50302 ) ) ;
#43988=CARTESIAN_POINT ( 'NONE',  ( 19.71799482800311054, 15.56722426018198036, 0.000000000000000000 ) ) ;
#43989=CARTESIAN_POINT ( 'NONE',  ( -44.26023579658940577, 48.10138582123773432, 41.38025477438755928 ) ) ;
#43996=CIRCLE ( 'NONE', #13694, 25.12245591505646303 ) ;
#43999=ORIENTED_EDGE ( 'NONE', *, *, #42106, .T. ) ;
#44001=ORIENTED_EDGE ( 'NONE', *, *, #8252, .F. ) ;
#44005=FACE_OUTER_BOUND ( 'NONE', #10405, .T. ) ;
#44009=DIRECTION ( 'NONE',  ( 0.000000000000000000, 0.000000000000000000, 1.000000000000000000 ) ) ;
#44013=ORIENTED_EDGE ( 'NONE', *, *, #3203, .T. ) ;
#44020=ORIENTED_EDGE ( 'NONE', *, *, #57657, .F. ) ;
#44030=CARTESIAN_POINT ( 'NONE',  ( -64.83840629396348731, 4.580509716059292913, 170.0000000000000000 ) ) ;
#44037=EDGE_CURVE ( 'NONE', #67474, #28312, #40959, .T. ) ;
#44039=ORIENTED_EDGE ( 'NONE', *, *, #42778, .F. ) ;
#44046=LINE ( 'NONE', #65526, #10555 ) ;
#44047=DIRECTION ( 'NONE',  ( 1.000000000000000000, 0.000000000000000000, 0.000000000000000000 ) ) ;
#44050=VERTEX_POINT ( 'NONE', #1880 ) ;
#44051=EDGE_CURVE ( 'NONE', #7953, #18463, #34230, .T. ) ;
#44059=CARTESIAN_POINT ( 'NONE',  ( 34.43940527065382895, 66.63700071734666608, 170.0000000000000000 ) ) ;
#44067=EDGE_LOOP ( 'NONE', ( #42020, #18325, #60866, #56969 ) ) ;
#44074=LINE ( 'NONE', #13478, #5138 ) ;
#44078=CARTESIAN_POINT ( 'NONE',  ( -62.31345272479883590, -18.49415068377726357, 40.00000000000003553 ) ) ;
#44080=ORIENTED_EDGE ( 'NONE', *, *, #47080, .T. ) ;
#44090=ORIENTED_EDGE ( 'NONE', *, *, #3985, .F. ) ;
#44093=CIRCLE ( 'NONE', #40751, 24.99999999999985434 ) ;
#44111=FACE_OUTER_BOUND ( 'NONE', #33910, .T. ) ;
#44113=LINE ( 'NONE', #48334, #21489 ) ;
#44119=ORIENTED_EDGE ( 'NONE', *, *, #11096, .T. ) ;
#44123=ORIENTED_EDGE ( 'NONE', *, *, #40010, .F. ) ;
#44124=ORIENTED_EDGE ( 'NONE', *, *, #49141, .T. ) ;
#44128=ORIENTED_EDGE ( 'NONE', *, *, #4761, .F. ) ;
#44150=EDGE_CURVE ( 'NONE', #46943, #6675, #60093, .T. ) ;
#44151=EDGE_CURVE ( 'NONE', #56795, #65664, #24370, .T. ) ;
#44159=CARTESIAN_POINT ( 'NONE',  ( -72.29721455218913206, 19.95276341750015803, 0.000000000000000000 ) ) ;
#44160=CARTESIAN_POINT ( 'NONE',  ( -9.273616082387997395, -77.77273080542778416, 133.5802547743875550 ) ) ;
#44173=EDGE_LOOP ( 'NONE', ( #50711, #57696, #51993, #32260 ) ) ;
#44175=ORIENTED_EDGE ( 'NONE', *, *, #5238, .F. ) ;
#44177=AXIS2_PLACEMENT_3D ( 'NONE', #8322, #66389, #34369 ) ;
#44182=LINE ( 'NONE', #50525, #47933 ) ;
#44186=FACE_OUTER_BOUND ( 'NONE', #51869, .T. ) ;
#44193=VECTOR ( 'NONE', #31117, 1000.000000000000114 ) ;
#44198=EDGE_CURVE ( 'NONE', #19302, #41523, #4621, .T. ) ;
#44203=CARTESIAN_POINT ( 'NONE',  ( -55.15976438495154355, 34.41253982194034933, 3.061616997868437868E-16 ) ) ;
#44211=EDGE_CURVE ( 'NONE', #32779, #8257, #58093, .T. ) ;
#44215=FACE_OUTER_BOUND ( 'NONE', #6434, .T. ) ;
#44222=DIRECTION ( 'NONE',  ( -0.4738686624730094610, 0.8805955318567321166, 0.000000000000000000 ) ) ;
#44230=AXIS2_PLACEMENT_3D ( 'NONE', #46535, #41957, #9952 ) ;
#44232=ORIENTED_EDGE ( 'NONE', *, *, #47080, .F. ) ;
#44235=EDGE_CURVE ( 'NONE', #37998, #65969, #18302, .T. ) ;
#44239=ORIENTED_EDGE ( 'NONE', *, *, #17391, .T. ) ;
#44242=AXIS2_PLACEMENT_3D ( 'NONE', #54457, #26714, #22469 ) ;
#44243=CIRCLE ( 'NONE', #13939, 65.00000000000000000 ) ;
#44244=DIRECTION ( 'NONE',  ( -1.000000000000000000, 0.000000000000000000, 0.000000000000000000 ) ) ;
#44246=AXIS2_PLACEMENT_3D ( 'NONE', #49936, #23227, #44676 ) ;
#44247=DIRECTION ( 'NONE',  ( -1.000000000000000000, 0.000000000000000000, 0.000000000000000000 ) ) ;
#44255=CYLINDRICAL_SURFACE ( 'NONE', #3286, 65.36598343705435354 ) ;
#44259=LINE ( 'NONE', #65740, #7014 ) ;
#44260=CARTESIAN_POINT ( 'NONE',  ( -4.613603609465520172, 74.86839895266042788, 170.0000000000000000 ) ) ;
#44264=CARTESIAN_POINT ( 'NONE',  ( 10.01137213834967987, -64.59476928204588830, 3.125053320693562722E-16 ) ) ;
#44266=DIRECTION ( 'NONE',  ( -0.000000000000000000, -0.000000000000000000, 1.000000000000000000 ) ) ;
#44275=CARTESIAN_POINT ( 'NONE',  ( -18.15845058245935562, -17.18344181019548955, 0.000000000000000000 ) ) ;
#44277=LINE ( 'NONE', #66125, #7265 ) ;
#44278=CARTESIAN_POINT ( 'NONE',  ( -0.4701925031012952338, -38.33111675900010340, 13.32819299319724315 ) ) ;
#44286=AXIS2_PLACEMENT_3D ( 'NONE', #15402, #48082, #63593 ) ;
#44287=ORIENTED_EDGE ( 'NONE', *, *, #47863, .T. ) ;
#44289=VERTEX_POINT ( 'NONE', #34504 ) ;
#44291=DIRECTION ( 'NONE',  ( 1.000000000000000000, 0.000000000000000000, 0.000000000000000000 ) ) ;
#44297=DIRECTION ( 'NONE',  ( 0.3513748240813305279, 0.9362348706397417564, 2.500042656554809847E-16 ) ) ;
#44312=ORIENTED_EDGE ( 'NONE', *, *, #36868, .T. ) ;
#44314=ORIENTED_EDGE ( 'NONE', *, *, #37286, .F. ) ;
#44317=CARTESIAN_POINT ( 'NONE',  ( 0.000000000000000000, 0.000000000000000000, 40.00000000000003553 ) ) ;
#44318=ORIENTED_EDGE ( 'NONE', *, *, #29701, .T. ) ;
#44321=EDGE_CURVE ( 'NONE', #37971, #47893, #51013, .T. ) ;
#44324=ADVANCED_FACE ( 'NONE', ( #19685 ), #46070, .T. ) ;
#44332=ORIENTED_EDGE ( 'NONE', *, *, #49191, .F. ) ;
#44345=VECTOR ( 'NONE', #2009, 1000.000000000000000 ) ;
#44348=VECTOR ( 'NONE', #30241, 1000.000000000000000 ) ;
#44362=CARTESIAN_POINT ( 'NONE',  ( -51.82969867401435948, -54.20961478705483927, 0.000000000000000000 ) ) ;
#44366=VERTEX_POINT ( 'NONE', #56984 ) ;
#44368=DIRECTION ( 'NONE',  ( -0.000000000000000000, -0.000000000000000000, -1.000000000000000000 ) ) ;
#44370=CARTESIAN_POINT ( 'NONE',  ( 0.000000000000000000, 0.000000000000000000, 0.000000000000000000 ) ) ;
#44371=CARTESIAN_POINT ( 'NONE',  ( -52.00772271844017780, -26.43299457339944425, 27.58472369387556000 ) ) ;
#44387=ORIENTED_EDGE ( 'NONE', *, *, #3924, .T. ) ;
#44389=DIRECTION ( 'NONE',  ( -0.000000000000000000, 0.000000000000000000, -1.000000000000000000 ) ) ;
#44399=LINE ( 'NONE', #65885, #55028 ) ;
#44403=CARTESIAN_POINT ( 'NONE',  ( 19.71799482800311054, 15.56722426018198036, 0.000000000000000000 ) ) ;
#44404=ORIENTED_EDGE ( 'NONE', *, *, #4908, .T. ) ;
#44412=CARTESIAN_POINT ( 'NONE',  ( -50.92620509423013431, -55.07344309828844331, 43.58025477438756923 ) ) ;
#44425=CARTESIAN_POINT ( 'NONE',  ( 0.000000000000000000, 0.000000000000000000, 41.38025477438755928 ) ) ;
#44426=ORIENTED_EDGE ( 'NONE', *, *, #52246, .T. ) ;
#44427=ORIENTED_EDGE ( 'NONE', *, *, #10375, .F. ) ;
#44432=CARTESIAN_POINT ( 'NONE',  ( -74.69807204964297398, 6.722948167756991111, 43.58025477438756212 ) ) ;
#44437=ORIENTED_EDGE ( 'NONE', *, *, #22814, .T. ) ;
#44438=VECTOR ( 'NONE', #18833, 1000.000000000000227 ) ;
#44447=EDGE_CURVE ( 'NONE', #29231, #11589, #41084, .T. ) ;
#44448=AXIS2_PLACEMENT_3D ( 'NONE', #42049, #4758, #15666 ) ;
#44449=CARTESIAN_POINT ( 'NONE',  ( 13.24564585880131773, -63.65041531508827433, 3.061616997868437868E-16 ) ) ;
#44450=CARTESIAN_POINT ( 'NONE',  ( 0.000000000000000000, 0.000000000000000000, 170.0000000000000000 ) ) ;
#44452=CARTESIAN_POINT ( 'NONE',  ( 7.533997733929801655, -64.93035244659006366, 43.58025477438756212 ) ) ;
#44453=ORIENTED_EDGE ( 'NONE', *, *, #24050, .T. ) ;
#44455=VERTEX_POINT ( 'NONE', #54001 ) ;
#44457=ADVANCED_FACE ( 'NONE', ( #17429 ), #33285, .T. ) ;
#44458=ORIENTED_EDGE ( 'NONE', *, *, #42021, .F. ) ;
#44459=PLANE ( 'NONE',  #61935 ) ;
#44467=CARTESIAN_POINT ( 'NONE',  ( 10.00000000000000000, 1.224646799147353256E-15, 170.0010000000000048 ) ) ;
#44491=AXIS2_PLACEMENT_3D ( 'NONE', #28162, #1096, #40124 ) ;
#44502=VECTOR ( 'NONE', #13948, 1000.000000000000000 ) ;
#44503=CONICAL_SURFACE ( 'NONE', #64736, 74.95140232871122521, 0.8777644062502172329 ) ;
#44504=CARTESIAN_POINT ( 'NONE',  ( 30.83327692011752674, 12.90705744104631947, 6.893342932883484764 ) ) ;
#44507=CIRCLE ( 'NONE', #42250, 24.99999999999985434 ) ;
#44511=CIRCLE ( 'NONE', #31070, 74.95140232871122521 ) ;
#44518=DIRECTION ( 'NONE',  ( 0.000000000000000000, 0.000000000000000000, 1.000000000000000000 ) ) ;
#44519=VERTEX_POINT ( 'NONE', #48724 ) ;
#44528=LINE ( 'NONE', #44160, #7787 ) ;
#44531=ORIENTED_EDGE ( 'NONE', *, *, #5550, .T. ) ;
#44544=ADVANCED_FACE ( 'NONE', ( #1259 ), #65279, .F. ) ;
#44553=EDGE_CURVE ( 'NONE', #33141, #27057, #63109, .T. ) ;
#44558=DIRECTION ( 'NONE',  ( 0.000000000000000000, 0.000000000000000000, 1.000000000000000000 ) ) ;
#44565=DIRECTION ( 'NONE',  ( -0.000000000000000000, -0.000000000000000000, -1.000000000000000000 ) ) ;
#44567=ADVANCED_FACE ( 'NONE', ( #4209 ), #25674, .T. ) ;
#44574=VERTEX_POINT ( 'NONE', #32577 ) ;
#44576=CARTESIAN_POINT ( 'NONE',  ( 75.00000000000000000, 1.249999999999979350, 170.0000000000000000 ) ) ;
#44580=CARTESIAN_POINT ( 'NONE',  ( -26.69131247781301752, 59.26697088776972322, 40.00000000000003553 ) ) ;
#44587=ORIENTED_EDGE ( 'NONE', *, *, #49458, .F. ) ;
#44588=DIRECTION ( 'NONE',  ( 1.000000000000000000, 0.000000000000000000, 0.000000000000000000 ) ) ;
#44596=CARTESIAN_POINT ( 'NONE',  ( -41.50537345350708307, 50.04124777106294886, 170.0000000000000000 ) ) ;
#44601=EDGE_CURVE ( 'NONE', #26798, #38050, #47105, .T. ) ;
#44602=DIRECTION ( 'NONE',  ( -0.000000000000000000, -0.000000000000000000, 1.000000000000000000 ) ) ;
#44615=B_SPLINE_CURVE_WITH_KNOTS ( 'NONE', 3,
 ( #68747, #68423, #53602, #47291, #63144, #4733 ),
 .UNSPECIFIED., .F., .F.,
 ( 4, 2, 4 ),
 ( 0.03218938496963300727, 0.06469835385212996393, 0.09720732273462692752 ),
 .UNSPECIFIED. ) ;
#44624=EDGE_CURVE ( 'NONE', #14895, #35197, #33202, .T. ) ;
#44627=FACE_OUTER_BOUND ( 'NONE', #9022, .T. ) ;
#44628=VERTEX_POINT ( 'NONE', #54354 ) ;
#44635=FACE_OUTER_BOUND ( 'NONE', #5768, .T. ) ;
#44636=DIRECTION ( 'NONE',  ( 0.1785568947986229116, 0.9839295885986321100, 2.500042656554809847E-16 ) ) ;
#44637=ORIENTED_EDGE ( 'NONE', *, *, #41939, .F. ) ;
#44638=VECTOR ( 'NONE', #46125, 999.9999999999998863 ) ;
#44661=VERTEX_POINT ( 'NONE', #12514 ) ;
#44667=LINE ( 'NONE', #50979, #8910 ) ;
#44671=ORIENTED_EDGE ( 'NONE', *, *, #30440, .T. ) ;
#44676=DIRECTION ( 'NONE',  ( -1.000000000000000000, 0.000000000000000000, 0.000000000000000000 ) ) ;
#44680=ORIENTED_EDGE ( 'NONE', *, *, #19462, .F. ) ;
#44687=ORIENTED_EDGE ( 'NONE', *, *, #4761, .T. ) ;
#44691=EDGE_CURVE ( 'NONE', #21788, #60419, #19739, .T. ) ;
#44702=CONICAL_SURFACE ( 'NONE', #12167, 65.00000000000000000, 0.7853981633974497223 ) ;
#44709=EDGE_CURVE ( 'NONE', #30492, #56234, #44870, .T. ) ;
#44718=ORIENTED_EDGE ( 'NONE', *, *, #32783, .F. ) ;
#44730=ORIENTED_EDGE ( 'NONE', *, *, #35558, .T. ) ;
#44735=B_SPLINE_CURVE_WITH_KNOTS ( 'NONE', 3,
 ( #12406, #39480, #54953, #60936, #60240, #61633 ),
 .UNSPECIFIED., .F., .F.,
 ( 4, 2, 4 ),
 ( 1.095770181116721450E-06, 0.03239442681617712289, 0.06478775786217312593 ),
 .UNSPECIFIED. ) ;
#44739=EDGE_CURVE ( 'NONE', #47893, #42894, #7240, .T. ) ;
#44740=EDGE_CURVE ( 'NONE', #64346, #13447, #55063, .T. ) ;
#44747=ADVANCED_FACE ( 'NONE', ( #29385 ), #1773, .T. ) ;
#44749=VECTOR ( 'NONE', #64459, 1000.000000000000000 ) ;
#44765=CARTESIAN_POINT ( 'NONE',  ( 51.85299110299497016, -39.21848821248376282, 43.58025477438756923 ) ) ;
#44771=DIRECTION ( 'NONE',  ( 0.3090169943749446757, 0.9510565162951544194, 0.000000000000000000 ) ) ;
#44774=DIRECTION ( 'NONE',  ( -0.04486483035050447404, -0.9989930665413151445, 0.000000000000000000 ) ) ;
#44776=CYLINDRICAL_SURFACE ( 'NONE', #39088, 65.36598343705435354 ) ;
#44777=EDGE_CURVE ( 'NONE', #36599, #27671, #6881, .T. ) ;
#44780=CARTESIAN_POINT ( 'NONE',  ( -31.90315521289066680, -56.64813493366048647, 3.061616997868437868E-16 ) ) ;
#44782=FACE_OUTER_BOUND ( 'NONE', #20424, .T. ) ;
#44784=ORIENTED_EDGE ( 'NONE', *, *, #53599, .T. ) ;
#44787=CARTESIAN_POINT ( 'NONE',  ( -17.90772993695011550, -72.84144224619156205, 170.0000000000000000 ) ) ;
#44797=ORIENTED_EDGE ( 'NONE', *, *, #12454, .F. ) ;
#44801=VERTEX_POINT ( 'NONE', #50840 ) ;
#44803=ADVANCED_FACE ( 'NONE', ( #24119 ), #8503, .T. ) ;
#44809=VECTOR ( 'NONE', #22125, 1000.000000000000114 ) ;
#44815=ORIENTED_EDGE ( 'NONE', *, *, #21365, .T. ) ;
#44818=DIRECTION ( 'NONE',  ( -0.9639628606958512425, -0.2660368455666826670, 0.000000000000000000 ) ) ;
#44837=DIRECTION ( 'NONE',  ( 0.9009688679024218105, -0.4338837391175525693, 0.000000000000000000 ) ) ;
#44841=VERTEX_POINT ( 'NONE', #36050 ) ;
#44848=DIRECTION ( 'NONE',  ( -0.3090169943749447312, -0.9510565162951544194, 0.000000000000000000 ) ) ;
#44851=PLANE ( 'NONE',  #42831 ) ;
#44852=EDGE_CURVE ( 'NONE', #13054, #10843, #36616, .T. ) ;
#44855=ADVANCED_FACE ( 'NONE', ( #9314 ), #50070, .T. ) ;
#44866=AXIS2_PLACEMENT_3D ( 'NONE', #51622, #14670, #24895 ) ;
#44867=ORIENTED_EDGE ( 'NONE', *, *, #40753, .T. ) ;
#44870=LINE ( 'NONE', #29054, #44438 ) ;
#44882=DIRECTION ( 'NONE',  ( 1.000000000000000000, 0.000000000000000000, 0.000000000000000000 ) ) ;
#44884=LINE ( 'NONE', #61060, #35566 ) ;
#44898=CARTESIAN_POINT ( 'NONE',  ( 29.31537757312406356, -16.05900791856644005, 6.893342934923157195 ) ) ;
#44900=AXIS2_PLACEMENT_3D ( 'NONE', #30743, #29700, #19141 ) ;
#44902=LINE ( 'NONE', #60728, #38268 ) ;
#44904=ORIENTED_EDGE ( 'NONE', *, *, #30411, .F. ) ;
#44907=CARTESIAN_POINT ( 'NONE',  ( -51.84164840787130402, -39.21024726209533640, 40.00000000000003553 ) ) ;
#44911=ORIENTED_EDGE ( 'NONE', *, *, #21405, .F. ) ;
#44914=FACE_OUTER_BOUND ( 'NONE', #32512, .T. ) ;
#44918=DIRECTION ( 'NONE',  ( -2.241020959626955766E-17, 2.489978219820156880E-16, 1.000000000000000000 ) ) ;
#44927=CARTESIAN_POINT ( 'NONE',  ( -12.71198166530289342, -21.52685583500284139, 0.000000000000000000 ) ) ;
#44935=ORIENTED_EDGE ( 'NONE', *, *, #51929, .T. ) ;
#44936=ORIENTED_EDGE ( 'NONE', *, *, #24760, .T. ) ;
#44938=ADVANCED_FACE ( 'NONE', ( #64152 ), #58867, .F. ) ;
#44940=DIRECTION ( 'NONE',  ( 0.000000000000000000, 0.000000000000000000, 1.000000000000000000 ) ) ;
#44941=ORIENTED_EDGE ( 'NONE', *, *, #29392, .F. ) ;
#44960=CARTESIAN_POINT ( 'NONE',  ( -22.15007140920429407, 31.28689709046298617, 13.32819299319723605 ) ) ;
#44969=DIRECTION ( 'NONE',  ( 1.644874880248609566E-16, -1.882710788443290569E-16, 1.000000000000000000 ) ) ;
#44970=ORIENTED_EDGE ( 'NONE', *, *, #60529, .T. ) ;
#44976=VECTOR ( 'NONE', #46020, 999.9999999999998863 ) ;
#44980=DIRECTION ( 'NONE',  ( -0.000000000000000000, 0.000000000000000000, -1.000000000000000000 ) ) ;
#44984=LINE ( 'NONE', #66465, #17158 ) ;
#44991=ORIENTED_EDGE ( 'NONE', *, *, #18054, .T. ) ;
#44992=CARTESIAN_POINT ( 'NONE',  ( -41.05116137042202240, 31.37049953149684356, 26.66469104408689006 ) ) ;
#44996=ADVANCED_FACE ( 'NONE', ( #482 ), #42233, .T. ) ;
#44998=CARTESIAN_POINT ( 'NONE',  ( -31.90315521289065970, -56.64813493366050068, 41.38025477438755928 ) ) ;
#45004=CARTESIAN_POINT ( 'NONE',  ( 48.11816970607299027, -43.69944786993949748, 170.0000000000000000 ) ) ;
#45006=DIRECTION ( 'NONE',  ( 0.1785568947986370392, -0.9839295885986295565, 0.000000000000000000 ) ) ;
#45008=VECTOR ( 'NONE', #31676, 1000.000000000000000 ) ;
#45013=VECTOR ( 'NONE', #45726, 1000.000000000000000 ) ;
#45018=ORIENTED_EDGE ( 'NONE', *, *, #13355, .T. ) ;
#45020=EDGE_CURVE ( 'NONE', #62331, #32020, #11891, .T. ) ;
#45033=ORIENTED_EDGE ( 'NONE', *, *, #704, .T. ) ;
#45037=EDGE_CURVE ( 'NONE', #7248, #59256, #14172, .T. ) ;
#45046=LINE ( 'NONE', #1809, #46267 ) ;
#45049=ORIENTED_EDGE ( 'NONE', *, *, #31596, .T. ) ;
#45056=CARTESIAN_POINT ( 'NONE',  ( 0.000000000000000000, 0.000000000000000000, 0.000000000000000000 ) ) ;
#45057=AXIS2_PLACEMENT_3D ( 'NONE', #22501, #66138, #60826 ) ;
#45059=VECTOR ( 'NONE', #23314, 1000.000000000000000 ) ;
#45067=LINE ( 'NONE', #13417, #52523 ) ;
#45083=DIRECTION ( 'NONE',  ( -0.04486483035051862939, 0.9989930665413143673, 0.000000000000000000 ) ) ;
#45084=CARTESIAN_POINT ( 'NONE',  ( 69.68177367721139603, 20.52767805628179332, 41.38025477438755928 ) ) ;
#45089=EDGE_LOOP ( 'NONE', ( #61750, #63480, #36443, #54217 ) ) ;
#45090=FACE_OUTER_BOUND ( 'NONE', #63675, .T. ) ;
#45096=ORIENTED_EDGE ( 'NONE', *, *, #41921, .T. ) ;
#45101=EDGE_CURVE ( 'NONE', #34747, #54206, #64724, .T. ) ;
#45103=ORIENTED_EDGE ( 'NONE', *, *, #43225, .T. ) ;
#45107=CONICAL_SURFACE ( 'NONE', #36130, 74.95140232871122521, 0.8777644062502172329 ) ;
#45111=CONICAL_SURFACE ( 'NONE', #20411, 74.95140232871122521, 0.8777644062502172329 ) ;
#45123=CARTESIAN_POINT ( 'NONE',  ( -8.651394039243120559, 32.28678488987412010, 6.893342931991233158 ) ) ;
#45127=EDGE_CURVE ( 'NONE', #67017, #42777, #28249, .T. ) ;
#45131=DIRECTION ( 'NONE',  ( 1.000000000000000000, 0.000000000000000000, 0.000000000000000000 ) ) ;
#45133=ORIENTED_EDGE ( 'NONE', *, *, #58910, .T. ) ;
#45135=VERTEX_POINT ( 'NONE', #39175 ) ;
#45136=ORIENTED_EDGE ( 'NONE', *, *, #59414, .F. ) ;
#45137=CARTESIAN_POINT ( 'NONE',  ( 0.000000000000000000, 0.000000000000000000, 170.0000000000000000 ) ) ;
#45141=B_SPLINE_CURVE_WITH_KNOTS ( 'NONE', 3,
 ( #9263, #8926, #51496, #52514, #20162, #30374 ),
 .UNSPECIFIED., .F., .F.,
 ( 4, 2, 4 ),
 ( 1.095770181088879689E-06, 0.03239442681617710207, 0.06478775786217311206 ),
 .UNSPECIFIED. ) ;
#45149=CARTESIAN_POINT ( 'NONE',  ( -30.60309003827974550, 68.41902945196812880, 41.38025477438755928 ) ) ;
#45166=FACE_OUTER_BOUND ( 'NONE', #62501, .T. ) ;
#45170=AXIS2_PLACEMENT_3D ( 'NONE', #54434, #32998, #55139 ) ;
#45171=CARTESIAN_POINT ( 'NONE',  ( 0.000000000000000000, 0.000000000000000000, 41.38025477438755928 ) ) ;
#45176=DIRECTION ( 'NONE',  ( -0.000000000000000000, -0.000000000000000000, 1.000000000000000000 ) ) ;
#45181=ADVANCED_FACE ( 'NONE', ( #19088 ), #63036, .T. ) ;
#45197=LINE ( 'NONE', #13878, #6182 ) ;
#45210=CARTESIAN_POINT ( 'NONE',  ( 45.78444578631987127, 59.41672343742573759, 170.0000000000000000 ) ) ;
#45219=PLANE ( 'NONE',  #55359 ) ;
#45220=ORIENTED_EDGE ( 'NONE', *, *, #44553, .T. ) ;
#45229=CARTESIAN_POINT ( 'NONE',  ( 24.91130694661015710, -3.250319586706349018, 3.061616997868437868E-16 ) ) ;
#45248=DIRECTION ( 'NONE',  ( -0.000000000000000000, 0.000000000000000000, -1.000000000000000000 ) ) ;
#45250=EDGE_CURVE ( 'NONE', #59881, #56091, #30343, .T. ) ;
#45254=VERTEX_POINT ( 'NONE', #62704 ) ;
#45255=CONICAL_SURFACE ( 'NONE', #67717, 65.00000000000000000, 0.7853981633974497223 ) ;
#45260=DIRECTION ( 'NONE',  ( -2.298858655265465393E-16, 9.825793442285913883E-17, 1.000000000000000000 ) ) ;
#45265=AXIS2_PLACEMENT_3D ( 'NONE', #14879, #68021, #46899 ) ;
#45268=EDGE_CURVE ( 'NONE', #22952, #37048, #45650, .T. ) ;
#45294=AXIS2_PLACEMENT_3D ( 'NONE', #9016, #58552, #51911 ) ;
#45298=ORIENTED_EDGE ( 'NONE', *, *, #10246, .F. ) ;
#45301=VECTOR ( 'NONE', #759, 1000.000000000000000 ) ;
#45325=CARTESIAN_POINT ( 'NONE',  ( -6.774725108395958983, 24.06456107444435233, 0.000000000000000000 ) ) ;
#45326=EDGE_CURVE ( 'NONE', #48528, #55351, #55745, .T. ) ;
#45330=ORIENTED_EDGE ( 'NONE', *, *, #5150, .T. ) ;
#45334=ORIENTED_EDGE ( 'NONE', *, *, #8129, .F. ) ;
#45340=EDGE_CURVE ( 'NONE', #25681, #60309, #25767, .T. ) ;
#45342=ORIENTED_EDGE ( 'NONE', *, *, #11125, .F. ) ;
#45356=ORIENTED_EDGE ( 'NONE', *, *, #10683, .T. ) ;
#45359=CARTESIAN_POINT ( 'NONE',  ( -60.41792053122281914, 24.01035990323430624, 170.0000000000000000 ) ) ;
#45364=VECTOR ( 'NONE', #51723, 999.9999999999998863 ) ;
#45366=CIRCLE ( 'NONE', #27367, 65.00000000000000000 ) ;
#45371=VECTOR ( 'NONE', #4866, 1000.000000000000000 ) ;
#45375=CARTESIAN_POINT ( 'NONE',  ( 57.30278335769541087, 48.40406511297401693, 43.58025477438756212 ) ) ;
#45386=VERTEX_POINT ( 'NONE', #16914 ) ;
#45393=ADVANCED_FACE ( 'NONE', ( #27120 ), #16570, .T. ) ;
#45395=DIRECTION ( 'NONE',  ( -0.000000000000000000, -0.000000000000000000, 1.000000000000000000 ) ) ;
#45398=LINE ( 'NONE', #59823, #4049 ) ;
#45400=ORIENTED_EDGE ( 'NONE', *, *, #43446, .T. ) ;
#45401=CIRCLE ( 'NONE', #15076, 25.12245591505646303 ) ;
#45414=VERTEX_POINT ( 'NONE', #21496 ) ;
#45422=AXIS2_PLACEMENT_3D ( 'NONE', #69227, #42160, #21728 ) ;
#45433=EDGE_CURVE ( 'NONE', #28173, #60623, #26447, .T. ) ;
#45441=CARTESIAN_POINT ( 'NONE',  ( 35.43132383622789661, 14.63273331248878506, 13.32819299319723072 ) ) ;
#45447=ORIENTED_EDGE ( 'NONE', *, *, #64243, .F. ) ;
#45452=ORIENTED_EDGE ( 'NONE', *, *, #52356, .T. ) ;
#45457=ORIENTED_EDGE ( 'NONE', *, *, #56393, .T. ) ;
#45458=VECTOR ( 'NONE', #4835, 1000.000000000000114 ) ;
#45468=VERTEX_POINT ( 'NONE', #17979 ) ;
#45470=CARTESIAN_POINT ( 'NONE',  ( -10.50008313721455089, 40.38642104775755115, 13.79046412294882984 ) ) ;
#45480=EDGE_CURVE ( 'NONE', #28072, #13483, #48741, .T. ) ;
#45483=ORIENTED_EDGE ( 'NONE', *, *, #31596, .F. ) ;
#45485=LINE ( 'NONE', #56743, #608 ) ;
#45493=ADVANCED_FACE ( 'NONE', ( #17261 ), #66186, .T. ) ;
#45496=AXIS2_PLACEMENT_3D ( 'NONE', #57425, #30349, #9931 ) ;
#45499=CARTESIAN_POINT ( 'NONE',  ( -45.81425895439424067, 46.10914959592843587, 40.00000000000003553 ) ) ;
#45505=ORIENTED_EDGE ( 'NONE', *, *, #6745, .F. ) ;
#45520=ORIENTED_EDGE ( 'NONE', *, *, #20575, .F. ) ;
#45521=LINE ( 'NONE', #29692, #38317 ) ;
#45524=EDGE_CURVE ( 'NONE', #58687, #15601, #38733, .T. ) ;
#45525=LINE ( 'NONE', #55738, #39083 ) ;
#45532=ORIENTED_EDGE ( 'NONE', *, *, #67592, .F. ) ;
#45533=CARTESIAN_POINT ( 'NONE',  ( 61.91366885787729046, 28.42865614899000448, 43.58025477438756923 ) ) ;
#45535=CARTESIAN_POINT ( 'NONE',  ( 37.92109651401251114, 5.611248309713812610, 13.32819397642332859 ) ) ;
#45545=CARTESIAN_POINT ( 'NONE',  ( 29.69502258243350923, 57.82046033912877903, 40.00000000000003553 ) ) ;
#45553=DIRECTION ( 'NONE',  ( 1.000000000000000000, 0.000000000000000000, 0.000000000000000000 ) ) ;
#45555=VECTOR ( 'NONE', #22949, 1000.000000000000227 ) ;
#45556=ORIENTED_EDGE ( 'NONE', *, *, #63546, .F. ) ;
#45559=CARTESIAN_POINT ( 'NONE',  ( 0.000000000000000000, 0.000000000000000000, 40.00000000000003553 ) ) ;
#45561=AXIS2_PLACEMENT_3D ( 'NONE', #36042, #63119, #40971 ) ;
#45572=CARTESIAN_POINT ( 'NONE',  ( 19.00668540189186473, 62.54164772954719353, 41.38025477438755928 ) ) ;
#45573=PLANE ( 'NONE',  #18297 ) ;
#45583=ADVANCED_FACE ( 'NONE', ( #4222 ), #3874, .F. ) ;
#45597=CARTESIAN_POINT ( 'NONE',  ( 41.71033745877218735, 1.250000000000018652, 13.79046412284416867 ) ) ;
#45599=DIRECTION ( 'NONE',  ( -0.000000000000000000, 0.000000000000000000, -1.000000000000000000 ) ) ;
#45604=AXIS2_PLACEMENT_3D ( 'NONE', #49430, #63296, #4545 ) ;
#45610=EDGE_CURVE ( 'NONE', #7485, #49653, #8555, .T. ) ;
#45630=LINE ( 'NONE', #9377, #36226 ) ;
#45631=CARTESIAN_POINT ( 'NONE',  ( 0.000000000000000000, 0.000000000000000000, 41.38025477438755928 ) ) ;
#45637=VERTEX_POINT ( 'NONE', #20054 ) ;
#45644=CARTESIAN_POINT ( 'NONE',  ( 24.36509522349078338, -70.94296747916756374, 170.0000000000000000 ) ) ;
#45648=DIRECTION ( 'NONE',  ( -0.2225209339563042066, -0.9749279121818259508, 0.000000000000000000 ) ) ;
#45650=CIRCLE ( 'NONE', #1830, 25.12245591505646303 ) ;
#45663=CARTESIAN_POINT ( 'NONE',  ( -56.44201257846585662, -32.26641783793645857, 170.0000000000000000 ) ) ;
#45673=AXIS2_PLACEMENT_3D ( 'NONE', #17094, #22740, #40222 ) ;
#45679=EDGE_CURVE ( 'NONE', #50613, #34211, #27380, .T. ) ;
#45689=DIRECTION ( 'NONE',  ( 0.9959742939952382912, 0.08963930890344089242, -0.000000000000000000 ) ) ;
#45691=DIRECTION ( 'NONE',  ( -0.7227948638273878901, -0.6910626489868685329, 2.500042656554810833E-16 ) ) ;
#45702=EDGE_CURVE ( 'NONE', #54393, #47483, #47805, .T. ) ;
#45705=DIRECTION ( 'NONE',  ( -0.000000000000000000, -0.000000000000000000, -1.000000000000000000 ) ) ;
#45706=AXIS2_PLACEMENT_3D ( 'NONE', #58358, #53070, #10863 ) ;
#45714=DIRECTION ( 'NONE',  ( 1.000000000000000000, 0.000000000000000000, 0.000000000000000000 ) ) ;
#45716=ORIENTED_EDGE ( 'NONE', *, *, #15075, .T. ) ;
#45717=AXIS2_PLACEMENT_3D ( 'NONE', #34532, #8126, #7083 ) ;
#45723=EDGE_LOOP ( 'NONE', ( #43697, #26634, #12442, #58985 ) ) ;
#45726=DIRECTION ( 'NONE',  ( 0.8090169943749422332, 0.5877852522924802425, -0.000000000000000000 ) ) ;
#45728=ORIENTED_EDGE ( 'NONE', *, *, #67658, .F. ) ;
#45729=CARTESIAN_POINT ( 'NONE',  ( -64.83840629396345889, -4.580509716060185532, 170.0000000000000000 ) ) ;
#45730=ADVANCED_FACE ( 'NONE', ( #36919 ), #24330, .T. ) ;
#45732=CARTESIAN_POINT ( 'NONE',  ( 0.000000000000000000, 0.000000000000000000, 43.58025477438756212 ) ) ;
#45738=ORIENTED_EDGE ( 'NONE', *, *, #24400, .F. ) ;
#45739=DIRECTION ( 'NONE',  ( -0.5508969814521065267, 0.8345732537212999791, 0.000000000000000000 ) ) ;
#45741=ORIENTED_EDGE ( 'NONE', *, *, #13653, .F. ) ;
#45753=ORIENTED_EDGE ( 'NONE', *, *, #67944, .T. ) ;
#45760=CARTESIAN_POINT ( 'NONE',  ( -56.44201257846585662, -32.26641783793645857, 170.0000000000000000 ) ) ;
#45768=CARTESIAN_POINT ( 'NONE',  ( -24.53636015449789554, 60.58612729876395520, 43.58025477438756212 ) ) ;
#45787=CARTESIAN_POINT ( 'NONE',  ( -7.486743542470036594, 64.58150799671129505, 3.061616997868437868E-16 ) ) ;
#45788=CARTESIAN_POINT ( 'NONE',  ( 0.000000000000000000, 0.000000000000000000, 41.38025477438755928 ) ) ;
#45789=B_SPLINE_CURVE_WITH_KNOTS ( 'NONE', 3,
 ( #39975, #29423, #45597, #8672, #67082, #7280 ),
 .UNSPECIFIED., .F., .F.,
 ( 4, 2, 4 ),
 ( 0.03218932424835717343, 0.06469830966704906428, 0.09720729508574096900 ),
 .UNSPECIFIED. ) ;
#45794=CIRCLE ( 'NONE', #15466, 74.95140232871122521 ) ;
#45798=ORIENTED_EDGE ( 'NONE', *, *, #29372, .F. ) ;
#45806=VECTOR ( 'NONE', #12837, 1000.000000000000000 ) ;
#45807=ORIENTED_EDGE ( 'NONE', *, *, #17533, .T. ) ;
#45811=VERTEX_POINT ( 'NONE', #662 ) ;
#45814=CARTESIAN_POINT ( 'NONE',  ( 64.16679220703368003, 10.37413986118183828, 170.0000000000000000 ) ) ;
#45824=CARTESIAN_POINT ( 'NONE',  ( -11.76013739941318548, -57.14197750166816547, 27.58472369372398347 ) ) ;
#45830=LINE ( 'NONE', #4309, #34392 ) ;
#45837=ORIENTED_EDGE ( 'NONE', *, *, #60667, .F. ) ;
#45843=DIRECTION ( 'NONE',  ( 0.8584487936018728726, -0.5128992774058949156, 0.000000000000000000 ) ) ;
#45844=DIRECTION ( 'NONE',  ( 0.5128992774059071280, -0.8584487936018655452, 0.000000000000000000 ) ) ;
#45855=AXIS2_PLACEMENT_3D ( 'NONE', #27426, #14555, #21459 ) ;
#45864=CARTESIAN_POINT ( 'NONE',  ( 8.171862737214143024, -51.01496555961261237, 26.66469066592268078 ) ) ;
#45871=LINE ( 'NONE', #62040, #9165 ) ;
#45878=EDGE_CURVE ( 'NONE', #3054, #42365, #13529, .T. ) ;
#45889=DIRECTION ( 'NONE',  ( 0.04486483035051862939, -0.9989930665413143673, 0.000000000000000000 ) ) ;
#45893=CARTESIAN_POINT ( 'NONE',  ( -60.41792053122248518, -24.01035990323518021, 43.58025477438756923 ) ) ;
#45902=CARTESIAN_POINT ( 'NONE',  ( 23.05216796272336666, 9.986758404124199018, 3.061616997868437868E-16 ) ) ;
#45906=ORIENTED_EDGE ( 'NONE', *, *, #498, .T. ) ;
#45912=DIRECTION ( 'NONE',  ( 0.000000000000000000, 0.000000000000000000, 1.000000000000000000 ) ) ;
#45918=VERTEX_POINT ( 'NONE', #56914 ) ;
#45931=ORIENTED_EDGE ( 'NONE', *, *, #59368, .T. ) ;
#45936=LINE ( 'NONE', #67401, #35569 ) ;
#45948=LINE ( 'NONE', #7283, #54674 ) ;
#45951=ORIENTED_EDGE ( 'NONE', *, *, #56209, .T. ) ;
#45956=VECTOR ( 'NONE', #21131, 1000.000000000000114 ) ;
#45972=CARTESIAN_POINT ( 'NONE',  ( 0.000000000000000000, 0.000000000000000000, 43.58025477438756212 ) ) ;
#45974=DIRECTION ( 'NONE',  ( -0.4338837391175656699, 0.9009688679024155933, 0.000000000000000000 ) ) ;
#45975=EDGE_LOOP ( 'NONE', ( #33654, #39060, #16472, #17758 ) ) ;
#45998=EDGE_CURVE ( 'NONE', #62436, #10617, #47027, .T. ) ;
#46008=ORIENTED_EDGE ( 'NONE', *, *, #65129, .T. ) ;
#46014=FACE_OUTER_BOUND ( 'NONE', #27595, .T. ) ;
#46020=DIRECTION ( 'NONE',  ( -0.1785568947986229393, -0.9839295885986322210, 0.000000000000000000 ) ) ;
#46021=ORIENTED_EDGE ( 'NONE', *, *, #52002, .T. ) ;
#46026=CARTESIAN_POINT ( 'NONE',  ( -74.69807204964287450, -6.722948167758066695, 0.000000000000000000 ) ) ;
#46035=CARTESIAN_POINT ( 'NONE',  ( -40.53976144614951949, -9.891532800627171440, 13.79046340968177553 ) ) ;
#46041=CARTESIAN_POINT ( 'NONE',  ( -4.337405327941355360, 24.62086340933515416, 0.000000000000000000 ) ) ;
#46051=AXIS2_PLACEMENT_3D ( 'NONE', #59520, #11338, #54239 ) ;
#46059=ADVANCED_FACE ( 'NONE', ( #32252 ), #31552, .T. ) ;
#46068=LINE ( 'NONE', #66508, #28856 ) ;
#46070=PLANE ( 'NONE',  #21937 ) ;
#46091=CARTESIAN_POINT ( 'NONE',  ( -20.93485882276935328, -13.66498028065569059, 0.000000000000000000 ) ) ;
#46096=CARTESIAN_POINT ( 'NONE',  ( -7.486743542469089796, -64.58150799671139453, 41.38025477438755928 ) ) ;
#46107=CARTESIAN_POINT ( 'NONE',  ( -47.07758065111505630, -21.28397262622344499, 26.66469104408689361 ) ) ;
#46112=ORIENTED_EDGE ( 'NONE', *, *, #16639, .T. ) ;
#46113=LINE ( 'NONE', #13425, #26672 ) ;
#46122=EDGE_CURVE ( 'NONE', #68798, #68305, #44884, .T. ) ;
#46125=DIRECTION ( 'NONE',  ( 0.9362348706397369824, 0.3513748240813435175, 0.000000000000000000 ) ) ;
#46130=VECTOR ( 'NONE', #50957, 999.9999999999998863 ) ;
#46133=LINE ( 'NONE', #35592, #65135 ) ;
#46134=DIRECTION ( 'NONE',  ( 1.000000000000000000, 0.000000000000000000, 0.000000000000000000 ) ) ;
#46140=EDGE_CURVE ( 'NONE', #47483, #23762, #6199, .T. ) ;
#46142=EDGE_CURVE ( 'NONE', #34747, #49220, #27300, .T. ) ;
#46145=CYLINDRICAL_SURFACE ( 'NONE', #50571, 65.00000000000000000 ) ;
#46155=VERTEX_POINT ( 'NONE', #27651 ) ;
#46156=CIRCLE ( 'NONE', #47256, 24.99999999999985434 ) ;
#46159=AXIS2_PLACEMENT_3D ( 'NONE', #19142, #57136, #36017 ) ;
#46161=CARTESIAN_POINT ( 'NONE',  ( -61.41100614348687969, 43.07262267896646790, 170.0000000000000000 ) ) ;
#46170=ORIENTED_EDGE ( 'NONE', *, *, #33239, .T. ) ;
#46172=ORIENTED_EDGE ( 'NONE', *, *, #44852, .T. ) ;
#46175=FACE_OUTER_BOUND ( 'NONE', #17207, .T. ) ;
#46183=CARTESIAN_POINT ( 'NONE',  ( 0.000000000000000000, 0.000000000000000000, 170.0000000000000000 ) ) ;
#46187=CARTESIAN_POINT ( 'NONE',  ( -23.03840347525647658, 9.707315041312055470, 0.000000000000000000 ) ) ;
#46197=CARTESIAN_POINT ( 'NONE',  ( -14.86595946517991429, -20.25193917588099524, 0.000000000000000000 ) ) ;
#46199=ADVANCED_FACE ( 'NONE', ( #4320 ), #61419, .T. ) ;
#46201=DIRECTION ( 'NONE',  ( 1.000000000000000000, 0.000000000000000000, 0.000000000000000000 ) ) ;
#46204=ADVANCED_FACE ( 'NONE', ( #25089 ), #42292, .T. ) ;
#46219=CARTESIAN_POINT ( 'NONE',  ( 0.000000000000000000, 0.000000000000000000, 170.0000000000000000 ) ) ;
#46223=VERTEX_POINT ( 'NONE', #14522 ) ;
#46227=AXIS2_PLACEMENT_3D ( 'NONE', #49008, #60628, #32504 ) ;
#46239=CARTESIAN_POINT ( 'NONE',  ( 44.01696072965949469, 47.84694004974210912, 170.0000000000000000 ) ) ;
#46243=CARTESIAN_POINT ( 'NONE',  ( 4.360227497916021377, -41.50063969896140037, 13.79046340968177731 ) ) ;
#46254=AXIS2_PLACEMENT_3D ( 'NONE', #58829, #54941, #6760 ) ;
#46263=ORIENTED_EDGE ( 'NONE', *, *, #52387, .T. ) ;
#46267=VECTOR ( 'NONE', #17982, 1000.000000000000227 ) ;
#46271=LINE ( 'NONE', #57534, #51287 ) ;
#46278=EDGE_LOOP ( 'NONE', ( #15823, #34875, #53814, #57477, #11276, #36824, #4393, #3819, #10500 ) ) ;
#46279=CARTESIAN_POINT ( 'NONE',  ( 57.61205590192970050, -9.184630597077863001, 27.58472369370706545 ) ) ;
#46290=FACE_OUTER_BOUND ( 'NONE', #67928, .T. ) ;
#46291=CARTESIAN_POINT ( 'NONE',  ( -65.36598343705435354, 0.000000000000000000, 41.38025477438755928 ) ) ;
#46304=DIRECTION ( 'NONE',  ( -0.000000000000000000, -0.000000000000000000, -1.000000000000000000 ) ) ;
#46306=EDGE_CURVE ( 'NONE', #56091, #63790, #52155, .T. ) ;
#46310=CIRCLE ( 'NONE', #11443, 65.36598343705435354 ) ;
#46324=ORIENTED_EDGE ( 'NONE', *, *, #57657, .T. ) ;
#46342=VERTEX_POINT ( 'NONE', #52501 ) ;
#46351=CARTESIAN_POINT ( 'NONE',  ( -15.67984581961064450, 63.08044415722863363, 170.0000000000000000 ) ) ;
#46358=ORIENTED_EDGE ( 'NONE', *, *, #50280, .F. ) ;
#46363=EDGE_CURVE ( 'NONE', #4738, #59256, #20985, .T. ) ;
#46375=ADVANCED_FACE ( 'NONE', ( #26804 ), #42959, .T. ) ;
#46378=CYLINDRICAL_SURFACE ( 'NONE', #5185, 65.00000000000000000 ) ;
#46388=CARTESIAN_POINT ( 'NONE',  ( 61.28323125814129213, -21.66484633135379667, 170.0000000000000000 ) ) ;
#46404=LINE ( 'NONE', #2471, #54130 ) ;
#46407=LINE ( 'NONE', #55942, #47910 ) ;
#46414=AXIS2_PLACEMENT_3D ( 'NONE', #24764, #30039, #67677 ) ;
#46418=CARTESIAN_POINT ( 'NONE',  ( -62.97854483871577713, 16.08424353203677271, 40.00000000000003553 ) ) ;
#46435=ORIENTED_EDGE ( 'NONE', *, *, #18567, .F. ) ;
#46442=ORIENTED_EDGE ( 'NONE', *, *, #44709, .T. ) ;
#46449=CYLINDRICAL_SURFACE ( 'NONE', #61372, 65.00000000000000000 ) ;
#46454=EDGE_CURVE ( 'NONE', #2615, #68299, #67115, .T. ) ;
#46456=EDGE_LOOP ( 'NONE', ( #68789, #17181, #40869, #12776, #40987, #59863, #4113, #43549, #34383 ) ) ;
#46461=CONICAL_SURFACE ( 'NONE', #10499, 74.95140232871122521, 0.8777644062502172329 ) ;
#46468=DIRECTION ( 'NONE',  ( 0.000000000000000000, 0.000000000000000000, 1.000000000000000000 ) ) ;
#46476=EDGE_CURVE ( 'NONE', #64497, #695, #56959, .T. ) ;
#46477=DIRECTION ( 'NONE',  ( 0.000000000000000000, 0.000000000000000000, 1.000000000000000000 ) ) ;
#46480=ORIENTED_EDGE ( 'NONE', *, *, #6365, .T. ) ;
#46483=DIRECTION ( 'NONE',  ( -0.000000000000000000, -0.000000000000000000, -1.000000000000000000 ) ) ;
#46509=CARTESIAN_POINT ( 'NONE',  ( 25.09133896793783336, 1.250000000000021982, 3.061616997868437868E-16 ) ) ;
#46518=CONICAL_SURFACE ( 'NONE', #36480, 74.95140232871122521, 0.8777644062502172329 ) ;
#46531=VERTEX_POINT ( 'NONE', #55265 ) ;
#46535=CARTESIAN_POINT ( 'NONE',  ( 0.000000000000000000, 0.000000000000000000, 0.000000000000000000 ) ) ;
#46551=EDGE_LOOP ( 'NONE', ( #38177, #60608, #6699, #23141 ) ) ;
#46558=AXIS2_PLACEMENT_3D ( 'NONE', #2355, #45599, #65060 ) ;
#46565=EDGE_LOOP ( 'NONE', ( #48530, #29156, #41063, #42636 ) ) ;
#46568=DIRECTION ( 'NONE',  ( -0.7530714660036099684, -0.6579387259397138088, 0.000000000000000000 ) ) ;
#46573=CARTESIAN_POINT ( 'NONE',  ( 50.59696802070018151, -10.45241205790868477, 26.66469104408688295 ) ) ;
#46593=EDGE_CURVE ( 'NONE', #21766, #17523, #30222, .T. ) ;
#46599=LINE ( 'NONE', #13903, #50905 ) ;
#46620=CARTESIAN_POINT ( 'NONE',  ( 24.17157287525367693, 0.000000000000000000, 2.000000000000001776 ) ) ;
#46629=B_SPLINE_CURVE_WITH_KNOTS ( 'NONE', 3,
 ( #34393, #40679, #35414, #18544 ),
 .UNSPECIFIED., .F., .F.,
 ( 4, 4 ),
 ( 0.1259919275528356697, 0.1829744153748743274 ),
 .UNSPECIFIED. ) ;
#46631=CARTESIAN_POINT ( 'NONE',  ( 0.000000000000000000, 0.000000000000000000, 41.38025477438755928 ) ) ;
#46636=DIRECTION ( 'NONE',  ( -1.000000000000000000, 0.000000000000000000, 0.000000000000000000 ) ) ;
#46649=LINE ( 'NONE', #20265, #30456 ) ;
#46650=ORIENTED_EDGE ( 'NONE', *, *, #62017, .F. ) ;
#46662=CARTESIAN_POINT ( 'NONE',  ( 10.00000000000000000, 1.224646799147353256E-15, 2.000000000000001776 ) ) ;
#46667=ORIENTED_EDGE ( 'NONE', *, *, #11749, .F. ) ;
#46678=EDGE_CURVE ( 'NONE', #42865, #2737, #57355, .T. ) ;
#46695=ORIENTED_EDGE ( 'NONE', *, *, #40363, .F. ) ;
#46697=ORIENTED_EDGE ( 'NONE', *, *, #10246, .T. ) ;
#46698=AXIS2_PLACEMENT_3D ( 'NONE', #68410, #25163, #30777 ) ;
#46704=DIRECTION ( 'NONE',  ( 0.000000000000000000, 0.000000000000000000, 1.000000000000000000 ) ) ;
#46706=VECTOR ( 'NONE', #28538, 1000.000000000000114 ) ;
#46715=ORIENTED_EDGE ( 'NONE', *, *, #65101, .T. ) ;
#46727=CARTESIAN_POINT ( 'NONE',  ( -32.53122335971237788, -7.681316725934842715, 6.893343212288939093 ) ) ;
#46730=LINE ( 'NONE', #63263, #718 ) ;
#46746=ORIENTED_EDGE ( 'NONE', *, *, #58200, .T. ) ;
#46758=AXIS2_PLACEMENT_3D ( 'NONE', #42909, #11252, #37292 ) ;
#46761=EDGE_CURVE ( 'NONE', #68971, #2402, #22141, .T. ) ;
#46767=DIRECTION ( 'NONE',  ( -0.8090169943749422332, -0.5877852522924802425, 0.000000000000000000 ) ) ;
#46771=ORIENTED_EDGE ( 'NONE', *, *, #58535, .T. ) ;
#46790=DIRECTION ( 'NONE',  ( 0.000000000000000000, 0.000000000000000000, 1.000000000000000000 ) ) ;
#46803=FACE_OUTER_BOUND ( 'NONE', #40864, .T. ) ;
#46805=VECTOR ( 'NONE', #69264, 1000.000000000000000 ) ;
#46811=AXIS2_PLACEMENT_3D ( 'NONE', #30534, #24916, #3800 ) ;
#46812=EDGE_LOOP ( 'NONE', ( #26602, #13290, #24696, #65911 ) ) ;
#46817=ORIENTED_EDGE ( 'NONE', *, *, #20893, .T. ) ;
#46818=AXIS2_PLACEMENT_3D ( 'NONE', #21077, #15786, #26693 ) ;
#46821=DIRECTION ( 'NONE',  ( 0.000000000000000000, 0.000000000000000000, 1.000000000000000000 ) ) ;
#46822=CARTESIAN_POINT ( 'NONE',  ( 65.02478361689782105, -37.39438481343979959, 170.0000000000000000 ) ) ;
#46827=ORIENTED_EDGE ( 'NONE', *, *, #42167, .F. ) ;
#46828=CARTESIAN_POINT ( 'NONE',  ( 4.165045035621076863, -64.88046627338039229, 170.0000000000000000 ) ) ;
#46855=EDGE_CURVE ( 'NONE', #45414, #42599, #47758, .T. ) ;
#46857=CARTESIAN_POINT ( 'NONE',  ( 45.82394788922800899, 46.11928342727495078, 41.38025477438755928 ) ) ;
#46861=DIRECTION ( 'NONE',  ( -0.4338837391175525693, -0.9009688679024218105, 2.500042656554809354E-16 ) ) ;
#46870=VECTOR ( 'NONE', #27985, 1000.000000000000000 ) ;
#46877=DIRECTION ( 'NONE',  ( 0.000000000000000000, 0.000000000000000000, 1.000000000000000000 ) ) ;
#46897=PLANE ( 'NONE',  #22564 ) ;
#46898=VECTOR ( 'NONE', #46821, 1000.000000000000000 ) ;
#46899=DIRECTION ( 'NONE',  ( -1.000000000000000000, 0.000000000000000000, 0.000000000000000000 ) ) ;
#46903=LINE ( 'NONE', #19831, #53467 ) ;
#46906=CARTESIAN_POINT ( 'NONE',  ( 21.98745393275290638, -71.71550996510497100, 43.58025477438756212 ) ) ;
#46908=CARTESIAN_POINT ( 'NONE',  ( -71.96466849523078224, 21.15771699336999845, 43.58025477438756212 ) ) ;
#46909=FACE_OUTER_BOUND ( 'NONE', #1579, .T. ) ;
#46912=VECTOR ( 'NONE', #65901, 1000.000000000000114 ) ;
#46918=AXIS2_PLACEMENT_3D ( 'NONE', #48738, #11822, #27997 ) ;
#46919=ORIENTED_EDGE ( 'NONE', *, *, #58139, .F. ) ;
#46920=EDGE_CURVE ( 'NONE', #31642, #44050, #25621, .T. ) ;
#46926=DIRECTION ( 'NONE',  ( 0.3090169943749447312, 0.9510565162951545304, 0.000000000000000000 ) ) ;
#46943=VERTEX_POINT ( 'NONE', #31239 ) ;
#46947=DIRECTION ( 'NONE',  ( -1.000000000000000000, 0.000000000000000000, 0.000000000000000000 ) ) ;
#46950=FACE_OUTER_BOUND ( 'NONE', #49688, .T. ) ;
#46954=VERTEX_POINT ( 'NONE', #594 ) ;
#46958=DIRECTION ( 'NONE',  ( -0.000000000000000000, -0.000000000000000000, -1.000000000000000000 ) ) ;
#46961=VECTOR ( 'NONE', #34680, 1000.000000000000000 ) ;
#46967=ORIENTED_EDGE ( 'NONE', *, *, #49054, .T. ) ;
#46968=ORIENTED_EDGE ( 'NONE', *, *, #12395, .T. ) ;
#46969=AXIS2_PLACEMENT_3D ( 'NONE', #48384, #11123, #54012 ) ;
#46973=CYLINDRICAL_SURFACE ( 'NONE', #68578, 65.36598343705435354 ) ;
#46976=CARTESIAN_POINT ( 'NONE',  ( -2.116120943112233199, 74.98056102853672655, 73.58025477438756923 ) ) ;
#46979=PLANE ( 'NONE',  #5965 ) ;
#46993=ORIENTED_EDGE ( 'NONE', *, *, #37286, .T. ) ;
#46995=EDGE_CURVE ( 'NONE', #55150, #1969, #53350, .T. ) ;
#47001=EDGE_CURVE ( 'NONE', #20206, #6708, #53006, .T. ) ;
#47007=DIRECTION ( 'NONE',  ( 3.989004196750126251E-18, -3.181124695048441435E-18, -1.000000000000000000 ) ) ;
#47009=AXIS2_PLACEMENT_3D ( 'NONE', #6714, #26785, #28159 ) ;
#47011=CARTESIAN_POINT ( 'NONE',  ( 48.39383208188379371, 43.94028683479089636, 3.125053320693570118E-16 ) ) ;
#47013=CARTESIAN_POINT ( 'NONE',  ( 30.12852347772543027, -74.98256102853682137, 73.58025477438755502 ) ) ;
#47015=ORIENTED_EDGE ( 'NONE', *, *, #9957, .F. ) ;
#47018=ADVANCED_FACE ( 'NONE', ( #26642 ), #17633, .T. ) ;
#47021=EDGE_CURVE ( 'NONE', #22570, #2304, #44182, .T. ) ;
#47027=B_SPLINE_CURVE_WITH_KNOTS ( 'NONE', 3,
 ( #4137, #40036, #8024, #223 ),
 .UNSPECIFIED., .F., .F.,
 ( 4, 4 ),
 ( 9.900409499100981944E-07, 0.05658314289920114704 ),
 .UNSPECIFIED. ) ;
#47037=DIRECTION ( 'NONE',  ( -0.4738686624730094610, 0.8805955318567321166, 0.000000000000000000 ) ) ;
#47044=ORIENTED_EDGE ( 'NONE', *, *, #23180, .F. ) ;
#47048=FACE_OUTER_BOUND ( 'NONE', #2676, .T. ) ;
#47049=CARTESIAN_POINT ( 'NONE',  ( 19.00668540189274225, -62.54164772954691642, 41.38025477438755928 ) ) ;
#47050=CARTESIAN_POINT ( 'NONE',  ( -64.61430802170492882, 7.070445451047391749, 170.0000000000000000 ) ) ;
#47052=VECTOR ( 'NONE', #54332, 1000.000000000000227 ) ;
#47064=PLANE ( 'NONE',  #54724 ) ;
#47079=( LENGTH_UNIT ( ) NAMED_UNIT ( * ) SI_UNIT ( .MILLI., .METRE. ) );
#47080=EDGE_CURVE ( 'NONE', #20436, #65848, #945, .T. ) ;
#47089=VECTOR ( 'NONE', #68816, 1000.000000000000114 ) ;
#47103=VERTEX_POINT ( 'NONE', #50176 ) ;
#47105=LINE ( 'NONE', #43460, #6224 ) ;
#47111=ORIENTED_EDGE ( 'NONE', *, *, #32636, .T. ) ;
#47114=AXIS2_PLACEMENT_3D ( 'NONE', #53489, #21829, #736 ) ;
#47117=DIRECTION ( 'NONE',  ( 1.357354004350931427E-18, 4.918261777702530142E-18, -1.000000000000000000 ) ) ;
#47121=CARTESIAN_POINT ( 'NONE',  ( 42.52268486319166385, -51.31691592985912109, 34.48241824003540046 ) ) ;
#47122=CARTESIAN_POINT ( 'NONE',  ( -53.60725281709914469, 37.40286400928249577, 41.38025477438755928 ) ) ;
#47124=CARTESIAN_POINT ( 'NONE',  ( 19.00668540189185407, 62.54164772954719353, 43.58025477438756212 ) ) ;
#47129=DIRECTION ( 'NONE',  ( -0.000000000000000000, -0.000000000000000000, -1.000000000000000000 ) ) ;
#47134=EDGE_CURVE ( 'NONE', #40013, #12323, #25109, .T. ) ;
#47142=CARTESIAN_POINT ( 'NONE',  ( -36.84489839129265931, -53.54860840895233309, 40.00000000000003553 ) ) ;
#47144=AXIS2_PLACEMENT_3D ( 'NONE', #36299, #41916, #51448 ) ;
#47166=CARTESIAN_POINT ( 'NONE',  ( 64.16679220703369424, 10.37413986118183828, 40.00000000000003553 ) ) ;
#47168=VERTEX_POINT ( 'NONE', #22747 ) ;
#47171=LINE ( 'NONE', #61966, #34270 ) ;
#47173=ORIENTED_EDGE ( 'NONE', *, *, #33182, .F. ) ;
#47192=CARTESIAN_POINT ( 'NONE',  ( 0.000000000000000000, 0.000000000000000000, 0.000000000000000000 ) ) ;
#47195=FACE_OUTER_BOUND ( 'NONE', #20123, .T. ) ;
#47196=CARTESIAN_POINT ( 'NONE',  ( 36.64089410029661309, -65.45232906116366678, 170.0000000000000000 ) ) ;
#47206=DIRECTION ( 'NONE',  ( 0.000000000000000000, 0.000000000000000000, 1.000000000000000000 ) ) ;
#47214=ADVANCED_FACE ( 'NONE', ( #12199 ), #55091, .F. ) ;
#47219=ORIENTED_EDGE ( 'NONE', *, *, #62771, .T. ) ;
#47223=FACE_OUTER_BOUND ( 'NONE', #7494, .T. ) ;
#47226=CARTESIAN_POINT ( 'NONE',  ( 0.000000000000000000, 0.000000000000000000, 0.000000000000000000 ) ) ;
#47236=EDGE_CURVE ( 'NONE', #66025, #11003, #29079, .T. ) ;
#47244=CARTESIAN_POINT ( 'NONE',  ( 60.82895951008336510, 30.68107831874607072, 0.000000000000000000 ) ) ;
#47248=ORIENTED_EDGE ( 'NONE', *, *, #36950, .T. ) ;
#47251=CARTESIAN_POINT ( 'NONE',  ( -15.67984581961064450, 63.08044415722863363, 40.00000000000003553 ) ) ;
#47253=VERTEX_POINT ( 'NONE', #35388 ) ;
#47256=AXIS2_PLACEMENT_3D ( 'NONE', #53951, #5443, #65229 ) ;
#47267=ORIENTED_EDGE ( 'NONE', *, *, #63761, .F. ) ;
#47275=ORIENTED_EDGE ( 'NONE', *, *, #35419, .F. ) ;
#47276=ORIENTED_EDGE ( 'NONE', *, *, #24142, .F. ) ;
#47277=ORIENTED_EDGE ( 'NONE', *, *, #25645, .T. ) ;
#47281=DIRECTION ( 'NONE',  ( 0.000000000000000000, 0.000000000000000000, 1.000000000000000000 ) ) ;
#47291=CARTESIAN_POINT ( 'NONE',  ( -53.09243206623446554, 24.18057240364262128, 27.58472369387556355 ) ) ;
#47293=CARTESIAN_POINT ( 'NONE',  ( 61.28323125814100081, 21.66484633135460669, 40.00000000000003553 ) ) ;
#47297=ADVANCED_FACE ( 'NONE', ( #54918 ), #6743, .T. ) ;
#47302=CARTESIAN_POINT ( 'NONE',  ( 60.82895951008336510, 30.68107831874607072, 43.58025477438756923 ) ) ;
#47305=AXIS2_PLACEMENT_3D ( 'NONE', #12050, #17679, #54949 ) ;
#47306=DIRECTION ( 'NONE',  ( -1.000000000000000000, 0.000000000000000000, 0.000000000000000000 ) ) ;
#47311=EDGE_CURVE ( 'NONE', #22570, #21034, #50359, .T. ) ;
#47319=CARTESIAN_POINT ( 'NONE',  ( 0.000000000000000000, 0.000000000000000000, 0.000000000000000000 ) ) ;
#47325=ORIENTED_EDGE ( 'NONE', *, *, #69568, .F. ) ;
#47329=ORIENTED_EDGE ( 'NONE', *, *, #43084, .T. ) ;
#47337=CARTESIAN_POINT ( 'NONE',  ( -72.62976060914745347, 18.74780984163036024, 170.0000000000000000 ) ) ;
#47343=ORIENTED_EDGE ( 'NONE', *, *, #47311, .F. ) ;
#47344=ORIENTED_EDGE ( 'NONE', *, *, #2551, .F. ) ;
#47349=ORIENTED_EDGE ( 'NONE', *, *, #43014, .T. ) ;
#47351=VECTOR ( 'NONE', #50713, 1000.000000000000000 ) ;
#47352=DIRECTION ( 'NONE',  ( 0.000000000000000000, 0.000000000000000000, 1.000000000000000000 ) ) ;
#47358=LINE ( 'NONE', #20634, #63983 ) ;
#47359=CARTESIAN_POINT ( 'NONE',  ( -55.89173002820263036, 16.72186783039639124, 27.58472315868180402 ) ) ;
#47369=CARTESIAN_POINT ( 'NONE',  ( -67.03031041878467988, 33.66749151869449008, 170.0000000000000000 ) ) ;
#47379=EDGE_CURVE ( 'NONE', #11718, #18311, #45067, .T. ) ;
#47382=CARTESIAN_POINT ( 'NONE',  ( 55.04622734272535212, -19.32405960966675451, 27.58472369380034550 ) ) ;
#47388=ORIENTED_EDGE ( 'NONE', *, *, #10997, .T. ) ;
#47395=CARTESIAN_POINT ( 'NONE',  ( 0.000000000000000000, 0.000000000000000000, 41.38025477438755928 ) ) ;
#47418=CARTESIAN_POINT ( 'NONE',  ( 69.68177367721197868, -20.52767805628085895, 41.38025477438755928 ) ) ;
#47424=DIRECTION ( 'NONE',  ( -0.000000000000000000, -0.000000000000000000, -1.000000000000000000 ) ) ;
#47425=ORIENTED_EDGE ( 'NONE', *, *, #57514, .F. ) ;
#47436=CARTESIAN_POINT ( 'NONE',  ( -13.24252603915519444, -63.63674649211960599, 40.00000000000003553 ) ) ;
#47442=ORIENTED_EDGE ( 'NONE', *, *, #56064, .F. ) ;
#47443=DIRECTION ( 'NONE',  ( 1.000000000000000000, 0.000000000000000000, 0.000000000000000000 ) ) ;
#47444=ORIENTED_EDGE ( 'NONE', *, *, #3642, .T. ) ;
#47448=CARTESIAN_POINT ( 'NONE',  ( 55.61348889667009132, -50.24791103897046440, 41.38025477438755928 ) ) ;
#47454=CARTESIAN_POINT ( 'NONE',  ( 16.62148331457517969, -18.83783649008704586, 3.061616997868437868E-16 ) ) ;
#47455=EDGE_CURVE ( 'NONE', #49554, #65052, #27808, .T. ) ;
#47460=ADVANCED_FACE ( 'NONE', ( #55274 ), #18001, .F. ) ;
#47461=VERTEX_POINT ( 'NONE', #40834 ) ;
#47466=EDGE_CURVE ( 'NONE', #30492, #34240, #31818, .T. ) ;
#47471=DIRECTION ( 'NONE',  ( -1.000000000000000000, 0.000000000000000000, 0.000000000000000000 ) ) ;
#47477=CARTESIAN_POINT ( 'NONE',  ( 19.71799482800335923, -15.56722426018171035, 3.061616997868437868E-16 ) ) ;
#47483=VERTEX_POINT ( 'NONE', #20078 ) ;
#47485=DIRECTION ( 'NONE',  ( -0.000000000000000000, -0.000000000000000000, -1.000000000000000000 ) ) ;
#47495=LINE ( 'NONE', #58402, #7462 ) ;
#47500=LINE ( 'NONE', #4606, #37060 ) ;
#47505=ORIENTED_EDGE ( 'NONE', *, *, #2945, .T. ) ;
#47507=ORIENTED_EDGE ( 'NONE', *, *, #38854, .F. ) ;
#47508=VERTEX_POINT ( 'NONE', #68604 ) ;
#47519=CARTESIAN_POINT ( 'NONE',  ( 0.000000000000000000, 0.000000000000000000, 40.00000000000003553 ) ) ;
#47525=LINE ( 'NONE', #46161, #9875 ) ;
#47537=CARTESIAN_POINT ( 'NONE',  ( -10.27459178052906097, 50.63337688185094976, 26.66469104408689006 ) ) ;
#47539=DIRECTION ( 'NONE',  ( 0.000000000000000000, 0.000000000000000000, 1.000000000000000000 ) ) ;
#47542=VECTOR ( 'NONE', #66105, 1000.000000000000000 ) ;
#47543=CARTESIAN_POINT ( 'NONE',  ( -29.87147652227455552, -74.98256102853682137, 133.5802547743875550 ) ) ;
#47544=CARTESIAN_POINT ( 'NONE',  ( 24.34685647903079442, -70.88683439560421107, 41.38025477438755928 ) ) ;
#47545=EDGE_CURVE ( 'NONE', #60060, #68173, #18366, .T. ) ;
#47551=CARTESIAN_POINT ( 'NONE',  ( 13.56909401489541800, -65.06753427964257241, 133.5802547743875550 ) ) ;
#47552=CARTESIAN_POINT ( 'NONE',  ( 74.95140232871122521, 0.000000000000000000, 41.38025477438755928 ) ) ;
#47557=CARTESIAN_POINT ( 'NONE',  ( 0.000000000000000000, 0.000000000000000000, 41.38025477438755928 ) ) ;
#47562=VECTOR ( 'NONE', #19905, 999.9999999999998863 ) ;
#47571=CARTESIAN_POINT ( 'NONE',  ( 60.40479419793796012, -24.00543350795314979, 170.0000000000000000 ) ) ;
#47574=ORIENTED_EDGE ( 'NONE', *, *, #15554, .T. ) ;
#47581=ORIENTED_EDGE ( 'NONE', *, *, #20789, .F. ) ;
#47588=LINE ( 'NONE', #30749, #35522 ) ;
#47589=CARTESIAN_POINT ( 'NONE',  ( 31.89651141207536256, 56.63578868294628421, 170.0000000000000000 ) ) ;
#47602=CIRCLE ( 'NONE', #2698, 74.95140232871122521 ) ;
#47604=EDGE_CURVE ( 'NONE', #59849, #51881, #8283, .T. ) ;
#47606=CARTESIAN_POINT ( 'NONE',  ( 26.69682282325795697, -59.27986298182186431, 170.0000000000000000 ) ) ;
#47608=CARTESIAN_POINT ( 'NONE',  ( -65.36598343705435354, 0.000000000000000000, 41.38025477438755928 ) ) ;
#47609=LINE ( 'NONE', #16644, #58955 ) ;
#47610=DIRECTION ( 'NONE',  ( -0.08963930890342655666, -0.9959742939952397345, 2.500042656554808861E-16 ) ) ;
#47619=CARTESIAN_POINT ( 'NONE',  ( -24.02131556907225018, 34.12171082077519202, 13.79046412364926688 ) ) ;
#47624=DIRECTION ( 'NONE',  ( 1.000000000000000000, 0.000000000000000000, 0.000000000000000000 ) ) ;
#47627=EDGE_CURVE ( 'NONE', #22457, #15914, #68935, .T. ) ;
#47634=LINE ( 'NONE', #58204, #56203 ) ;
#47638=EDGE_LOOP ( 'NONE', ( #12130, #5394, #478, #3117, #31640, #63206, #4330, #5305, #38622, #28855, #38800, #57626, #65914, #20363, #21753, #13556, #4645, #32088, #5145, #2632, #43999, #69256, #8942 ) ) ;
#47640=DIRECTION ( 'NONE',  ( -0.9839295885986321100, 0.1785568947986229116, 0.000000000000000000 ) ) ;
#47643=EDGE_CURVE ( 'NONE', #50410, #9782, #7601, .T. ) ;
#47662=EDGE_LOOP ( 'NONE', ( #26056, #39023, #39960, #26245 ) ) ;
#47666=CARTESIAN_POINT ( 'NONE',  ( -35.66505502203998645, -56.29927565066983419, 34.48241823996503541 ) ) ;
#47670=ORIENTED_EDGE ( 'NONE', *, *, #20789, .T. ) ;
#47675=ORIENTED_EDGE ( 'NONE', *, *, #45524, .F. ) ;
#47678=FACE_OUTER_BOUND ( 'NONE', #31520, .T. ) ;
#47681=CARTESIAN_POINT ( 'NONE',  ( -64.18058723658641895, -10.37664328995269791, 3.061616997868437868E-16 ) ) ;
#47683=DIRECTION ( 'NONE',  ( -1.000000000000000000, 0.000000000000000000, 0.000000000000000000 ) ) ;
#47685=ORIENTED_EDGE ( 'NONE', *, *, #11568, .T. ) ;
#47688=VECTOR ( 'NONE', #11191, 1000.000000000000000 ) ;
#47692=LINE ( 'NONE', #60342, #20858 ) ;
#47696=B_SPLINE_CURVE_WITH_KNOTS ( 'NONE', 3,
 ( #33860, #23654, #67278, #7486, #50722, #18371 ),
 .UNSPECIFIED., .F., .F.,
 ( 4, 2, 4 ),
 ( 0.03218934490037906465, 0.06469832469447792112, 0.09720730448857675676 ),
 .UNSPECIFIED. ) ;
#47701=VECTOR ( 'NONE', #63537, 1000.000000000000227 ) ;
#47703=CARTESIAN_POINT ( 'NONE',  ( 70.65683382808231272, -25.18281821780013274, 170.0000000000000000 ) ) ;
#47712=CARTESIAN_POINT ( 'NONE',  ( -26.83517958587572494, -59.60356471962950309, 41.38025477438755928 ) ) ;
#47728=CARTESIAN_POINT ( 'NONE',  ( 53.32245423372616244, -37.19594572654634845, 170.0000000000000000 ) ) ;
#47740=ADVANCED_FACE ( 'NONE', ( #58219 ), #4412, .T. ) ;
#47741=FACE_OUTER_BOUND ( 'NONE', #42032, .T. ) ;
#47743=CARTESIAN_POINT ( 'NONE',  ( 55.65793654284612302, 50.28674377798304107, 170.0000000000000000 ) ) ;
#47745=VECTOR ( 'NONE', #53486, 1000.000000000000000 ) ;
#47747=VECTOR ( 'NONE', #25763, 1000.000000000000000 ) ;
#47758=B_SPLINE_CURVE_WITH_KNOTS ( 'NONE', 3,
 ( #8750, #19633, #41785, #61838 ),
 .UNSPECIFIED., .F., .F.,
 ( 4, 4 ),
 ( 9.900409499241261188E-07, 0.05658314289920116785 ),
 .UNSPECIFIED. ) ;
#47792=EDGE_CURVE ( 'NONE', #43717, #50848, #32186, .T. ) ;
#47796=EDGE_CURVE ( 'NONE', #27271, #68798, #7653, .T. ) ;
#47798=ORIENTED_EDGE ( 'NONE', *, *, #55044, .T. ) ;
#47799=CARTESIAN_POINT ( 'NONE',  ( -21.03405120204975276, 13.73704776265648775, 3.061616997868437868E-16 ) ) ;
#47802=AXIS2_PLACEMENT_3D ( 'NONE', #47395, #52347, #41107 ) ;
#47805=LINE ( 'NONE', #5582, #41188 ) ;
#47826=ORIENTED_EDGE ( 'NONE', *, *, #68753, .F. ) ;
#47829=CARTESIAN_POINT ( 'NONE',  ( 51.00231698266622260, -42.89951341137784624, 34.48241824007785539 ) ) ;
#47839=CARTESIAN_POINT ( 'NONE',  ( 0.000000000000000000, 0.000000000000000000, 43.58025477438756212 ) ) ;
#47840=DIRECTION ( 'NONE',  ( -0.000000000000000000, -0.000000000000000000, -1.000000000000000000 ) ) ;
#47845=DIRECTION ( 'NONE',  ( 0.000000000000000000, 0.000000000000000000, 1.000000000000000000 ) ) ;
#47861=ORIENTED_EDGE ( 'NONE', *, *, #38744, .F. ) ;
#47862=AXIS2_PLACEMENT_3D ( 'NONE', #6905, #54737, #13491 ) ;
#47863=EDGE_CURVE ( 'NONE', #58815, #41480, #64180, .T. ) ;
#47870=CARTESIAN_POINT ( 'NONE',  ( 60.82895951008428170, -30.68107831874537084, 170.0000000000000000 ) ) ;
#47872=CYLINDRICAL_SURFACE ( 'NONE', #47114, 65.00000000000000000 ) ;
#47884=CARTESIAN_POINT ( 'NONE',  ( 26.12852347772543737, 70.00000000000000000, 77.58025477438755502 ) ) ;
#47888=DIRECTION ( 'NONE',  ( 0.9510565162951544194, -0.3090169943749447312, 0.000000000000000000 ) ) ;
#47891=EDGE_LOOP ( 'NONE', ( #63573, #25417, #20567, #17203 ) ) ;
#47893=VERTEX_POINT ( 'NONE', #61347 ) ;
#47895=ORIENTED_EDGE ( 'NONE', *, *, #65597, .F. ) ;
#47899=CARTESIAN_POINT ( 'NONE',  ( -19.15041326417105338, -47.98507813326755667, 26.66469066592269144 ) ) ;
#47900=DIRECTION ( 'NONE',  ( 0.000000000000000000, 0.000000000000000000, 1.000000000000000000 ) ) ;
#47903=ORIENTED_EDGE ( 'NONE', *, *, #67800, .F. ) ;
#47910=VECTOR ( 'NONE', #34502, 999.9999999999998863 ) ;
#47911=CARTESIAN_POINT ( 'NONE',  ( 36.30976181811464443, 12.29214648180296088, 13.32819397642331971 ) ) ;
#47929=VERTEX_POINT ( 'NONE', #39543 ) ;
#47933=VECTOR ( 'NONE', #28016, 1000.000000000000000 ) ;
#47936=LINE ( 'NONE', #59182, #54579 ) ;
#47949=VECTOR ( 'NONE', #18244, 1000.000000000000000 ) ;
#47953=CARTESIAN_POINT ( 'NONE',  ( -66.97713359923356791, 33.64188291208976977, 41.38025477438755928 ) ) ;
#47961=VERTEX_POINT ( 'NONE', #7186 ) ;
#47962=B_SPLINE_CURVE_WITH_KNOTS ( 'NONE', 3,
 ( #57605, #19265, #30874, #68168, #40718, #35101 ),
 .UNSPECIFIED., .F., .F.,
 ( 4, 2, 4 ),
 ( 1.095770181093909371E-06, 0.03239442681617710207, 0.06478775786217311206 ),
 .UNSPECIFIED. ) ;
#47971=VERTEX_POINT ( 'NONE', #28644 ) ;
#47973=CARTESIAN_POINT ( 'NONE',  ( 0.000000000000000000, 0.000000000000000000, 41.38025477438755928 ) ) ;
#47978=CARTESIAN_POINT ( 'NONE',  ( -18.15845058245960075, 17.18344181019522310, 0.000000000000000000 ) ) ;
#47983=ORIENTED_EDGE ( 'NONE', *, *, #67817, .F. ) ;
#48006=DIRECTION ( 'NONE',  ( -1.000000000000000000, 0.000000000000000000, 0.000000000000000000 ) ) ;
#48012=VERTEX_POINT ( 'NONE', #68360 ) ;
#48017=EDGE_CURVE ( 'NONE', #18311, #67396, #45141, .T. ) ;
#48022=LINE ( 'NONE', #42750, #59792 ) ;
#48024=EDGE_CURVE ( 'NONE', #16, #26782, #6528, .T. ) ;
#48028=DIRECTION ( 'NONE',  ( -0.000000000000000000, -0.000000000000000000, -1.000000000000000000 ) ) ;
#48034=ADVANCED_FACE ( 'NONE', ( #63072 ), #68019, .T. ) ;
#48041=EDGE_CURVE ( 'NONE', #31287, #28747, #14876, .T. ) ;
#48059=LINE ( 'NONE', #37864, #38526 ) ;
#48067=PLANE ( 'NONE',  #14194 ) ;
#48072=LINE ( 'NONE', #10109, #41043 ) ;
#48082=DIRECTION ( 'NONE',  ( -0.000000000000000000, -0.000000000000000000, -1.000000000000000000 ) ) ;
#48100=EDGE_CURVE ( 'NONE', #63790, #36305, #15583, .T. ) ;
#48110=VERTEX_POINT ( 'NONE', #28200 ) ;
#48134=DIRECTION ( 'NONE',  ( 1.000000000000000000, 0.000000000000000000, 0.000000000000000000 ) ) ;
#48137=DIRECTION ( 'NONE',  ( 1.000000000000000000, 0.000000000000000000, -0.000000000000000000 ) ) ;
#48151=DIRECTION ( 'NONE',  ( 0.000000000000000000, 0.000000000000000000, 1.000000000000000000 ) ) ;
#48167=ORIENTED_EDGE ( 'NONE', *, *, #60038, .F. ) ;
#48171=CARTESIAN_POINT ( 'NONE',  ( -66.25334388784037287, 7.217961348991855708, 34.48241795236665297 ) ) ;
#48175=DIRECTION ( 'NONE',  ( -0.3090169943749447312, -0.9510565162951544194, 0.000000000000000000 ) ) ;
#48177=VECTOR ( 'NONE', #36022, 1000.000000000000000 ) ;
#48204=PLANE ( 'NONE',  #34588 ) ;
#48209=CIRCLE ( 'NONE', #54959, 25.12245591505646303 ) ;
#48211=FACE_OUTER_BOUND ( 'NONE', #9435, .T. ) ;
#48225=CARTESIAN_POINT ( 'NONE',  ( -58.00979178563811445, -29.32343869649178814, 40.00000000000003553 ) ) ;
#48236=CARTESIAN_POINT ( 'NONE',  ( -15.47041015649658391, 73.39774458108210808, 170.0000000000000000 ) ) ;
#48238=ORIENTED_EDGE ( 'NONE', *, *, #37626, .F. ) ;
#48250=DIRECTION ( 'NONE',  ( 0.8584487936018655452, 0.5128992774059070170, 0.000000000000000000 ) ) ;
#48262=CARTESIAN_POINT ( 'NONE',  ( -34.79003333406912901, 38.19633060033950755, 26.66469104408690427 ) ) ;
#48272=DIRECTION ( 'NONE',  ( 0.000000000000000000, 0.000000000000000000, 1.000000000000000000 ) ) ;
#48287=CARTESIAN_POINT ( 'NONE',  ( 11.51073125898252947, 31.38130312474459416, 6.893343212288933763 ) ) ;
#48290=EDGE_LOOP ( 'NONE', ( #47685, #54321, #17592, #10834 ) ) ;
#48296=FACE_OUTER_BOUND ( 'NONE', #48290, .T. ) ;
#48310=DIRECTION ( 'NONE',  ( 4.852411958229186445E-18, -1.576644219464734062E-18, -1.000000000000000000 ) ) ;
#48327=DIRECTION ( 'NONE',  ( -0.000000000000000000, -0.000000000000000000, -1.000000000000000000 ) ) ;
#48334=CARTESIAN_POINT ( 'NONE',  ( -1.666933348992582609, 64.97862212458815634, 170.0000000000000000 ) ) ;
#48347=AXIS2_PLACEMENT_3D ( 'NONE', #39405, #49948, #12674 ) ;
#48351=LINE ( 'NONE', #31521, #900 ) ;
#48352=CARTESIAN_POINT ( 'NONE',  ( -58.00979178563811445, -29.32343869649178814, 40.00000000000003553 ) ) ;
#48354=LINE ( 'NONE', #37134, #10557 ) ;
#48355=AXIS2_PLACEMENT_3D ( 'NONE', #54745, #43836, #64971 ) ;
#48361=ORIENTED_EDGE ( 'NONE', *, *, #59719, .F. ) ;
#48363=CARTESIAN_POINT ( 'NONE',  ( -52.69240448066584293, -53.30312580971443026, 41.38025477438755928 ) ) ;
#48369=CARTESIAN_POINT ( 'NONE',  ( -24.98026281234600887, 0.9932118737287082277, 0.000000000000000000 ) ) ;
#48376=DIRECTION ( 'NONE',  ( -0.000000000000000000, -0.000000000000000000, -1.000000000000000000 ) ) ;
#48380=ORIENTED_EDGE ( 'NONE', *, *, #61150, .F. ) ;
#48383=CARTESIAN_POINT ( 'NONE',  ( 69.68177367721199289, -20.52767805628082698, 170.0000000000000000 ) ) ;
#48384=CARTESIAN_POINT ( 'NONE',  ( 0.000000000000000000, 0.000000000000000000, 40.00000000000003553 ) ) ;
#48387=CIRCLE ( 'NONE', #33823, 74.95140232871122521 ) ;
#48398=VECTOR ( 'NONE', #12111, 1000.000000000000000 ) ;
#48402=DIRECTION ( 'NONE',  ( -1.644874880248581709E-16, -1.882710788443314728E-16, 1.000000000000000000 ) ) ;
#48408=CARTESIAN_POINT ( 'NONE',  ( -61.36325649057843634, 43.03793052543095854, 41.38025477438755928 ) ) ;
#48419=VERTEX_POINT ( 'NONE', #60129 ) ;
#48422=LINE ( 'NONE', #49476, #37658 ) ;
#48432=VERTEX_POINT ( 'NONE', #50286 ) ;
#48433=CARTESIAN_POINT ( 'NONE',  ( 70.34686579112866411, -18.11777090454118877, 0.000000000000000000 ) ) ;
#48436=CARTESIAN_POINT ( 'NONE',  ( -31.73109720166984715, 21.50890660541002219, 13.32819299319723072 ) ) ;
#48442=CIRCLE ( 'NONE', #18166, 24.99999999999985434 ) ;
#48454=FACE_OUTER_BOUND ( 'NONE', #46565, .T. ) ;
#48459=ORIENTED_EDGE ( 'NONE', *, *, #58656, .T. ) ;
#48472=ADVANCED_FACE ( 'NONE', ( #68539 ), #24941, .T. ) ;
#48473=ORIENTED_EDGE ( 'NONE', *, *, #66109, .T. ) ;
#48487=ORIENTED_EDGE ( 'NONE', *, *, #35664, .T. ) ;
#48491=EDGE_LOOP ( 'NONE', ( #28719, #9981, #66679, #26567 ) ) ;
#48507=CARTESIAN_POINT ( 'NONE',  ( 8.904582680623983393, 23.36040254969773144, 0.000000000000000000 ) ) ;
#48513=CARTESIAN_POINT ( 'NONE',  ( 70.34686579112866411, -18.11777090454118877, 170.0000000000000000 ) ) ;
#48517=VERTEX_POINT ( 'NONE', #63609 ) ;
#48524=ORIENTED_EDGE ( 'NONE', *, *, #35664, .F. ) ;
#48526=ORIENTED_EDGE ( 'NONE', *, *, #8502, .T. ) ;
#48528=VERTEX_POINT ( 'NONE', #37905 ) ;
#48530=ORIENTED_EDGE ( 'NONE', *, *, #25030, .T. ) ;
#48532=CARTESIAN_POINT ( 'NONE',  ( -49.77357484059193382, 41.82599373102802787, 170.0000000000000000 ) ) ;
#48535=ORIENTED_EDGE ( 'NONE', *, *, #51461, .T. ) ;
#48537=VECTOR ( 'NONE', #16119, 1000.000000000000000 ) ;
#48542=DIRECTION ( 'NONE',  ( -0.000000000000000000, -0.000000000000000000, -1.000000000000000000 ) ) ;
#48545=DIRECTION ( 'NONE',  ( -0.000000000000000000, -0.000000000000000000, 1.000000000000000000 ) ) ;
#48548=VECTOR ( 'NONE', #9385, 1000.000000000000114 ) ;
#48558=FACE_OUTER_BOUND ( 'NONE', #55837, .T. ) ;
#48565=CARTESIAN_POINT ( 'NONE',  ( -33.97701964160389565, -17.74986561234010551, 13.32819299319722894 ) ) ;
#48573=DIRECTION ( 'NONE',  ( -1.000000000000000000, 0.000000000000000000, 0.000000000000000000 ) ) ;
#48589=AXIS2_PLACEMENT_3D ( 'NONE', #40635, #63142, #51887 ) ;
#48600=CARTESIAN_POINT ( 'NONE',  ( 8.820885042877430138, 74.43053605947413587, 41.38025477438755928 ) ) ;
#48612=CARTESIAN_POINT ( 'NONE',  ( -1.068536314442417146, 51.65427688837380060, 26.66469104408687230 ) ) ;
#48619=CARTESIAN_POINT ( 'NONE',  ( 64.16679220703369424, 10.37413986118183828, 170.0000000000000000 ) ) ;
#48620=EDGE_CURVE ( 'NONE', #55364, #12081, #21377, .T. ) ;
#48637=LINE ( 'NONE', #65198, #19918 ) ;
#48640=EDGE_CURVE ( 'NONE', #3417, #43209, #32630, .T. ) ;
#48645=ORIENTED_EDGE ( 'NONE', *, *, #14894, .T. ) ;
#48648=ORIENTED_EDGE ( 'NONE', *, *, #33742, .F. ) ;
#48655=LINE ( 'NONE', #16325, #43589 ) ;
#48673=CARTESIAN_POINT ( 'NONE',  ( 23.93060502292685499, -7.646171227524485303, 3.061616997868437868E-16 ) ) ;
#48675=DIRECTION ( 'NONE',  ( -1.000000000000000000, 0.000000000000000000, 0.000000000000000000 ) ) ;
#48679=AXIS2_PLACEMENT_3D ( 'NONE', #813, #65895, #39154 ) ;
#48680=ORIENTED_EDGE ( 'NONE', *, *, #17155, .F. ) ;
#48682=PLANE ( 'NONE',  #54009 ) ;
#48694=ORIENTED_EDGE ( 'NONE', *, *, #40056, .T. ) ;
#48697=DIRECTION ( 'NONE',  ( -0.000000000000000000, -0.000000000000000000, -1.000000000000000000 ) ) ;
#48698=ORIENTED_EDGE ( 'NONE', *, *, #36122, .F. ) ;
#48714=LINE ( 'NONE', #6530, #35861 ) ;
#48718=VERTEX_POINT ( 'NONE', #25978 ) ;
#48724=CARTESIAN_POINT ( 'NONE',  ( 48.11816970607299027, -43.69944786993949748, 40.00000000000003553 ) ) ;
#48727=CIRCLE ( 'NONE', #26327, 65.00000000000000000 ) ;
#48728=CARTESIAN_POINT ( 'NONE',  ( 11.30618213853385967, 74.15344055032308290, 133.5802547743875550 ) ) ;
#48734=EDGE_CURVE ( 'NONE', #8790, #66330, #4857, .T. ) ;
#48735=AXIS2_PLACEMENT_3D ( 'NONE', #36766, #58211, #57186 ) ;
#48738=CARTESIAN_POINT ( 'NONE',  ( 0.000000000000000000, 0.000000000000000000, 41.38025477438755928 ) ) ;
#48740=VECTOR ( 'NONE', #63336, 1000.000000000000000 ) ;
#48741=B_SPLINE_CURVE_WITH_KNOTS ( 'NONE', 3,
 ( #2150, #49972, #12348, #7068 ),
 .UNSPECIFIED., .F., .F.,
 ( 4, 4 ),
 ( 0.1259919275528358917, 0.1829744153748748825 ),
 .UNSPECIFIED. ) ;
#48742=CARTESIAN_POINT ( 'NONE',  ( -53.31111153860302210, 37.18770477615724701, 170.0000000000000000 ) ) ;
#48748=ORIENTED_EDGE ( 'NONE', *, *, #12613, .F. ) ;
#48749=AXIS2_PLACEMENT_3D ( 'NONE', #25654, #25309, #24959 ) ;
#48753=VECTOR ( 'NONE', #50992, 1000.000000000000227 ) ;
#48758=DIRECTION ( 'NONE',  ( -0.000000000000000000, -0.000000000000000000, 1.000000000000000000 ) ) ;
#48759=CARTESIAN_POINT ( 'NONE',  ( -24.39249304643438521, 60.24953346690454481, 40.00000000000003553 ) ) ;
#48767=DIRECTION ( 'NONE',  ( -0.6910626489868580968, -0.7227948638273978821, 0.000000000000000000 ) ) ;
#48769=B_SPLINE_CURVE_WITH_KNOTS ( 'NONE', 3,
 ( #57197, #56492, #13253, #46279, #40660, #3046 ),
 .UNSPECIFIED., .F., .F.,
 ( 4, 2, 4 ),
 ( 0.03218933327099851582, 0.06469831623231186990, 0.09720729919362522398 ),
 .UNSPECIFIED. ) ;
#48782=VECTOR ( 'NONE', #5985, 1000.000000000000114 ) ;
#48784=EDGE_LOOP ( 'NONE', ( #7747, #39531, #50225, #18731 ) ) ;
#48790=VECTOR ( 'NONE', #66386, 1000.000000000000114 ) ;
#48792=CIRCLE ( 'NONE', #57819, 74.95140232871122521 ) ;
#48807=DIRECTION ( 'NONE',  ( 0.000000000000000000, 0.000000000000000000, -1.000000000000000000 ) ) ;
#48812=EDGE_CURVE ( 'NONE', #64523, #67945, #43859, .T. ) ;
#48819=LINE ( 'NONE', #68911, #4495 ) ;
#48820=CARTESIAN_POINT ( 'NONE',  ( 23.17627457812186620, -71.32923872213625316, 43.58025477438756212 ) ) ;
#48821=DIRECTION ( 'NONE',  ( -0.000000000000000000, -0.000000000000000000, -1.000000000000000000 ) ) ;
#48825=CIRCLE ( 'NONE', #18543, 65.00000000000000000 ) ;
#48835=CARTESIAN_POINT ( 'NONE',  ( 0.000000000000000000, 0.000000000000000000, 41.38025477438755928 ) ) ;
#48838=VECTOR ( 'NONE', #11494, 1000.000000000000000 ) ;
#48841=PLANE ( 'NONE',  #13894 ) ;
#48845=VECTOR ( 'NONE', #11095, 1000.000000000000000 ) ;
#48849=AXIS2_PLACEMENT_3D ( 'NONE', #9702, #25199, #4418 ) ;
#48850=FACE_OUTER_BOUND ( 'NONE', #4917, .T. ) ;
#48851=ORIENTED_EDGE ( 'NONE', *, *, #42413, .F. ) ;
#48854=VERTEX_POINT ( 'NONE', #6234 ) ;
#48859=DIRECTION ( 'NONE',  ( -4.691548276051970363E-18, 2.005263967813451899E-18, -1.000000000000000000 ) ) ;
#48862=EDGE_CURVE ( 'NONE', #18218, #27522, #17784, .T. ) ;
#48864=ORIENTED_EDGE ( 'NONE', *, *, #28577, .F. ) ;
#48867=DIRECTION ( 'NONE',  ( -0.2660368455666826670, 0.9639628606958513535, 0.000000000000000000 ) ) ;
#48874=EDGE_LOOP ( 'NONE', ( #61109, #30318, #43420, #58042 ) ) ;
#48877=ORIENTED_EDGE ( 'NONE', *, *, #6259, .F. ) ;
#48882=EDGE_CURVE ( 'NONE', #7248, #7351, #62795, .T. ) ;
#48888=CARTESIAN_POINT ( 'NONE',  ( 56.74421265833558436, 32.44697398030906044, 41.38025477438755928 ) ) ;
#48893=FACE_OUTER_BOUND ( 'NONE', #1032, .T. ) ;
#48897=ADVANCED_FACE ( 'NONE', ( #26488 ), #50889, .T. ) ;
#48908=CYLINDRICAL_SURFACE ( 'NONE', #33836, 65.00000000000000000 ) ;
#48911=LINE ( 'NONE', #31716, #16823 ) ;
#48920=CARTESIAN_POINT ( 'NONE',  ( -61.41100614348687969, 43.07262267896646790, 170.0000000000000000 ) ) ;
#48929=EDGE_LOOP ( 'NONE', ( #64148, #4129, #23650, #26307 ) ) ;
#48949=EDGE_CURVE ( 'NONE', #57856, #12108, #42658, .T. ) ;
#48964=EDGE_LOOP ( 'NONE', ( #62920, #66463, #63961, #2810 ) ) ;
#48967=DIRECTION ( 'NONE',  ( -0.6579387259397027066, -0.7530714660036196273, 0.000000000000000000 ) ) ;
#48973=ORIENTED_EDGE ( 'NONE', *, *, #47021, .T. ) ;
#48980=AXIS2_PLACEMENT_3D ( 'NONE', #40808, #51025, #30610 ) ;
#48994=DIRECTION ( 'NONE',  ( 0.000000000000000000, 0.000000000000000000, -1.000000000000000000 ) ) ;
#49001=DIRECTION ( 'NONE',  ( 1.000000000000000000, -1.243449787580175325E-14, 0.000000000000000000 ) ) ;
#49004=DIRECTION ( 'NONE',  ( -0.9510565162951545304, 0.3090169943749447312, 2.500042656554810833E-16 ) ) ;
#49007=CARTESIAN_POINT ( 'NONE',  ( -39.55079474733624068, -51.59997227571039957, 43.58025477438756923 ) ) ;
#49008=CARTESIAN_POINT ( 'NONE',  ( -60.67627457812130132, 44.08389392193514311, 0.000000000000000000 ) ) ;
#49014=ORIENTED_EDGE ( 'NONE', *, *, #5096, .T. ) ;
#49015=ORIENTED_EDGE ( 'NONE', *, *, #68529, .F. ) ;
#49017=DIRECTION ( 'NONE',  ( 0.1342332658176667304, -0.9909497617679331460, 0.000000000000000000 ) ) ;
#49031=DIRECTION ( 'NONE',  ( -0.000000000000000000, -0.000000000000000000, 1.000000000000000000 ) ) ;
#49032=DIRECTION ( 'NONE',  ( -1.000000000000000000, 0.000000000000000000, 0.000000000000000000 ) ) ;
#49049=DIRECTION ( 'NONE',  ( 0.000000000000000000, 0.000000000000000000, 1.000000000000000000 ) ) ;
#49054=EDGE_CURVE ( 'NONE', #45414, #32511, #22590, .T. ) ;
#49071=ORIENTED_EDGE ( 'NONE', *, *, #39661, .T. ) ;
#49075=AXIS2_PLACEMENT_3D ( 'NONE', #23304, #56336, #29264 ) ;
#49090=FACE_OUTER_BOUND ( 'NONE', #40032, .T. ) ;
#49101=AXIS2_PLACEMENT_3D ( 'NONE', #30086, #25849, #3685 ) ;
#49102=FACE_OUTER_BOUND ( 'NONE', #12428, .T. ) ;
#49108=CARTESIAN_POINT ( 'NONE',  ( -17.90772993695113868, 72.84144224619130625, 170.0000000000000000 ) ) ;
#49109=CARTESIAN_POINT ( 'NONE',  ( -41.21054144751222026, -41.29403858773821412, 27.58472315868181113 ) ) ;
#49111=ORIENTED_EDGE ( 'NONE', *, *, #56193, .F. ) ;
#49118=EDGE_CURVE ( 'NONE', #65787, #1572, #58828, .T. ) ;
#49121=ADVANCED_FACE ( 'NONE', ( #28567 ), #50712, .F. ) ;
#49135=EDGE_CURVE ( 'NONE', #6327, #56020, #34895, .T. ) ;
#49136=DIRECTION ( 'NONE',  ( -0.000000000000000000, -0.000000000000000000, -1.000000000000000000 ) ) ;
#49140=VECTOR ( 'NONE', #35404, 999.9999999999998863 ) ;
#49141=EDGE_CURVE ( 'NONE', #12593, #54974, #13771, .T. ) ;
#49144=VECTOR ( 'NONE', #51529, 999.9999999999998863 ) ;
#49148=ORIENTED_EDGE ( 'NONE', *, *, #2073, .F. ) ;
#49151=CARTESIAN_POINT ( 'NONE',  ( 61.28323125814129213, -21.66484633135379667, 40.00000000000003553 ) ) ;
#49164=VERTEX_POINT ( 'NONE', #17670 ) ;
#49165=ORIENTED_EDGE ( 'NONE', *, *, #52039, .T. ) ;
#49169=CARTESIAN_POINT ( 'NONE',  ( -4.180838820195678096, -65.23214221112786504, 43.58025477438756212 ) ) ;
#49172=DIRECTION ( 'NONE',  ( -0.9510565162951499785, -0.3090169943749582204, 0.000000000000000000 ) ) ;
#49177=VERTEX_POINT ( 'NONE', #18016 ) ;
#49179=DIRECTION ( 'NONE',  ( -0.000000000000000000, -0.000000000000000000, -1.000000000000000000 ) ) ;
#49181=CARTESIAN_POINT ( 'NONE',  ( 69.77839676787897361, -27.52340539439948586, 170.0000000000000000 ) ) ;
#49187=LINE ( 'NONE', #22476, #44809 ) ;
#49190=DIRECTION ( 'NONE',  ( 2.497525279955783991E-16, 1.121639896553914790E-17, 1.000000000000000000 ) ) ;
#49191=EDGE_CURVE ( 'NONE', #53526, #33759, #8151, .T. ) ;
#49195=CARTESIAN_POINT ( 'NONE',  ( 0.000000000000000000, 0.000000000000000000, 170.0010000000000048 ) ) ;
#49196=LINE ( 'NONE', #36080, #11669 ) ;
#49197=VERTEX_POINT ( 'NONE', #61620 ) ;
#49198=CARTESIAN_POINT ( 'NONE',  ( -15.76129977463437015, -63.43731725181460490, 43.58025477438756212 ) ) ;
#49213=VERTEX_POINT ( 'NONE', #55288 ) ;
#49215=CARTESIAN_POINT ( 'NONE',  ( 21.38432669262978436, 61.76910524360980759, 43.58025477438756212 ) ) ;
#49220=VERTEX_POINT ( 'NONE', #28926 ) ;
#49229=LINE ( 'NONE', #7739, #50948 ) ;
#49233=AXIS2_PLACEMENT_3D ( 'NONE', #36184, #3479, #68202 ) ;
#49235=EDGE_LOOP ( 'NONE', ( #65883, #27518, #20187, #34455 ) ) ;
#49237=AXIS2_PLACEMENT_3D ( 'NONE', #17048, #16369, #37828 ) ;
#49241=B_SPLINE_CURVE_WITH_KNOTS ( 'NONE', 3,
 ( #4562, #15123, #64334, #63992, #31309, #36584 ),
 .UNSPECIFIED., .F., .F.,
 ( 4, 2, 4 ),
 ( 1.095770181088979215E-06, 0.03239442681617710207, 0.06478775786217311206 ),
 .UNSPECIFIED. ) ;
#49244=ORIENTED_EDGE ( 'NONE', *, *, #42856, .T. ) ;
#49245=CARTESIAN_POINT ( 'NONE',  ( -13.32397999417976564, -63.99361958670536410, 3.125053320693569132E-16 ) ) ;
#49252=ORIENTED_EDGE ( 'NONE', *, *, #48734, .T. ) ;
#49262=EDGE_CURVE ( 'NONE', #51505, #24194, #30035, .T. ) ;
#49275=CARTESIAN_POINT ( 'NONE',  ( 31.89651141207616192, -56.63578868294582946, 40.00000000000003553 ) ) ;
#49293=ADVANCED_FACE ( 'NONE', ( #18358 ), #29600, .T. ) ;
#49296=VECTOR ( 'NONE', #33689, 1000.000000000000000 ) ;
#49300=DIRECTION ( 'NONE',  ( -1.000000000000000000, 0.000000000000000000, 0.000000000000000000 ) ) ;
#49305=EDGE_CURVE ( 'NONE', #44841, #67632, #17676, .T. ) ;
#49321=CARTESIAN_POINT ( 'NONE',  ( 45.78444578631987127, 59.41672343742573759, 170.0000000000000000 ) ) ;
#49333=CARTESIAN_POINT ( 'NONE',  ( 65.35403040894466642, -1.250000000000021982, 6.377659838150137469E-18 ) ) ;
#49335=CARTESIAN_POINT ( 'NONE',  ( 0.1230226671131348926, -25.12215469714591976, 3.061616997868437868E-16 ) ) ;
#49346=DIRECTION ( 'NONE',  ( -1.000000000000000000, 0.000000000000000000, 0.000000000000000000 ) ) ;
#49348=CARTESIAN_POINT ( 'NONE',  ( 37.34307084251124564, 44.82188538352577467, 27.58472315868181113 ) ) ;
#49350=CARTESIAN_POINT ( 'NONE',  ( 8.820885042877430138, 74.43053605947413587, 41.38025477438755928 ) ) ;
#49359=VECTOR ( 'NONE', #15017, 1000.000000000000000 ) ;
#49362=DIRECTION ( 'NONE',  ( 1.000000000000000000, 0.000000000000000000, 0.000000000000000000 ) ) ;
#49363=CARTESIAN_POINT ( 'NONE',  ( 0.000000000000000000, 0.000000000000000000, 0.000000000000000000 ) ) ;
#49375=EDGE_CURVE ( 'NONE', #26839, #6967, #9540, .T. ) ;
#49383=DIRECTION ( 'NONE',  ( 1.000000000000000000, 0.000000000000000000, -0.000000000000000000 ) ) ;
#49391=ORIENTED_EDGE ( 'NONE', *, *, #26883, .T. ) ;
#49395=EDGE_CURVE ( 'NONE', #57138, #26798, #33400, .T. ) ;
#49402=EDGE_CURVE ( 'NONE', #60863, #26321, #10213, .T. ) ;
#49427=ORIENTED_EDGE ( 'NONE', *, *, #52408, .T. ) ;
#49430=CARTESIAN_POINT ( 'NONE',  ( 4.165045035621076863, -64.88046627338039229, 170.0000000000000000 ) ) ;
#49438=ORIENTED_EDGE ( 'NONE', *, *, #34823, .T. ) ;
#49442=LINE ( 'NONE', #27298, #1999 ) ;
#49443=DIRECTION ( 'NONE',  ( 1.000000000000000000, 0.000000000000000000, 0.000000000000000000 ) ) ;
#49450=VERTEX_POINT ( 'NONE', #32721 ) ;
#49452=ORIENTED_EDGE ( 'NONE', *, *, #62333, .T. ) ;
#49457=CARTESIAN_POINT ( 'NONE',  ( -41.50537345350635121, -50.04124777106355282, 41.38025477438755928 ) ) ;
#49458=EDGE_CURVE ( 'NONE', #17792, #65052, #37289, .T. ) ;
#49460=AXIS2_PLACEMENT_3D ( 'NONE', #27652, #66366, #61061 ) ;
#49470=CARTESIAN_POINT ( 'NONE',  ( 29.67531360975017662, -24.26667169483791753, 13.32819299319724671 ) ) ;
#49472=ORIENTED_EDGE ( 'NONE', *, *, #11256, .F. ) ;
#49474=VECTOR ( 'NONE', #17376, 1000.000000000000114 ) ;
#49476=CARTESIAN_POINT ( 'NONE',  ( 34.43940527065382895, 66.63700071734666608, 170.0000000000000000 ) ) ;
#49478=CARTESIAN_POINT ( 'NONE',  ( -4.610955605663495938, 74.80943656680578613, 41.38025477438755928 ) ) ;
#49480=ORIENTED_EDGE ( 'NONE', *, *, #58825, .F. ) ;
#49483=ADVANCED_FACE ( 'NONE', ( #10561 ), #32030, .F. ) ;
#49492=DIRECTION ( 'NONE',  ( -0.04486483035050447404, -0.9989930665413151445, 0.000000000000000000 ) ) ;
#49493=ORIENTED_EDGE ( 'NONE', *, *, #44211, .T. ) ;
#49496=ORIENTED_EDGE ( 'NONE', *, *, #27485, .T. ) ;
#49502=VECTOR ( 'NONE', #27923, 1000.000000000000227 ) ;
#49507=CIRCLE ( 'NONE', #19198, 65.36598343705435354 ) ;
#49511=CARTESIAN_POINT ( 'NONE',  ( -61.29635759142585982, -21.66977272663580578, 43.58025477438756923 ) ) ;
#49537=ADVANCED_FACE ( 'NONE', ( #59780 ), #11591, .T. ) ;
#49538=CARTESIAN_POINT ( 'NONE',  ( 10.73115448446713494, 22.57968829347503714, 0.000000000000000000 ) ) ;
#49545=CARTESIAN_POINT ( 'NONE',  ( -44.00727179482512241, -47.83680621839620528, 40.00000000000003553 ) ) ;
#49547=LINE ( 'NONE', #18255, #35381 ) ;
#49548=PLANE ( 'NONE',  #4973 ) ;
#49549=ORIENTED_EDGE ( 'NONE', *, *, #35580, .F. ) ;
#49554=VERTEX_POINT ( 'NONE', #59436 ) ;
#49555=VECTOR ( 'NONE', #59257, 999.9999999999998863 ) ;
#49568=CIRCLE ( 'NONE', #55204, 65.00000000000000000 ) ;
#49573=ORIENTED_EDGE ( 'NONE', *, *, #55022, .F. ) ;
#49576=DIRECTION ( 'NONE',  ( -1.000000000000000000, 0.000000000000000000, 0.000000000000000000 ) ) ;
#49583=ORIENTED_EDGE ( 'NONE', *, *, #25723, .F. ) ;
#49602=CARTESIAN_POINT ( 'NONE',  ( 56.42997683260146857, -32.25922681454192542, 40.00000000000003553 ) ) ;
#49613=DIRECTION ( 'NONE',  ( 0.2225209339563184452, -0.9749279121818226201, 0.000000000000000000 ) ) ;
#49616=CARTESIAN_POINT ( 'NONE',  ( -84.49322488516129681, 0.000000000000000000, 43.58025477438756212 ) ) ;
#49617=AXIS2_PLACEMENT_3D ( 'NONE', #41584, #58110, #25770 ) ;
#49624=CARTESIAN_POINT ( 'NONE',  ( 70.34686579112866411, -18.11777090454118877, 170.0000000000000000 ) ) ;
#49635=CARTESIAN_POINT ( 'NONE',  ( -2.747334524841524406, 33.31268902856695746, 6.893342931471464929 ) ) ;
#49637=ORIENTED_EDGE ( 'NONE', *, *, #9282, .F. ) ;
#49653=VERTEX_POINT ( 'NONE', #39736 ) ;
#49655=CARTESIAN_POINT ( 'NONE',  ( -62.97854483871553555, -16.08424353203763602, 170.0000000000000000 ) ) ;
#49661=VECTOR ( 'NONE', #65808, 1000.000000000000114 ) ;
#49662=ADVANCED_FACE ( 'NONE', ( #1403 ), #66840, .F. ) ;
#49664=CARTESIAN_POINT ( 'NONE',  ( -65.36598343705435354, 0.000000000000000000, 41.38025477438755928 ) ) ;
#49673=AXIS2_PLACEMENT_3D ( 'NONE', #38974, #64658, #44588 ) ;
#49684=CARTESIAN_POINT ( 'NONE',  ( 0.000000000000000000, 0.000000000000000000, 0.000000000000000000 ) ) ;
#49688=EDGE_LOOP ( 'NONE', ( #60281, #43435, #22956, #56218 ) ) ;
#49698=LINE ( 'NONE', #23688, #62329 ) ;
#49701=DIRECTION ( 'NONE',  ( 1.000000000000000000, 0.000000000000000000, 0.000000000000000000 ) ) ;
#49706=VECTOR ( 'NONE', #26926, 1000.000000000000114 ) ;
#49709=DIRECTION ( 'NONE',  ( 1.000000000000000000, 0.000000000000000000, 0.000000000000000000 ) ) ;
#49711=DIRECTION ( 'NONE',  ( 1.000000000000000000, 0.000000000000000000, -0.000000000000000000 ) ) ;
#49718=CARTESIAN_POINT ( 'NONE',  ( 29.69502258243432635, -57.82046033912835270, 170.0000000000000000 ) ) ;
#49721=VECTOR ( 'NONE', #7682, 1000.000000000000000 ) ;
#49725=CARTESIAN_POINT ( 'NONE',  ( 26.12852347772543737, 70.00000000000000000, 129.5802547743875550 ) ) ;
#49726=ORIENTED_EDGE ( 'NONE', *, *, #39723, .T. ) ;
#49735=DIRECTION ( 'NONE',  ( -0.000000000000000000, -0.000000000000000000, -1.000000000000000000 ) ) ;
#49737=FACE_OUTER_BOUND ( 'NONE', #5911, .T. ) ;
#49742=EDGE_LOOP ( 'NONE', ( #3845, #37992, #7098, #33101, #50408, #21084, #33599, #27562, #14856 ) ) ;
#49753=DIRECTION ( 'NONE',  ( -0.08963930890344087854, 0.9959742939952382912, 0.000000000000000000 ) ) ;
#49756=DIRECTION ( 'NONE',  ( 6.651034621319562720E-17, 2.409948271074239284E-16, 1.000000000000000000 ) ) ;
#49758=AXIS2_PLACEMENT_3D ( 'NONE', #5670, #20475, #20138 ) ;
#49761=CONICAL_SURFACE ( 'NONE', #21648, 65.00000000000000000, 0.7853981633974497223 ) ;
#49763=CIRCLE ( 'NONE', #28436, 74.95140232871122521 ) ;
#49776=DIRECTION ( 'NONE',  ( 0.04486483035050447404, 0.9989930665413151445, 0.000000000000000000 ) ) ;
#49785=CARTESIAN_POINT ( 'NONE',  ( -49.77357484059130144, -41.82599373102875973, 41.38025477438755928 ) ) ;
#49787=CARTESIAN_POINT ( 'NONE',  ( 61.62594073580573450, -21.79346734964915555, 3.125053320693586388E-16 ) ) ;
#49796=EDGE_CURVE ( 'NONE', #62951, #23405, #5212, .T. ) ;
#49804=ORIENTED_EDGE ( 'NONE', *, *, #8894, .T. ) ;
#49806=ORIENTED_EDGE ( 'NONE', *, *, #21801, .T. ) ;
#49807=FACE_OUTER_BOUND ( 'NONE', #4103, .T. ) ;
#49812=CARTESIAN_POINT ( 'NONE',  ( -41.65447303895287234, 2.493917956440751649, 13.79046412286063550 ) ) ;
#49825=CARTESIAN_POINT ( 'NONE',  ( 45.82394788922801609, 46.11928342727494368, 3.061616997868437868E-16 ) ) ;
#49841=DIRECTION ( 'NONE',  ( -0.000000000000000000, -0.000000000000000000, 1.000000000000000000 ) ) ;
#49850=FACE_OUTER_BOUND ( 'NONE', #65459, .T. ) ;
#49854=ORIENTED_EDGE ( 'NONE', *, *, #15653, .F. ) ;
#49856=CIRCLE ( 'NONE', #48679, 65.36598343705435354 ) ;
#49860=DIRECTION ( 'NONE',  ( 0.9839295885986296675, 0.1785568947986370669, 0.000000000000000000 ) ) ;
#49876=EDGE_LOOP ( 'NONE', ( #44124, #18956, #20476, #1758 ) ) ;
#49882=EDGE_CURVE ( 'NONE', #45637, #35650, #4863, .T. ) ;
#49886=CARTESIAN_POINT ( 'NONE',  ( 0.000000000000000000, 0.000000000000000000, 40.00000000000003553 ) ) ;
#49888=DIRECTION ( 'NONE',  ( 0.7530714660036099684, 0.6579387259397136978, 0.000000000000000000 ) ) ;
#49891=ORIENTED_EDGE ( 'NONE', *, *, #40894, .T. ) ;
#49896=LINE ( 'NONE', #43570, #60152 ) ;
#49902=ORIENTED_EDGE ( 'NONE', *, *, #42152, .F. ) ;
#49904=PLANE ( 'NONE',  #53180 ) ;
#49915=ORIENTED_EDGE ( 'NONE', *, *, #33675, .F. ) ;
#49922=DIRECTION ( 'NONE',  ( -0.2225209339563184452, 0.9749279121818226201, 0.000000000000000000 ) ) ;
#49936=CARTESIAN_POINT ( 'NONE',  ( 0.000000000000000000, 0.000000000000000000, 0.000000000000000000 ) ) ;
#49942=DIRECTION ( 'NONE',  ( -0.000000000000000000, -0.000000000000000000, 1.000000000000000000 ) ) ;
#49948=DIRECTION ( 'NONE',  ( 0.9195277725514544587, -0.3930250316539148359, 2.500042656554809847E-16 ) ) ;
#49951=VERTEX_POINT ( 'NONE', #28761 ) ;
#49972=CARTESIAN_POINT ( 'NONE',  ( 29.67531435111662219, 24.26667234255101135, 13.32819397642333215 ) ) ;
#49978=VECTOR ( 'NONE', #27358, 1000.000000000000114 ) ;
#49979=CARTESIAN_POINT ( 'NONE',  ( 66.63364047053092065, -1.250000000000021760, 34.48241795236666007 ) ) ;
#49988=LINE ( 'NONE', #29927, #13643 ) ;
#49991=CARTESIAN_POINT ( 'NONE',  ( -52.13778968636738398, -39.42540649522064911, 41.38025477438755928 ) ) ;
#50012=EDGE_CURVE ( 'NONE', #59078, #6708, #57048, .T. ) ;
#50016=DIRECTION ( 'NONE',  ( -0.000000000000000000, -0.000000000000000000, -1.000000000000000000 ) ) ;
#50017=LINE ( 'NONE', #49655, #26036 ) ;
#50019=B_SPLINE_CURVE_WITH_KNOTS ( 'NONE', 3,
 ( #24422, #45864, #39547, #61001 ),
 .UNSPECIFIED., .F., .F.,
 ( 4, 4 ),
 ( 9.900409499071532726E-07, 0.05658314289920116785 ),
 .UNSPECIFIED. ) ;
#50029=CIRCLE ( 'NONE', #11866, 65.36598343705435354 ) ;
#50031=ORIENTED_EDGE ( 'NONE', *, *, #816, .T. ) ;
#50039=ORIENTED_EDGE ( 'NONE', *, *, #48812, .F. ) ;
#50040=EDGE_CURVE ( 'NONE', #43949, #56091, #40344, .T. ) ;
#50041=EDGE_CURVE ( 'NONE', #7321, #57335, #31630, .T. ) ;
#50042=ORIENTED_EDGE ( 'NONE', *, *, #55330, .T. ) ;
#50047=DIRECTION ( 'NONE',  ( 0.000000000000000000, 0.000000000000000000, 1.000000000000000000 ) ) ;
#50070=CONICAL_SURFACE ( 'NONE', #46698, 65.00000000000000000, 0.7853981633974497223 ) ;
#50072=ORIENTED_EDGE ( 'NONE', *, *, #12817, .F. ) ;
#50073=VERTEX_POINT ( 'NONE', #13612 ) ;
#50087=ORIENTED_EDGE ( 'NONE', *, *, #24481, .T. ) ;
#50106=B_SPLINE_CURVE_WITH_KNOTS ( 'NONE', 3,
 ( #11165, #974, #32976, #22768 ),
 .UNSPECIFIED., .F., .F.,
 ( 4, 4 ),
 ( 0.1259919275528360583, 0.1829744153748752988 ),
 .UNSPECIFIED. ) ;
#50113=CARTESIAN_POINT ( 'NONE',  ( 36.85262215550070408, 53.56030941157735015, 41.38025477438755928 ) ) ;
#50114=CARTESIAN_POINT ( 'NONE',  ( 21.38432669262978436, 61.76910524360980759, 6.377659838150160580E-18 ) ) ;
#50116=ORIENTED_EDGE ( 'NONE', *, *, #797, .T. ) ;
#50131=DIRECTION ( 'NONE',  ( 5.055952397801357946E-18, -6.848752866791659805E-19, -1.000000000000000000 ) ) ;
#50141=CARTESIAN_POINT ( 'NONE',  ( 0.000000000000000000, 0.000000000000000000, 170.0000000000000000 ) ) ;
#50143=ORIENTED_EDGE ( 'NONE', *, *, #2324, .F. ) ;
#50151=DIRECTION ( 'NONE',  ( -0.7530714660036099684, -0.6579387259397138088, 0.000000000000000000 ) ) ;
#50159=CARTESIAN_POINT ( 'NONE',  ( -11.97857133224687409, 31.20571980842448667, 6.893343212288939093 ) ) ;
#50172=LINE ( 'NONE', #50863, #38575 ) ;
#50176=CARTESIAN_POINT ( 'NONE',  ( -15.47041015649551809, -73.39774458108233546, 43.58025477438756923 ) ) ;
#50178=CIRCLE ( 'NONE', #59145, 65.00000000000000000 ) ;
#50191=ORIENTED_EDGE ( 'NONE', *, *, #32132, .T. ) ;
#50193=EDGE_CURVE ( 'NONE', #54158, #53910, #48351, .T. ) ;
#50201=CARTESIAN_POINT ( 'NONE',  ( -58.20343000000241318, -3.983351041215688504, 27.58472315868180402 ) ) ;
#50204=DIRECTION ( 'NONE',  ( -0.000000000000000000, -0.000000000000000000, 1.000000000000000000 ) ) ;
#50212=EDGE_CURVE ( 'NONE', #48110, #33531, #45794, .T. ) ;
#50223=VECTOR ( 'NONE', #19291, 999.9999999999998863 ) ;
#50225=ORIENTED_EDGE ( 'NONE', *, *, #56532, .T. ) ;
#50231=VECTOR ( 'NONE', #12811, 1000.000000000000000 ) ;
#50236=DIRECTION ( 'NONE',  ( -0.000000000000000000, -0.000000000000000000, -1.000000000000000000 ) ) ;
#50242=CARTESIAN_POINT ( 'NONE',  ( 21.27121078971612889, 61.42097029141972087, 133.5802547743875550 ) ) ;
#50252=EDGE_CURVE ( 'NONE', #7475, #42734, #33612, .T. ) ;
#50264=AXIS2_PLACEMENT_3D ( 'NONE', #60918, #50016, #2192 ) ;
#50266=DIRECTION ( 'NONE',  ( -0.5877852522924802425, 0.8090169943749422332, 0.000000000000000000 ) ) ;
#50268=CARTESIAN_POINT ( 'NONE',  ( -64.18058723658640474, -10.37664328995270857, 43.58025477438756923 ) ) ;
#50276=EDGE_CURVE ( 'NONE', #14895, #15856, #22345, .T. ) ;
#50280=EDGE_CURVE ( 'NONE', #20254, #32779, #39574, .T. ) ;
#50284=AXIS2_PLACEMENT_3D ( 'NONE', #29981, #66594, #34589 ) ;
#50286=CARTESIAN_POINT ( 'NONE',  ( -17.90772993695113868, 72.84144224619130625, 170.0000000000000000 ) ) ;
#50291=CARTESIAN_POINT ( 'NONE',  ( -29.87147652227456263, 100.0000000000000000, 73.58025477438756923 ) ) ;
#50296=DIRECTION ( 'NONE',  ( -0.000000000000000000, -0.000000000000000000, -1.000000000000000000 ) ) ;
#50297=CARTESIAN_POINT ( 'NONE',  ( 61.91366885787727625, 28.42865614899003290, 170.0000000000000000 ) ) ;
#50302=ORIENTED_EDGE ( 'NONE', *, *, #60618, .T. ) ;
#50318=B_SPLINE_CURVE_WITH_KNOTS ( 'NONE', 3,
 ( #9100, #30548, #30898, #10123 ),
 .UNSPECIFIED., .F., .F.,
 ( 4, 4 ),
 ( 0.1259919275528358362, 0.1829744153748746882 ),
 .UNSPECIFIED. ) ;
#50331=CARTESIAN_POINT ( 'NONE',  ( -0.2498518736781690786, 33.42485144267424602, 6.893343212288930211 ) ) ;
#50344=CARTESIAN_POINT ( 'NONE',  ( 0.000000000000000000, 0.000000000000000000, 0.000000000000000000 ) ) ;
#50349=DIRECTION ( 'NONE',  ( -1.000000000000000000, 0.000000000000000000, 0.000000000000000000 ) ) ;
#50354=ORIENTED_EDGE ( 'NONE', *, *, #62889, .F. ) ;
#50355=ORIENTED_EDGE ( 'NONE', *, *, #62408, .F. ) ;
#50359=LINE ( 'NONE', #60204, #1976 ) ;
#50364=EDGE_CURVE ( 'NONE', #35065, #38023, #40265, .T. ) ;
#50366=ORIENTED_EDGE ( 'NONE', *, *, #20334, .F. ) ;
#50377=CARTESIAN_POINT ( 'NONE',  ( 1.667562369267789890, -64.99262834925670518, 170.0000000000000000 ) ) ;
#50381=DIRECTION ( 'NONE',  ( -1.000000000000000000, 0.000000000000000000, 0.000000000000000000 ) ) ;
#50389=DIRECTION ( 'NONE',  ( -0.000000000000000000, 0.000000000000000000, -1.000000000000000000 ) ) ;
#50408=ORIENTED_EDGE ( 'NONE', *, *, #30355, .F. ) ;
#50410=VERTEX_POINT ( 'NONE', #25138 ) ;
#50412=CARTESIAN_POINT ( 'NONE',  ( -4.364688291132434728, -24.74039788130350459, 3.061616997868437868E-16 ) ) ;
#50439=CARTESIAN_POINT ( 'NONE',  ( -18.15845058245960075, 17.18344181019522310, 0.000000000000000000 ) ) ;
#50446=ORIENTED_EDGE ( 'NONE', *, *, #2551, .T. ) ;
#50456=CYLINDRICAL_SURFACE ( 'NONE', #57959, 65.00000000000000000 ) ;
#50458=ORIENTED_EDGE ( 'NONE', *, *, #24142, .T. ) ;
#50463=DIRECTION ( 'NONE',  ( 0.9839295885986321100, -0.1785568947986229116, 0.000000000000000000 ) ) ;
#50465=VERTEX_POINT ( 'NONE', #2988 ) ;
#50473=ORIENTED_EDGE ( 'NONE', *, *, #60280, .F. ) ;
#50478=CARTESIAN_POINT ( 'NONE',  ( 36.61292551086699376, -65.40035471292219427, 41.38025477438755928 ) ) ;
#50479=AXIS2_PLACEMENT_3D ( 'NONE', #14218, #41979, #58485 ) ;
#50480=CARTESIAN_POINT ( 'NONE',  ( 38.61145386526410306, 15.82625607536648005, 13.79046412312118086 ) ) ;
#50482=ORIENTED_EDGE ( 'NONE', *, *, #31675, .F. ) ;
#50489=CARTESIAN_POINT ( 'NONE',  ( -27.41072479265578110, -43.79449985997803196, 26.66469066592268433 ) ) ;
#50495=DIRECTION ( 'NONE',  ( -1.000000000000000000, 0.000000000000000000, 0.000000000000000000 ) ) ;
#50508=DIRECTION ( 'NONE',  ( -0.000000000000000000, -0.000000000000000000, -1.000000000000000000 ) ) ;
#50514=FACE_OUTER_BOUND ( 'NONE', #56972, .T. ) ;
#50518=DIRECTION ( 'NONE',  ( 1.000000000000000000, 0.000000000000000000, -0.000000000000000000 ) ) ;
#50523=CARTESIAN_POINT ( 'NONE',  ( -58.20343064176747561, 3.983351098974750482, 27.58472369368492139 ) ) ;
#50524=CIRCLE ( 'NONE', #28015, 65.00000000000000000 ) ;
#50525=CARTESIAN_POINT ( 'NONE',  ( 47.73902449249074920, -57.85799893277823713, 170.0000000000000000 ) ) ;
#50527=CIRCLE ( 'NONE', #46051, 74.95140232871122521 ) ;
#50530=CARTESIAN_POINT ( 'NONE',  ( 0.000000000000000000, 0.000000000000000000, 0.000000000000000000 ) ) ;
#50539=ORIENTED_EDGE ( 'NONE', *, *, #56060, .F. ) ;
#50542=CARTESIAN_POINT ( 'NONE',  ( 56.56044417847081718, -35.24940704026185045, 34.48241795236666718 ) ) ;
#50544=CARTESIAN_POINT ( 'NONE',  ( -49.77357484059130144, -41.82599373102875973, 43.58025477438756923 ) ) ;
#50553=ORIENTED_EDGE ( 'NONE', *, *, #35814, .F. ) ;
#50569=CARTESIAN_POINT ( 'NONE',  ( 45.78444578631984285, 59.41672343742577311, 43.58025477438756923 ) ) ;
#50571=AXIS2_PLACEMENT_3D ( 'NONE', #67615, #19415, #40872 ) ;
#50573=ORIENTED_EDGE ( 'NONE', *, *, #288, .T. ) ;
#50589=DIRECTION ( 'NONE',  ( -0.7818314824680221431, -0.6234898018587432533, 5.102127870520021999E-18 ) ) ;
#50592=ORIENTED_EDGE ( 'NONE', *, *, #65796, .T. ) ;
#50611=DIRECTION ( 'NONE',  ( 0.7818314824680311359, -0.6234898018587318180, 5.102127870520020458E-18 ) ) ;
#50612=DIRECTION ( 'NONE',  ( 1.000000000000000000, 0.000000000000000000, -0.000000000000000000 ) ) ;
#50613=VERTEX_POINT ( 'NONE', #7318 ) ;
#50628=ORIENTED_EDGE ( 'NONE', *, *, #61473, .T. ) ;
#50630=DIRECTION ( 'NONE',  ( -0.000000000000000000, -0.000000000000000000, -1.000000000000000000 ) ) ;
#50633=CARTESIAN_POINT ( 'NONE',  ( 5.722400986011420443, -32.93231276838069022, 6.893342931642330029 ) ) ;
#50635=AXIS2_PLACEMENT_3D ( 'NONE', #4180, #45705, #25648 ) ;
#50650=FACE_OUTER_BOUND ( 'NONE', #58493, .T. ) ;
#50691=LINE ( 'NONE', #24666, #8370 ) ;
#50696=LINE ( 'NONE', #30634, #25485 ) ;
#50711=ORIENTED_EDGE ( 'NONE', *, *, #26426, .T. ) ;
#50712=PLANE ( 'NONE',  #53711 ) ;
#50713=DIRECTION ( 'NONE',  ( -0.000000000000000000, -0.000000000000000000, -1.000000000000000000 ) ) ;
#50715=CARTESIAN_POINT ( 'NONE',  ( -72.62976060914746768, 18.74780984163032826, 43.58025477438756923 ) ) ;
#50722=CARTESIAN_POINT ( 'NONE',  ( -64.56490107723145400, 16.52205003563488006, 34.48241823982461085 ) ) ;
#50723=ORIENTED_EDGE ( 'NONE', *, *, #40967, .F. ) ;
#50727=CARTESIAN_POINT ( 'NONE',  ( 63.00000000000000000, 7.715274834628325378E-15, 170.0000000000000000 ) ) ;
#50730=ORIENTED_EDGE ( 'NONE', *, *, #36033, .F. ) ;
#50739=CIRCLE ( 'NONE', #21553, 65.00000000000000000 ) ;
#50740=CARTESIAN_POINT ( 'NONE',  ( -23.73638277007043840, 7.847555861075215411, 0.000000000000000000 ) ) ;
#50745=LINE ( 'NONE', #1884, #33168 ) ;
#50760=ORIENTED_EDGE ( 'NONE', *, *, #6174, .F. ) ;
#50772=FACE_OUTER_BOUND ( 'NONE', #6551, .T. ) ;
#50775=DIRECTION ( 'NONE',  ( -0.000000000000000000, -0.000000000000000000, -1.000000000000000000 ) ) ;
#50776=CARTESIAN_POINT ( 'NONE',  ( -74.52723870109939242, -7.962625360375267469, 41.38025477438755928 ) ) ;
#50787=CONICAL_SURFACE ( 'NONE', #10352, 65.00000000000000000, 0.7853981633974497223 ) ;
#50793=FACE_OUTER_BOUND ( 'NONE', #33416, .T. ) ;
#50802=DIRECTION ( 'NONE',  ( -0.04486483035051862939, 0.9989930665413143673, 0.000000000000000000 ) ) ;
#50803=LINE ( 'NONE', #50113, #33461 ) ;
#50805=ORIENTED_EDGE ( 'NONE', *, *, #47545, .F. ) ;
#50809=ORIENTED_EDGE ( 'NONE', *, *, #11877, .T. ) ;
#50829=ADVANCED_FACE ( 'NONE', ( #43451 ), #65269, .T. ) ;
#50834=VERTEX_POINT ( 'NONE', #45902 ) ;
#50840=CARTESIAN_POINT ( 'NONE',  ( 39.54205320694339321, 51.58901073076764021, 170.0000000000000000 ) ) ;
#50844=LINE ( 'NONE', #61398, #28642 ) ;
#50848=VERTEX_POINT ( 'NONE', #34318 ) ;
#50860=ORIENTED_EDGE ( 'NONE', *, *, #26231, .T. ) ;
#50863=CARTESIAN_POINT ( 'NONE',  ( -56.44201257846631847, 32.26641783793562013, 0.000000000000000000 ) ) ;
#50871=EDGE_LOOP ( 'NONE', ( #6586, #57650, #66906, #6987 ) ) ;
#50873=FACE_OUTER_BOUND ( 'NONE', #66507, .T. ) ;
#50875=LINE ( 'NONE', #39978, #55549 ) ;
#50880=VECTOR ( 'NONE', #34174, 1000.000000000000114 ) ;
#50889=PLANE ( 'NONE',  #39132 ) ;
#50896=EDGE_CURVE ( 'NONE', #2615, #26373, #40969, .T. ) ;
#50902=B_SPLINE_CURVE_WITH_KNOTS ( 'NONE', 3,
 ( #69109, #31166, #10369, #20244, #4416, #58223 ),
 .UNSPECIFIED., .F., .F.,
 ( 4, 2, 4 ),
 ( 1.095770181115537934E-06, 0.03239442681617711595, 0.06478775786217312593 ),
 .UNSPECIFIED. ) ;
#50905=VECTOR ( 'NONE', #4051, 1000.000000000000000 ) ;
#50906=PLANE ( 'NONE',  #32537 ) ;
#50911=ORIENTED_EDGE ( 'NONE', *, *, #53734, .F. ) ;
#50912=ORIENTED_EDGE ( 'NONE', *, *, #39579, .T. ) ;
#50916=ADVANCED_FACE ( 'NONE', ( #26171 ), #37402, .F. ) ;
#50933=VECTOR ( 'NONE', #10871, 1000.000000000000000 ) ;
#50935=CARTESIAN_POINT ( 'NONE',  ( -7.486743542470078339, 64.58150799671128084, 170.0000000000000000 ) ) ;
#50943=ORIENTED_EDGE ( 'NONE', *, *, #31366, .T. ) ;
#50944=VECTOR ( 'NONE', #7979, 1000.000000000000114 ) ;
#50948=VECTOR ( 'NONE', #45006, 1000.000000000000227 ) ;
#50956=VECTOR ( 'NONE', #32173, 1000.000000000000114 ) ;
#50957=DIRECTION ( 'NONE',  ( -0.9009688679024155933, -0.4338837391175656699, 0.000000000000000000 ) ) ;
#50979=CARTESIAN_POINT ( 'NONE',  ( 63.72039997003709288, 12.83396383267841223, 170.0000000000000000 ) ) ;
#50992=DIRECTION ( 'NONE',  ( 0.9909497617679351444, -0.1342332658176522420, 0.000000000000000000 ) ) ;
#50994=ORIENTED_EDGE ( 'NONE', *, *, #43887, .F. ) ;
#50995=AXIS2_PLACEMENT_3D ( 'NONE', #66799, #61504, #35108 ) ;
#51002=CIRCLE ( 'NONE', #45422, 65.00000000000000000 ) ;
#51011=DIRECTION ( 'NONE',  ( -0.000000000000000000, 0.000000000000000000, -1.000000000000000000 ) ) ;
#51013=LINE ( 'NONE', #51702, #52277 ) ;
#51025=DIRECTION ( 'NONE',  ( -0.000000000000000000, -0.000000000000000000, -1.000000000000000000 ) ) ;
#51026=CARTESIAN_POINT ( 'NONE',  ( -74.69807204964297398, 6.722948167756991111, 0.000000000000000000 ) ) ;
#51033=CARTESIAN_POINT ( 'NONE',  ( -65.00200000000002376, -1.250000000000021982, 0.000000000000000000 ) ) ;
#51034=VERTEX_POINT ( 'NONE', #49335 ) ;
#51037=VECTOR ( 'NONE', #3983, 1000.000000000000227 ) ;
#51039=LINE ( 'NONE', #33818, #37868 ) ;
#51043=EDGE_CURVE ( 'NONE', #65910, #4577, #21572, .T. ) ;
#51046=ORIENTED_EDGE ( 'NONE', *, *, #54703, .F. ) ;
#51057=ORIENTED_EDGE ( 'NONE', *, *, #24333, .T. ) ;
#51058=DIRECTION ( 'NONE',  ( -0.000000000000000000, -0.000000000000000000, -1.000000000000000000 ) ) ;
#51061=CARTESIAN_POINT ( 'NONE',  ( 25.12245591505646658, 0.000000000000000000, 0.000000000000000000 ) ) ;
#51066=ORIENTED_EDGE ( 'NONE', *, *, #6251, .F. ) ;
#51079=CARTESIAN_POINT ( 'NONE',  ( 8.828807734115068584, -74.48902371486708773, 170.0000000000000000 ) ) ;
#51084=DIRECTION ( 'NONE',  ( -0.000000000000000000, -0.000000000000000000, -1.000000000000000000 ) ) ;
#51092=FACE_OUTER_BOUND ( 'NONE', #54021, .T. ) ;
#51099=DIRECTION ( 'NONE',  ( 0.1785568947986370392, -0.9839295885986295565, 0.000000000000000000 ) ) ;
#51100=DIRECTION ( 'NONE',  ( -0.000000000000000000, -0.000000000000000000, -1.000000000000000000 ) ) ;
#51111=DIRECTION ( 'NONE',  ( 1.000000000000000000, 0.000000000000000000, 0.000000000000000000 ) ) ;
#51129=ORIENTED_EDGE ( 'NONE', *, *, #40363, .T. ) ;
#51134=FACE_OUTER_BOUND ( 'NONE', #8046, .T. ) ;
#51148=LINE ( 'NONE', #40246, #39701 ) ;
#51152=VECTOR ( 'NONE', #44774, 1000.000000000000114 ) ;
#51163=ORIENTED_EDGE ( 'NONE', *, *, #34499, .T. ) ;
#51165=DIRECTION ( 'NONE',  ( -1.000000000000000000, 0.000000000000000000, 0.000000000000000000 ) ) ;
#51175=CARTESIAN_POINT ( 'NONE',  ( -40.27405704175546930, -63.28161525591320924, 170.0000000000000000 ) ) ;
#51177=DIRECTION ( 'NONE',  ( -0.9959742939952382912, -0.08963930890344089242, 0.000000000000000000 ) ) ;
#51184=VECTOR ( 'NONE', #23767, 1000.000000000000000 ) ;
#51191=CIRCLE ( 'NONE', #47802, 74.95140232871122521 ) ;
#51193=ORIENTED_EDGE ( 'NONE', *, *, #64468, .T. ) ;
#51197=CARTESIAN_POINT ( 'NONE',  ( 0.000000000000000000, 0.000000000000000000, 0.000000000000000000 ) ) ;
#51201=CIRCLE ( 'NONE', #20859, 65.00000000000000000 ) ;
#51205=ORIENTED_EDGE ( 'NONE', *, *, #30523, .T. ) ;
#51207=PLANE ( 'NONE',  #14744 ) ;
#51215=ORIENTED_EDGE ( 'NONE', *, *, #63938, .F. ) ;
#51216=DIRECTION ( 'NONE',  ( -0.000000000000000000, -0.000000000000000000, -1.000000000000000000 ) ) ;
#51217=EDGE_CURVE ( 'NONE', #34928, #69323, #29356, .T. ) ;
#51221=CARTESIAN_POINT ( 'NONE',  ( -74.75133697335806460, 5.472689625386069068, 41.38025477438755928 ) ) ;
#51232=DIRECTION ( 'NONE',  ( -0.2225209339563184729, 0.9749279121818227312, 0.000000000000000000 ) ) ;
#51238=EDGE_CURVE ( 'NONE', #60669, #17123, #41917, .T. ) ;
#51259=ORIENTED_EDGE ( 'NONE', *, *, #65354, .T. ) ;
#51260=DIRECTION ( 'NONE',  ( -0.8345732537213078617, 0.5508969814520945363, 0.000000000000000000 ) ) ;
#51264=CARTESIAN_POINT ( 'NONE',  ( -20.06363881723563480, 32.66414036569511836, 13.32819397642332682 ) ) ;
#51266=ORIENTED_EDGE ( 'NONE', *, *, #6338, .T. ) ;
#51277=ORIENTED_EDGE ( 'NONE', *, *, #27448, .T. ) ;
#51287=VECTOR ( 'NONE', #19547, 999.9999999999998863 ) ;
#51293=DIRECTION ( 'NONE',  ( -0.8584487936018655452, -0.5128992774059070170, 0.000000000000000000 ) ) ;
#51297=CARTESIAN_POINT ( 'NONE',  ( 49.35746990687617597, -44.78219184840987310, 34.48241795236666718 ) ) ;
#51302=ORIENTED_EDGE ( 'NONE', *, *, #15901, .F. ) ;
#51315=ORIENTED_EDGE ( 'NONE', *, *, #4290, .T. ) ;
#51322=CARTESIAN_POINT ( 'NONE',  ( -25.87147652227456263, 70.00000000000000000, 77.58025477438755502 ) ) ;
#51325=DIRECTION ( 'NONE',  ( -0.000000000000000000, -0.000000000000000000, -1.000000000000000000 ) ) ;
#51326=EDGE_CURVE ( 'NONE', #28608, #40972, #20357, .T. ) ;
#51329=CARTESIAN_POINT ( 'NONE',  ( -64.56490074351019359, -16.52204994353465395, 34.48241795236665297 ) ) ;
#51332=ORIENTED_EDGE ( 'NONE', *, *, #63163, .F. ) ;
#51339=ORIENTED_EDGE ( 'NONE', *, *, #35244, .T. ) ;
#51341=DIRECTION ( 'NONE',  ( 0.000000000000000000, 0.000000000000000000, 1.000000000000000000 ) ) ;
#51351=VECTOR ( 'NONE', #45648, 1000.000000000000000 ) ;
#51352=CARTESIAN_POINT ( 'NONE',  ( 48.39383208188382213, 43.94028683479088926, 41.38025477438755928 ) ) ;
#51359=ORIENTED_EDGE ( 'NONE', *, *, #38041, .T. ) ;
#51361=DIRECTION ( 'NONE',  ( -0.5508969814520944253, -0.8345732537213078617, 0.000000000000000000 ) ) ;
#51372=EDGE_CURVE ( 'NONE', #66025, #5466, #22616, .T. ) ;
#51373=CARTESIAN_POINT ( 'NONE',  ( -0.6225858422299265227, 41.72441810409881668, 13.79046340968177731 ) ) ;
#51379=DIRECTION ( 'NONE',  ( -0.9959742939952382912, -0.08963930890344087854, 0.000000000000000000 ) ) ;
#51382=DIRECTION ( 'NONE',  ( -0.9959742939952397345, 0.08963930890342655666, 0.000000000000000000 ) ) ;
#51389=LINE ( 'NONE', #45760, #41091 ) ;
#51392=DIRECTION ( 'NONE',  ( 0.9839295885986321100, -0.1785568947986229116, 0.000000000000000000 ) ) ;
#51398=LINE ( 'NONE', #24323, #10596 ) ;
#51402=ORIENTED_EDGE ( 'NONE', *, *, #31301, .F. ) ;
#51404=CARTESIAN_POINT ( 'NONE',  ( -12.77952633087662093, -21.62918162951127243, 3.061616997868437868E-16 ) ) ;
#51408=ADVANCED_FACE ( 'NONE', ( #43977 ), #64401, .F. ) ;
#51421=CARTESIAN_POINT ( 'NONE',  ( 64.98797965777978902, -1.250000000000021760, 40.00000000000003553 ) ) ;
#51427=ORIENTED_EDGE ( 'NONE', *, *, #14986, .F. ) ;
#51431=AXIS2_PLACEMENT_3D ( 'NONE', #35658, #36001, #68686 ) ;
#51432=CARTESIAN_POINT ( 'NONE',  ( 60.40479419793796012, -24.00543350795315334, 40.00000000000003553 ) ) ;
#51433=ORIENTED_EDGE ( 'NONE', *, *, #63021, .F. ) ;
#51435=DIRECTION ( 'NONE',  ( -1.000000000000000000, 0.000000000000000000, 0.000000000000000000 ) ) ;
#51438=ORIENTED_EDGE ( 'NONE', *, *, #51217, .T. ) ;
#51443=ORIENTED_EDGE ( 'NONE', *, *, #45101, .T. ) ;
#51446=VECTOR ( 'NONE', #29995, 1000.000000000000000 ) ;
#51448=DIRECTION ( 'NONE',  ( -1.000000000000000000, 0.000000000000000000, 0.000000000000000000 ) ) ;
#51451=LINE ( 'NONE', #61304, #28755 ) ;
#51459=DIRECTION ( 'NONE',  ( -0.000000000000000000, 0.000000000000000000, -1.000000000000000000 ) ) ;
#51461=EDGE_CURVE ( 'NONE', #35105, #56882, #27813, .T. ) ;
#51467=CARTESIAN_POINT ( 'NONE',  ( 63.74253542338254164, 39.54050679744537433, 43.58025477438756923 ) ) ;
#51470=VERTEX_POINT ( 'NONE', #38019 ) ;
#51481=B_SPLINE_CURVE_WITH_KNOTS ( 'NONE', 3,
 ( #39953, #6555, #34692, #22378, #50159, #66364 ),
 .UNSPECIFIED., .F., .F.,
 ( 4, 2, 4 ),
 ( 1.095770181102079639E-06, 0.03239442681617710207, 0.06478775786217311206 ),
 .UNSPECIFIED. ) ;
#51482=ORIENTED_EDGE ( 'NONE', *, *, #55129, .T. ) ;
#51488=VECTOR ( 'NONE', #8781, 1000.000000000000000 ) ;
#51495=CARTESIAN_POINT ( 'NONE',  ( 70.65683382808195745, 25.18281821780106711, 170.0000000000000000 ) ) ;
#51496=CARTESIAN_POINT ( 'NONE',  ( 57.61205526789942866, 9.184630482019173314, 27.58472315868180402 ) ) ;
#51503=VECTOR ( 'NONE', #37692, 1000.000000000000000 ) ;
#51505=VERTEX_POINT ( 'NONE', #61571 ) ;
#51507=DIRECTION ( 'NONE',  ( -0.6910626489868580968, -0.7227948638273978821, 0.000000000000000000 ) ) ;
#51512=ORIENTED_EDGE ( 'NONE', *, *, #10735, .T. ) ;
#51516=CYLINDRICAL_SURFACE ( 'NONE', #67875, 65.36598343705435354 ) ;
#51529=DIRECTION ( 'NONE',  ( 0.1342332658176522420, 0.9909497617679352555, -3.104767966278886959E-17 ) ) ;
#51531=CARTESIAN_POINT ( 'NONE',  ( 0.000000000000000000, 0.000000000000000000, 40.00000000000003553 ) ) ;
#51533=CARTESIAN_POINT ( 'NONE',  ( 64.16679220703382214, -10.37413986118096432, 170.0000000000000000 ) ) ;
#51537=ORIENTED_EDGE ( 'NONE', *, *, #58850, .F. ) ;
#51539=ORIENTED_EDGE ( 'NONE', *, *, #65166, .T. ) ;
#51554=CARTESIAN_POINT ( 'NONE',  ( -84.49322488516129681, 0.000000000000000000, 43.58025477438756212 ) ) ;
#51565=DIRECTION ( 'NONE',  ( 0.9639628606958512425, 0.2660368455666826670, 0.000000000000000000 ) ) ;
#51577=DIRECTION ( 'NONE',  ( 2.312964634635743450E-16, -0.000000000000000000, 1.000000000000000000 ) ) ;
#51583=VECTOR ( 'NONE', #56270, 1000.000000000000000 ) ;
#51586=PLANE ( 'NONE',  #65509 ) ;
#51588=CARTESIAN_POINT ( 'NONE',  ( 13.24564585880132839, -63.65041531508827433, 41.38025477438755928 ) ) ;
#51592=ORIENTED_EDGE ( 'NONE', *, *, #58715, .F. ) ;
#51599=CARTESIAN_POINT ( 'NONE',  ( 22.07550062443499428, -11.73338281062043364, 0.000000000000000000 ) ) ;
#51601=CARTESIAN_POINT ( 'NONE',  ( -23.98664742203151690, 23.27925779329526179, 6.893342939543522618 ) ) ;
#51602=CARTESIAN_POINT ( 'NONE',  ( -62.66631205405185057, 18.59153367093362874, 41.38025477438755928 ) ) ;
#51622=CARTESIAN_POINT ( 'NONE',  ( 0.000000000000000000, 0.000000000000000000, 0.000000000000000000 ) ) ;
#51628=EDGE_CURVE ( 'NONE', #43978, #13483, #49568, .T. ) ;
#51629=ORIENTED_EDGE ( 'NONE', *, *, #35967, .T. ) ;
#51636=LINE ( 'NONE', #9416, #55092 ) ;
#51638=CARTESIAN_POINT ( 'NONE',  ( 0.000000000000000000, 0.000000000000000000, 170.0000000000000000 ) ) ;
#51640=ORIENTED_EDGE ( 'NONE', *, *, #34778, .T. ) ;
#51655=CARTESIAN_POINT ( 'NONE',  ( -68.11501976657811497, -31.41506934893937952, 170.0000000000000000 ) ) ;
#51666=ORIENTED_EDGE ( 'NONE', *, *, #26205, .T. ) ;
#51674=DIRECTION ( 'NONE',  ( -0.000000000000000000, 0.000000000000000000, -1.000000000000000000 ) ) ;
#51676=FILL_AREA_STYLE_COLOUR ( '', #27024 ) ;
#51678=ORIENTED_EDGE ( 'NONE', *, *, #51238, .F. ) ;
#51683=FACE_OUTER_BOUND ( 'NONE', #3798, .T. ) ;
#51684=AXIS2_PLACEMENT_3D ( 'NONE', #30314, #67954, #14480 ) ;
#51692=CARTESIAN_POINT ( 'NONE',  ( 0.000000000000000000, 0.000000000000000000, 41.38025477438755928 ) ) ;
#51693=EDGE_LOOP ( 'NONE', ( #35843, #30273, #44232, #43532 ) ) ;
#51702=CARTESIAN_POINT ( 'NONE',  ( 74.62299871641495486, 5.461138973199027191, 43.58025477438756923 ) ) ;
#51716=DIRECTION ( 'NONE',  ( 1.000000000000000000, 0.000000000000000000, -0.000000000000000000 ) ) ;
#51723=DIRECTION ( 'NONE',  ( -0.1785568947986229393, -0.9839295885986322210, 0.000000000000000000 ) ) ;
#51725=DIRECTION ( 'NONE',  ( -0.000000000000000000, -0.000000000000000000, -1.000000000000000000 ) ) ;
#51746=CARTESIAN_POINT ( 'NONE',  ( 0.000000000000000000, 0.000000000000000000, 170.0000000000000000 ) ) ;
#51754=ORIENTED_EDGE ( 'NONE', *, *, #16181, .F. ) ;
#51756=LINE ( 'NONE', #25035, #29395 ) ;
#51767=ADVANCED_FACE ( 'NONE', ( #66694 ), #13560, .T. ) ;
#51772=CARTESIAN_POINT ( 'NONE',  ( 0.000000000000000000, 0.000000000000000000, 0.000000000000000000 ) ) ;
#51788=ORIENTED_EDGE ( 'NONE', *, *, #19128, .F. ) ;
#51789=AXIS2_PLACEMENT_3D ( 'NONE', #42876, #37963, #16156 ) ;
#51792=AXIS2_PLACEMENT_3D ( 'NONE', #887, #22339, #55742 ) ;
#51797=CARTESIAN_POINT ( 'NONE',  ( 0.000000000000000000, 0.000000000000000000, 170.0000000000000000 ) ) ;
#51803=ORIENTED_EDGE ( 'NONE', *, *, #40585, .T. ) ;
#51807=VERTEX_POINT ( 'NONE', #57165 ) ;
#51808=CARTESIAN_POINT ( 'NONE',  ( 60.74750367560238828, -24.13405452624854775, 41.38025477438755928 ) ) ;
#51811=DIRECTION ( 'NONE',  ( 0.7227948638273878901, 0.6910626489868685329, 5.102127870520021228E-18 ) ) ;
#51813=LINE ( 'NONE', #3974, #59105 ) ;
#51830=DIRECTION ( 'NONE',  ( -0.8090169943749506709, 0.5877852522924686962, 0.000000000000000000 ) ) ;
#51835=LINE ( 'NONE', #25469, #13680 ) ;
#51839=DIRECTION ( 'NONE',  ( -0.000000000000000000, -0.000000000000000000, -1.000000000000000000 ) ) ;
#51844=CARTESIAN_POINT ( 'NONE',  ( 0.000000000000000000, 0.000000000000000000, 41.38025477438755928 ) ) ;
#51851=CARTESIAN_POINT ( 'NONE',  ( 24.79066879238609644, 3.228426989449657114, 0.000000000000000000 ) ) ;
#51856=EDGE_CURVE ( 'NONE', #66979, #13790, #61978, .T. ) ;
#51858=CARTESIAN_POINT ( 'NONE',  ( 55.14772863908626732, 34.40534879854737227, 40.00000000000003553 ) ) ;
#51867=DIRECTION ( 'NONE',  ( -0.000000000000000000, -0.000000000000000000, -1.000000000000000000 ) ) ;
#51869=EDGE_LOOP ( 'NONE', ( #17001, #38419, #53902, #121 ) ) ;
#51873=DIRECTION ( 'NONE',  ( 1.954612056407561701E-16, -1.558751100573736303E-16, 1.000000000000000000 ) ) ;
#51881=VERTEX_POINT ( 'NONE', #55779 ) ;
#51882=VERTEX_POINT ( 'NONE', #40624 ) ;
#51887=DIRECTION ( 'NONE',  ( 1.000000000000000000, 0.000000000000000000, 0.000000000000000000 ) ) ;
#51892=EDGE_LOOP ( 'NONE', ( #43003, #42201, #5895, #8240, #6725, #9279, #18742, #68903, #25626 ) ) ;
#51893=PRODUCT ( 'y3+', 'y3+', '', ( #56864 ) ) ;
#51896=AXIS2_PLACEMENT_3D ( 'NONE', #58522, #30778, #42359 ) ;
#51897=CIRCLE ( 'NONE', #58602, 65.00000000000000000 ) ;
#51902=DIRECTION ( 'NONE',  ( -0.4738686624730094610, 0.8805955318567321166, 0.000000000000000000 ) ) ;
#51911=DIRECTION ( 'NONE',  ( 0.000000000000000000, 0.000000000000000000, -1.000000000000000000 ) ) ;
#51913=LINE ( 'NONE', #3720, #20763 ) ;
#51921=FACE_OUTER_BOUND ( 'NONE', #18893, .T. ) ;
#51925=EDGE_LOOP ( 'NONE', ( #33173, #53677, #1364, #50355 ) ) ;
#51928=DIRECTION ( 'NONE',  ( 1.084727855779380319E-16, 2.252460601983949986E-16, 1.000000000000000000 ) ) ;
#51929=EDGE_CURVE ( 'NONE', #68939, #8769, #23033, .T. ) ;
#51938=EDGE_CURVE ( 'NONE', #6273, #56020, #8066, .T. ) ;
#51939=DIRECTION ( 'NONE',  ( -0.000000000000000000, -0.000000000000000000, -1.000000000000000000 ) ) ;
#51943=ORIENTED_EDGE ( 'NONE', *, *, #34796, .T. ) ;
#51944=CARTESIAN_POINT ( 'NONE',  ( 3.904274594239516283, -38.13466019661239415, 13.32819397642333392 ) ) ;
#51948=CARTESIAN_POINT ( 'NONE',  ( -65.36598343705435354, 0.000000000000000000, 41.38025477438755928 ) ) ;
#51956=CARTESIAN_POINT ( 'NONE',  ( -28.32746765835430836, -69.45586423092646555, 170.0000000000000000 ) ) ;
#51965=ORIENTED_EDGE ( 'NONE', *, *, #56523, .T. ) ;
#51968=CARTESIAN_POINT ( 'NONE',  ( 19.00668540189274225, -62.54164772954691642, 43.58025477438756212 ) ) ;
#51977=B_SPLINE_CURVE_WITH_KNOTS ( 'NONE', 3,
 ( #63759, #15567, #69013, #26808, #26467, #52506 ),
 .UNSPECIFIED., .F., .F.,
 ( 4, 2, 4 ),
 ( 0.03218937259408877899, 0.06469834484649478190, 0.09720731709890076400 ),
 .UNSPECIFIED. ) ;
#51983=CARTESIAN_POINT ( 'NONE',  ( 31.71171398032105060, -10.56647026444650272, 6.893342932883488317 ) ) ;
#51984=PLANE ( 'NONE',  #15276 ) ;
#51991=VECTOR ( 'NONE', #47037, 1000.000000000000114 ) ;
#51993=ORIENTED_EDGE ( 'NONE', *, *, #13358, .T. ) ;
#52002=EDGE_CURVE ( 'NONE', #7110, #56044, #21552, .T. ) ;
#52006=CONICAL_SURFACE ( 'NONE', #54232, 74.95140232871122521, 0.8777644062502172329 ) ;
#52034=CARTESIAN_POINT ( 'NONE',  ( -51.84164840787130402, -39.21024726209533640, 170.0000000000000000 ) ) ;
#52038=ADVANCED_FACE ( 'NONE', ( #36313 ), #65356, .T. ) ;
#52039=EDGE_CURVE ( 'NONE', #44366, #40373, #63394, .T. ) ;
#52041=ORIENTED_EDGE ( 'NONE', *, *, #23993, .T. ) ;
#52042=ADVANCED_FACE ( 'NONE', ( #9582 ), #63039, .F. ) ;
#52043=CARTESIAN_POINT ( 'NONE',  ( 16.92909695399013259, -28.82167194761692386, 6.893342934305374925 ) ) ;
#52050=AXIS2_PLACEMENT_3D ( 'NONE', #27942, #55370, #55730 ) ;
#52056=VERTEX_POINT ( 'NONE', #46509 ) ;
#52068=ORIENTED_EDGE ( 'NONE', *, *, #69261, .F. ) ;
#52078=ORIENTED_EDGE ( 'NONE', *, *, #21365, .F. ) ;
#52080=CARTESIAN_POINT ( 'NONE',  ( -49.45633250947157933, 14.94581096590798630, 26.66469104408688295 ) ) ;
#52082=CARTESIAN_POINT ( 'NONE',  ( -33.00963958485551331, 25.52799196440124163, 13.79046340968177553 ) ) ;
#52084=VECTOR ( 'NONE', #5701, 1000.000000000000000 ) ;
#52094=CIRCLE ( 'NONE', #58807, 65.00000000000000000 ) ;
#52095=CONICAL_SURFACE ( 'NONE', #36338, 74.95140232871122521, 0.8777644062502172329 ) ;
#52097=ORIENTED_EDGE ( 'NONE', *, *, #45878, .T. ) ;
#52102=VECTOR ( 'NONE', #31736, 1000.000000000000000 ) ;
#52116=EDGE_LOOP ( 'NONE', ( #55373, #40097, #39935, #43228 ) ) ;
#52121=EDGE_CURVE ( 'NONE', #13679, #35908, #23840, .T. ) ;
#52130=VECTOR ( 'NONE', #9335, 1000.000000000000000 ) ;
#52133=VECTOR ( 'NONE', #32440, 1000.000000000000000 ) ;
#52142=VECTOR ( 'NONE', #3320, 999.9999999999998863 ) ;
#52144=LINE ( 'NONE', #57083, #25297 ) ;
#52147=CIRCLE ( 'NONE', #44246, 25.12245591505646303 ) ;
#52149=ORIENTED_EDGE ( 'NONE', *, *, #50040, .F. ) ;
#52155=LINE ( 'NONE', #18500, #58053 ) ;
#52162=ADVANCED_FACE ( 'NONE', ( #48558 ), #27470, .T. ) ;
#52166=CARTESIAN_POINT ( 'NONE',  ( -63.33140416796853600, 16.18162651919394435, 43.58025477438756212 ) ) ;
#52167=ADVANCED_FACE ( 'NONE', ( #5337 ), #59127, .F. ) ;
#52181=ORIENTED_EDGE ( 'NONE', *, *, #37320, .F. ) ;
#52183=CARTESIAN_POINT ( 'NONE',  ( 48.39383208188444030, -43.94028683479018582, 41.38025477438755928 ) ) ;
#52192=CONICAL_SURFACE ( 'NONE', #16228, 65.00000000000000000, 0.7853981633974497223 ) ;
#52195=ORIENTED_EDGE ( 'NONE', *, *, #3730, .F. ) ;
#52197=AXIS2_PLACEMENT_3D ( 'NONE', #31780, #10317, #52203 ) ;
#52198=DIRECTION ( 'NONE',  ( -0.1342332658176522420, -0.9909497617679352555, 3.104767966278886959E-17 ) ) ;
#52203=DIRECTION ( 'NONE',  ( 1.000000000000000000, 0.000000000000000000, 0.000000000000000000 ) ) ;
#52222=CARTESIAN_POINT ( 'NONE',  ( -19.44450014243025748, 27.18813181980454274, 6.893342935626288970 ) ) ;
#52223=CARTESIAN_POINT ( 'NONE',  ( -84.49322488516129681, 0.000000000000000000, 43.58025477438756212 ) ) ;
#52226=CIRCLE ( 'NONE', #552, 24.99999999999985434 ) ;
#52240=ORIENTED_EDGE ( 'NONE', *, *, #40894, .F. ) ;
#52241=ORIENTED_EDGE ( 'NONE', *, *, #15120, .T. ) ;
#52242=VECTOR ( 'NONE', #43536, 1000.000000000000000 ) ;
#52246=EDGE_CURVE ( 'NONE', #2801, #49554, #34520, .T. ) ;
#52247=PLANE ( 'NONE',  #17281 ) ;
#52253=DIRECTION ( 'NONE',  ( -1.000000000000000000, 0.000000000000000000, 0.000000000000000000 ) ) ;
#52263=EDGE_CURVE ( 'NONE', #26979, #32844, #45046, .T. ) ;
#52267=DIRECTION ( 'NONE',  ( 0.4338837391175525693, 0.9009688679024218105, 5.102127870520019688E-18 ) ) ;
#52271=CARTESIAN_POINT ( 'NONE',  ( 0.000000000000000000, 0.000000000000000000, 43.58025477438756212 ) ) ;
#52277=VECTOR ( 'NONE', #9139, 1000.000000000000000 ) ;
#52279=ORIENTED_EDGE ( 'NONE', *, *, #18682, .F. ) ;
#52280=CARTESIAN_POINT ( 'NONE',  ( 56.42997683260146857, -32.25922681454192542, 40.00000000000003553 ) ) ;
#52283=CYLINDRICAL_SURFACE ( 'NONE', #65667, 65.36598343705435354 ) ;
#52288=ORIENTED_EDGE ( 'NONE', *, *, #24565, .T. ) ;
#52291=AXIS2_PLACEMENT_3D ( 'NONE', #44425, #33545, #6790 ) ;
#52297=B_SPLINE_CURVE_WITH_KNOTS ( 'NONE', 3,
 ( #29851, #19638, #62560, #14372 ),
 .UNSPECIFIED., .F., .F.,
 ( 4, 4 ),
 ( 0.1259919275528358917, 0.1829744153748748547 ),
 .UNSPECIFIED. ) ;
#52301=DIRECTION ( 'NONE',  ( -0.9195277725514544587, 0.3930250316539147803, 0.000000000000000000 ) ) ;
#52306=LINE ( 'NONE', #26269, #19056 ) ;
#52318=EDGE_CURVE ( 'NONE', #59777, #22589, #21270, .T. ) ;
#52325=VECTOR ( 'NONE', #29731, 1000.000000000000114 ) ;
#52329=CARTESIAN_POINT ( 'NONE',  ( 23.93060502292685499, -7.646171227524485303, 3.061616997868437868E-16 ) ) ;
#52339=CARTESIAN_POINT ( 'NONE',  ( -9.964117946889913924, 64.24592483216710548, 0.000000000000000000 ) ) ;
#52347=DIRECTION ( 'NONE',  ( -0.000000000000000000, -0.000000000000000000, -1.000000000000000000 ) ) ;
#52356=EDGE_CURVE ( 'NONE', #37187, #44519, #66530, .T. ) ;
#52371=LINE ( 'NONE', #18632, #38633 ) ;
#52387=EDGE_CURVE ( 'NONE', #51881, #26997, #5829, .T. ) ;
#52389=PLANE ( 'NONE',  #46818 ) ;
#52392=CONICAL_SURFACE ( 'NONE', #45673, 63.58578643762691485, 0.7853981633974497223 ) ;
#52393=ORIENTED_EDGE ( 'NONE', *, *, #55773, .T. ) ;
#52398=ORIENTED_EDGE ( 'NONE', *, *, #68753, .T. ) ;
#52399=CARTESIAN_POINT ( 'NONE',  ( 49.76301652092226391, -41.81676920493045202, 170.0000000000000000 ) ) ;
#52408=EDGE_CURVE ( 'NONE', #65008, #49164, #10517, .T. ) ;
#52416=EDGE_CURVE ( 'NONE', #39147, #49450, #32674, .T. ) ;
#52423=CARTESIAN_POINT ( 'NONE',  ( 9.133089864015637716, 32.15384528989822854, 6.893342932533050416 ) ) ;
#52430=AXIS2_PLACEMENT_3D ( 'NONE', #25442, #51811, #56129 ) ;
#52431=CARTESIAN_POINT ( 'NONE',  ( 24.39800339187929978, -60.26242556095670722, 41.38025477438755928 ) ) ;
#52432=LINE ( 'NONE', #42221, #48740 ) ;
#52444=AXIS2_PLACEMENT_3D ( 'NONE', #14061, #24977, #51011 ) ;
#52450=CARTESIAN_POINT ( 'NONE',  ( 57.84269237198510893, 33.10328505625795970, 34.48241795236666007 ) ) ;
#52453=ORIENTED_EDGE ( 'NONE', *, *, #38908, .T. ) ;
#52458=ORIENTED_EDGE ( 'NONE', *, *, #17307, .T. ) ;
#52461=ORIENTED_EDGE ( 'NONE', *, *, #17533, .F. ) ;
#52468=VECTOR ( 'NONE', #27315, 1000.000000000000000 ) ;
#52469=ADVANCED_FACE ( 'NONE', ( #53764 ), #32860, .T. ) ;
#52474=CARTESIAN_POINT ( 'NONE',  ( 0.000000000000000000, 0.000000000000000000, 0.000000000000000000 ) ) ;
#52480=CARTESIAN_POINT ( 'NONE',  ( 13.24564585880136036, -63.65041531508826012, 170.0000000000000000 ) ) ;
#52481=DIRECTION ( 'NONE',  ( 0.000000000000000000, 0.000000000000000000, 1.000000000000000000 ) ) ;
#52501=CARTESIAN_POINT ( 'NONE',  ( -34.96012151086515019, 55.23134702900888016, 41.38025477438755928 ) ) ;
#52506=CARTESIAN_POINT ( 'NONE',  ( -28.30427060690011132, -69.40159203110334829, 41.38025477438755928 ) ) ;
#52514=CARTESIAN_POINT ( 'NONE',  ( 41.26323044930809658, 6.217756198492188524, 13.79046340968177908 ) ) ;
#52516=VECTOR ( 'NONE', #40163, 1000.000000000000114 ) ;
#52520=CARTESIAN_POINT ( 'NONE',  ( 0.000000000000000000, 0.000000000000000000, 170.0000000000000000 ) ) ;
#52523=VECTOR ( 'NONE', #12722, 1000.000000000000000 ) ;
#52527=CARTESIAN_POINT ( 'NONE',  ( 24.39800339187933176, -60.26242556095669300, 170.0000000000000000 ) ) ;
#52542=LINE ( 'NONE', #31439, #23278 ) ;
#52551=EDGE_CURVE ( 'NONE', #2737, #41122, #39347, .T. ) ;
#52552=LINE ( 'NONE', #57494, #57248 ) ;
#52556=CARTESIAN_POINT ( 'NONE',  ( 0.000000000000000000, 0.000000000000000000, 0.000000000000000000 ) ) ;
#52557=ORIENTED_EDGE ( 'NONE', *, *, #52387, .F. ) ;
#52558=VERTEX_POINT ( 'NONE', #56210 ) ;
#52571=EDGE_CURVE ( 'NONE', #26997, #68407, #1088, .T. ) ;
#52573=B_SPLINE_CURVE_WITH_KNOTS ( 'NONE', 3,
 ( #9137, #52043, #63293, #3859, #15104, #11529 ),
 .UNSPECIFIED., .F., .F.,
 ( 4, 2, 4 ),
 ( 0.03218939915585350420, 0.06469836417558690045, 0.09720732919532029670 ),
 .UNSPECIFIED. ) ;
#52575=EDGE_CURVE ( 'NONE', #12492, #4891, #44259, .T. ) ;
#52581=DIRECTION ( 'NONE',  ( -0.000000000000000000, -0.000000000000000000, -1.000000000000000000 ) ) ;
#52595=PLANE ( 'NONE',  #45294 ) ;
#52608=CARTESIAN_POINT ( 'NONE',  ( 73.57152302639893549, 14.62167909564604429, 170.0000000000000000 ) ) ;
#52609=EDGE_LOOP ( 'NONE', ( #18573, #34527, #34689, #49496, #44680, #63663, #28924, #43537, #68070 ) ) ;
#52615=DIRECTION ( 'NONE',  ( -0.000000000000000000, -0.000000000000000000, -1.000000000000000000 ) ) ;
#52618=CARTESIAN_POINT ( 'NONE',  ( 18.89356949897823768, 62.19351277735707839, 40.00000000000003553 ) ) ;
#52626=VERTEX_POINT ( 'NONE', #40040 ) ;
#52628=EDGE_CURVE ( 'NONE', #56478, #35701, #61499, .T. ) ;
#52633=CARTESIAN_POINT ( 'NONE',  ( -39.09764951710989322, -70.01774562958885895, 133.5802547743875550 ) ) ;
#52638=B_SPLINE_CURVE_WITH_KNOTS ( 'NONE', 3,
 ( #65763, #6305, #44278, #39367 ),
 .UNSPECIFIED., .F., .F.,
 ( 4, 4 ),
 ( 9.900409499040004042E-07, 0.05658314289920114010 ),
 .UNSPECIFIED. ) ;
#52641=EDGE_LOOP ( 'NONE', ( #6029, #7904, #18602, #44437 ) ) ;
#52644=CARTESIAN_POINT ( 'NONE',  ( -64.61430802170482934, -7.070445451048283481, 40.00000000000003553 ) ) ;
#52649=ORIENTED_EDGE ( 'NONE', *, *, #5789, .F. ) ;
#52661=VERTEX_POINT ( 'NONE', #42112 ) ;
#52663=CARTESIAN_POINT ( 'NONE',  ( 19.84876914995301078, -26.89441360497561107, 6.893343212288940869 ) ) ;
#52665=CARTESIAN_POINT ( 'NONE',  ( -64.18058723658640474, -10.37664328995274055, 170.0000000000000000 ) ) ;
#52668=LINE ( 'NONE', #24233, #21006 ) ;
#52671=CONICAL_SURFACE ( 'NONE', #34726, 74.95140232871122521, 0.8777644062502172329 ) ;
#52672=ORIENTED_EDGE ( 'NONE', *, *, #67437, .T. ) ;
#52679=CARTESIAN_POINT ( 'NONE',  ( 75.00000000000000000, 1.250000000000011102, 43.58025477438756923 ) ) ;
#52686=CARTESIAN_POINT ( 'NONE',  ( -48.12872802574265307, 43.70867239603709464, 43.58025477438756923 ) ) ;
#52697=LINE ( 'NONE', #46388, #23833 ) ;
#52703=ADVANCED_FACE ( 'NONE', ( #3788 ), #25258, .T. ) ;
#52708=VECTOR ( 'NONE', #10075, 999.9999999999998863 ) ;
#52710=EDGE_LOOP ( 'NONE', ( #42896, #33492, #10335, #43339 ) ) ;
#52714=AXIS2_PLACEMENT_3D ( 'NONE', #15338, #11079, #36797 ) ;
#52718=DIRECTION ( 'NONE',  ( 0.7530714660036099684, 0.6579387259397136978, 0.000000000000000000 ) ) ;
#52724=EDGE_LOOP ( 'NONE', ( #10088, #19662, #23626, #51259 ) ) ;
#52733=DIRECTION ( 'NONE',  ( 0.000000000000000000, 0.000000000000000000, 1.000000000000000000 ) ) ;
#52734=DIRECTION ( 'NONE',  ( -1.000000000000000000, 1.421085471520200372E-14, 2.135044278125301096E-16 ) ) ;
#52735=CARTESIAN_POINT ( 'NONE',  ( 47.70222499156840712, -57.81185381817577706, 41.38025477438755928 ) ) ;
#52749=CARTESIAN_POINT ( 'NONE',  ( 19.40210676408052137, 63.75862954620263423, 34.48241823983693166 ) ) ;
#52753=CARTESIAN_POINT ( 'NONE',  ( 16.62148331457517969, -18.83783649008704586, 3.061616997868437868E-16 ) ) ;
#52755=CARTESIAN_POINT ( 'NONE',  ( 44.74620948996083314, -37.43371689815204917, 27.58472369426657522 ) ) ;
#52758=B_SPLINE_CURVE_WITH_KNOTS ( 'NONE', 3,
 ( #64742, #38001, #29528, #34489, #33779, #24271 ),
 .UNSPECIFIED., .F., .F.,
 ( 4, 2, 4 ),
 ( 0.03218933327099875868, 0.06469831623231236950, 0.09720729919362600113 ),
 .UNSPECIFIED. ) ;
#52770=DIRECTION ( 'NONE',  ( -0.000000000000000000, -0.000000000000000000, -1.000000000000000000 ) ) ;
#52777=ORIENTED_EDGE ( 'NONE', *, *, #38703, .F. ) ;
#52786=VERTEX_POINT ( 'NONE', #45229 ) ;
#52798=CARTESIAN_POINT ( 'NONE',  ( -26.07811460555695859, -76.21509903021815546, 73.58025477438756923 ) ) ;
#52803=EDGE_LOOP ( 'NONE', ( #31300, #21781, #5802, #15894, #1747, #58059, #36071, #23244, #33564 ) ) ;
#52808=DIRECTION ( 'NONE',  ( -0.000000000000000000, -0.000000000000000000, -1.000000000000000000 ) ) ;
#52819=EDGE_LOOP ( 'NONE', ( #30700, #38801, #9363, #42867 ) ) ;
#52827=CARTESIAN_POINT ( 'NONE',  ( 0.000000000000000000, 0.000000000000000000, 170.0000000000000000 ) ) ;
#52834=DIRECTION ( 'NONE',  ( 1.156482317317871478E-16, 0.000000000000000000, 1.000000000000000000 ) ) ;
#52840=AXIS2_PLACEMENT_3D ( 'NONE', #20667, #3806, #4158 ) ;
#52847=CARTESIAN_POINT ( 'NONE',  ( -10.00000000000000000, 0.000000000000000000, 0.000000000000000000 ) ) ;
#52850=ADVANCED_FACE ( 'NONE', ( #57438 ), #36676, .F. ) ;
#52872=FACE_OUTER_BOUND ( 'NONE', #63731, .T. ) ;
#52881=ORIENTED_EDGE ( 'NONE', *, *, #52246, .F. ) ;
#52887=B_SPLINE_CURVE_WITH_KNOTS ( 'NONE', 3,
 ( #6588, #50542, #28034, #60742, #29096, #6932 ),
 .UNSPECIFIED., .F., .F.,
 ( 4, 2, 4 ),
 ( 1.095770181096429506E-06, 0.03239442681617710207, 0.06478775786217309818 ),
 .UNSPECIFIED. ) ;
#52894=VERTEX_POINT ( 'NONE', #27841 ) ;
#52916=CARTESIAN_POINT ( 'NONE',  ( 34.43940527065477397, -66.63700071734618291, 43.58025477438756212 ) ) ;
#52920=CARTESIAN_POINT ( 'NONE',  ( 0.000000000000000000, 0.000000000000000000, 0.000000000000000000 ) ) ;
#52923=CARTESIAN_POINT ( 'NONE',  ( 0.000000000000000000, 0.000000000000000000, 170.0000000000000000 ) ) ;
#52951=ADVANCED_FACE ( 'NONE', ( #65919 ), #33976, .T. ) ;
#52953=EDGE_LOOP ( 'NONE', ( #15325, #10918, #48648, #62316, #51277, #5383, #13816, #60848, #30044, #59410, #48698, #55893, #46021, #51512, #41882, #23951, #35596, #532, #67397, #68587, #57855, #10450, #53438, #19210, #13496, #6190, #24357, #50553, #15447, #37298, #29836, #33011, #67876, #39220, #65167, #36704, #57142, #26605, #724, #65777, #64421, #52241, #47442, #29032, #45330, #51539, #44718, #58329, #12586, #30853, #4906, #2, #2807, #5411, #32437, #13931, #37845, #56358, #64847, #51332, #5172, #29812, #53990, #30479, #58382, #30828, #28074, #19816, #37007, #36137, #259, #30417, #12691, #39339, #42336, #49637, #12399, #25858, #37778, #8190, #58917, #20310, #8474, #67630, #59511, #46715, #23440, #25354, #3247, #33888, #61546, #52149, #29579, #49071, #69341, #61503, #47015, #22164, #42589, #15525, #1684, #1269, #40512, #61618, #60242, #56726, #425, #55097, #23123, #40044, #49806, #66071, #12759, #4619, #49891, #54144, #38667, #20042, #23704, #32304, #63641, #67330, #68094, #9733, #8090, #10509, #3758, #12080, #8946, #50592, #31456, #62050, #731, #68619, #28470, #47983, #16962, #57357, #19641, #56274, #12461 ) ) ;
#52955=DIRECTION ( 'NONE',  ( -0.000000000000000000, -0.000000000000000000, 1.000000000000000000 ) ) ;
#52958=DIRECTION ( 'NONE',  ( -0.000000000000000000, -0.000000000000000000, -1.000000000000000000 ) ) ;
#52959=CARTESIAN_POINT ( 'NONE',  ( 61.91366885787729046, 28.42865614899000448, 41.38025477438755928 ) ) ;
#52960=CARTESIAN_POINT ( 'NONE',  ( -64.18058723658653264, 10.37664328995176888, 43.58025477438756923 ) ) ;
#52961=ORIENTED_EDGE ( 'NONE', *, *, #43446, .F. ) ;
#52962=CARTESIAN_POINT ( 'NONE',  ( 0.000000000000000000, 0.000000000000000000, 170.0000000000000000 ) ) ;
#52972=CIRCLE ( 'NONE', #21542, 65.36598343705435354 ) ;
#52975=DIRECTION ( 'NONE',  ( -1.000000000000000000, 0.000000000000000000, 0.000000000000000000 ) ) ;
#52977=AXIS2_PLACEMENT_3D ( 'NONE', #11288, #64769, #22902 ) ;
#52981=DIRECTION ( 'NONE',  ( 0.4738686624729966379, 0.8805955318567391110, 0.000000000000000000 ) ) ;
#52988=CARTESIAN_POINT ( 'NONE',  ( 39.54205320694339321, 51.58901073076764021, 40.00000000000003553 ) ) ;
#52998=EDGE_LOOP ( 'NONE', ( #36045, #37406, #44427, #19359, #38636, #35284, #23544, #48167, #49480 ) ) ;
#52999=CARTESIAN_POINT ( 'NONE',  ( -59.09450113343203270, -27.07101652673575032, 40.00000000000003553 ) ) ;
#53000=CARTESIAN_POINT ( 'NONE',  ( 40.56810594101300893, -52.87564016363982233, 34.48241795236665297 ) ) ;
#53006=LINE ( 'NONE', #10447, #63723 ) ;
#53008=EDGE_LOOP ( 'NONE', ( #17921, #39583, #36764, #66662 ) ) ;
#53011=DIRECTION ( 'NONE',  ( 1.000000000000000000, 0.000000000000000000, 0.000000000000000000 ) ) ;
#53012=CARTESIAN_POINT ( 'NONE',  ( -16.43619359402603664, -18.99971924381128474, 3.061616997868437868E-16 ) ) ;
#53016=EDGE_CURVE ( 'NONE', #1969, #28828, #10151, .T. ) ;
#53022=AXIS2_PLACEMENT_3D ( 'NONE', #39390, #50296, #6682 ) ;
#53031=CONICAL_SURFACE ( 'NONE', #20444, 65.00000000000000000, 0.7853981633974497223 ) ;
#53034=AXIS2_PLACEMENT_3D ( 'NONE', #64686, #27383, #54812 ) ;
#53036=EDGE_CURVE ( 'NONE', #9288, #42925, #3130, .T. ) ;
#53038=EDGE_CURVE ( 'NONE', #308, #28975, #29498, .T. ) ;
#53040=DIRECTION ( 'NONE',  ( -1.156482317317871232E-16, -0.000000000000000000, -1.000000000000000000 ) ) ;
#53041=CARTESIAN_POINT ( 'NONE',  ( -53.60725281709859757, -37.40286400928327026, 43.58025477438756212 ) ) ;
#53045=ORIENTED_EDGE ( 'NONE', *, *, #32383, .T. ) ;
#53046=CARTESIAN_POINT ( 'NONE',  ( -58.33959211650994803, -29.48226216511402242, 41.38025477438755928 ) ) ;
#53047=VERTEX_POINT ( 'NONE', #41101 ) ;
#53055=CARTESIAN_POINT ( 'NONE',  ( -7.486743542469090684, -64.58150799671139453, 170.0000000000000000 ) ) ;
#53056=ORIENTED_EDGE ( 'NONE', *, *, #5241, .F. ) ;
#53070=DIRECTION ( 'NONE',  ( 0.000000000000000000, 0.000000000000000000, 1.000000000000000000 ) ) ;
#53085=CARTESIAN_POINT ( 'NONE',  ( 0.000000000000000000, 0.000000000000000000, 170.0000000000000000 ) ) ;
#53091=ORIENTED_EDGE ( 'NONE', *, *, #34475, .T. ) ;
#53097=CARTESIAN_POINT ( 'NONE',  ( 0.000000000000000000, 0.000000000000000000, 170.0000000000000000 ) ) ;
#53102=ORIENTED_EDGE ( 'NONE', *, *, #36250, .T. ) ;
#53108=CARTESIAN_POINT ( 'NONE',  ( -41.43037391101678679, 4.983853614416524636, 13.79046340968177731 ) ) ;
#53109=DIRECTION ( 'NONE',  ( -1.000000000000000000, 0.000000000000000000, 0.000000000000000000 ) ) ;
#53115=CARTESIAN_POINT ( 'NONE',  ( -62.66631205405186478, 18.59153367093363229, 43.58025477438756212 ) ) ;
#53120=CIRCLE ( 'NONE', #29539, 65.36598343705435354 ) ;
#53152=CARTESIAN_POINT ( 'NONE',  ( -15.45727656667583005, -73.34020256436187424, 41.38025477438755928 ) ) ;
#53169=AXIS2_PLACEMENT_3D ( 'NONE', #35111, #44266, #56219 ) ;
#53176=EDGE_CURVE ( 'NONE', #67695, #44050, #52297, .T. ) ;
#53180=AXIS2_PLACEMENT_3D ( 'NONE', #38308, #60469, #10884 ) ;
#53181=ADVANCED_FACE ( 'NONE', ( #34792 ), #9094, .F. ) ;
#53199=EDGE_CURVE ( 'NONE', #13968, #37838, #21358, .T. ) ;
#53206=EDGE_LOOP ( 'NONE', ( #5997, #26843, #16999, #50031 ) ) ;
#53219=PLANE ( 'NONE',  #1682 ) ;
#53222=VECTOR ( 'NONE', #7488, 1000.000000000000000 ) ;
#53228=CARTESIAN_POINT ( 'NONE',  ( 55.14772863908626732, 34.40534879854737227, 170.0000000000000000 ) ) ;
#53230=VERTEX_POINT ( 'NONE', #10806 ) ;
#53242=ADVANCED_FACE ( 'NONE', ( #5528 ), #28392, .T. ) ;
#53255=EDGE_LOOP ( 'NONE', ( #50539, #58336, #44637, #8246, #17399, #20605, #51193, #18101, #31137 ) ) ;
#53257=EDGE_CURVE ( 'NONE', #41387, #47508, #66626, .T. ) ;
#53265=EDGE_LOOP ( 'NONE', ( #31152, #44671, #12503, #39415 ) ) ;
#53266=AXIS2_PLACEMENT_3D ( 'NONE', #46026, #39716, #39368 ) ;
#53278=ORIENTED_EDGE ( 'NONE', *, *, #32863, .T. ) ;
#53286=ORIENTED_EDGE ( 'NONE', *, *, #32135, .T. ) ;
#53293=CARTESIAN_POINT ( 'NONE',  ( 0.000000000000000000, 0.000000000000000000, 0.000000000000000000 ) ) ;
#53298=DIRECTION ( 'NONE',  ( -1.000000000000000000, 0.000000000000000000, 0.000000000000000000 ) ) ;
#53302=ORIENTED_EDGE ( 'NONE', *, *, #18054, .F. ) ;
#53318=VECTOR ( 'NONE', #10401, 1000.000000000000000 ) ;
#53326=ORIENTED_EDGE ( 'NONE', *, *, #40419, .F. ) ;
#53329=PLANE ( 'NONE',  #18292 ) ;
#53331=CARTESIAN_POINT ( 'NONE',  ( 26.69682282325795697, -59.27986298182186431, 41.38025477438755928 ) ) ;
#53344=EDGE_CURVE ( 'NONE', #36414, #4959, #44093, .T. ) ;
#53346=DIRECTION ( 'NONE',  ( -0.000000000000000000, -0.000000000000000000, -1.000000000000000000 ) ) ;
#53350=LINE ( 'NONE', #20665, #52468 ) ;
#53351=CARTESIAN_POINT ( 'NONE',  ( -13.90880041226882824, 35.72171523751327982, 13.32819397642331971 ) ) ;
#53371=ORIENTED_EDGE ( 'NONE', *, *, #69541, .F. ) ;
#53372=CARTESIAN_POINT ( 'NONE',  ( -63.73419499958981049, -12.83646726144931449, 43.58025477438756923 ) ) ;
#53380=ORIENTED_EDGE ( 'NONE', *, *, #32135, .F. ) ;
#53384=FACE_OUTER_BOUND ( 'NONE', #69436, .T. ) ;
#53391=LINE ( 'NONE', #37578, #52242 ) ;
#53395=DIRECTION ( 'NONE',  ( -0.000000000000000000, -0.000000000000000000, -1.000000000000000000 ) ) ;
#53411=AXIS2_PLACEMENT_3D ( 'NONE', #59587, #520, #5450 ) ;
#53418=VECTOR ( 'NONE', #42687, 1000.000000000000000 ) ;
#53419=CARTESIAN_POINT ( 'NONE',  ( 55.61348889666937367, 50.24791103897128863, 41.38025477438755928 ) ) ;
#53421=LINE ( 'NONE', #5254, #40892 ) ;
#53426=EDGE_CURVE ( 'NONE', #47929, #23514, #12205, .T. ) ;
#53428=DIRECTION ( 'NONE',  ( -0.9989930665413151445, 0.04486483035050447404, 5.102127870520021999E-18 ) ) ;
#53435=ORIENTED_EDGE ( 'NONE', *, *, #24333, .F. ) ;
#53438=ORIENTED_EDGE ( 'NONE', *, *, #44051, .F. ) ;
#53444=CARTESIAN_POINT ( 'NONE',  ( -19.56458807131854627, 15.75959024859389324, 0.000000000000000000 ) ) ;
#53447=ORIENTED_EDGE ( 'NONE', *, *, #25598, .F. ) ;
#53455=CARTESIAN_POINT ( 'NONE',  ( -65.20298343242136241, 4.613322252417249913, 3.125053320693571104E-16 ) ) ;
#53456=VECTOR ( 'NONE', #68653, 1000.000000000000000 ) ;
#53457=DIRECTION ( 'NONE',  ( -0.000000000000000000, -0.000000000000000000, -1.000000000000000000 ) ) ;
#53467=VECTOR ( 'NONE', #68367, 1000.000000000000000 ) ;
#53475=VECTOR ( 'NONE', #45843, 1000.000000000000227 ) ;
#53486=DIRECTION ( 'NONE',  ( -0.000000000000000000, -0.000000000000000000, -1.000000000000000000 ) ) ;
#53488=EDGE_CURVE ( 'NONE', #29070, #34941, #67409, .T. ) ;
#53489=CARTESIAN_POINT ( 'NONE',  ( 0.000000000000000000, 0.000000000000000000, 170.0000000000000000 ) ) ;
#53490=CARTESIAN_POINT ( 'NONE',  ( 39.48989012082040517, 13.48566859677802299, 13.79046340968177908 ) ) ;
#53495=EDGE_CURVE ( 'NONE', #52786, #21788, #48769, .T. ) ;
#53505=CARTESIAN_POINT ( 'NONE',  ( 21.98745393275193294, 71.71550996510526943, 170.0000000000000000 ) ) ;
#53513=VERTEX_POINT ( 'NONE', #34712 ) ;
#53514=EDGE_CURVE ( 'NONE', #61455, #9355, #60984, .T. ) ;
#53526=VERTEX_POINT ( 'NONE', #39974 ) ;
#53528=B_SPLINE_CURVE_WITH_KNOTS ( 'NONE', 3,
 ( #40748, #34460, #67845, #2778, #18957, #3469 ),
 .UNSPECIFIED., .F., .F.,
 ( 4, 2, 4 ),
 ( 1.095770181118997428E-06, 0.03239442681617710901, 0.06478775786217309818 ),
 .UNSPECIFIED. ) ;
#53531=DIRECTION ( 'NONE',  ( 0.000000000000000000, 0.000000000000000000, 1.000000000000000000 ) ) ;
#53533=CARTESIAN_POINT ( 'NONE',  ( 7.484861546145031852, 64.56761454192836425, 133.5802547743875550 ) ) ;
#53534=VERTEX_POINT ( 'NONE', #18524 ) ;
#53538=DIRECTION ( 'NONE',  ( 1.000000000000000000, 0.000000000000000000, 0.000000000000000000 ) ) ;
#53544=VERTEX_POINT ( 'NONE', #24507 ) ;
#53546=DIRECTION ( 'NONE',  ( -0.9959742939952397345, 0.08963930890342655666, 0.000000000000000000 ) ) ;
#53548=CARTESIAN_POINT ( 'NONE',  ( -44.00727179482577611, 47.83680621839560132, 40.00000000000003553 ) ) ;
#53557=VERTEX_POINT ( 'NONE', #5445 ) ;
#53570=ORIENTED_EDGE ( 'NONE', *, *, #45268, .F. ) ;
#53591=FACE_OUTER_BOUND ( 'NONE', #53206, .T. ) ;
#53594=ADVANCED_FACE ( 'NONE', ( #36779 ), #4078, .F. ) ;
#53599=EDGE_CURVE ( 'NONE', #26979, #43082, #20271, .T. ) ;
#53601=AXIS2_PLACEMENT_3D ( 'NONE', #22510, #16875, #38695 ) ;
#53602=CARTESIAN_POINT ( 'NONE',  ( -38.12207019443992095, 16.97122609182251196, 13.79046412329103077 ) ) ;
#53603=B_SPLINE_CURVE_WITH_KNOTS ( 'NONE', 3,
 ( #38587, #60031, #49470, #1305 ),
 .UNSPECIFIED., .F., .F.,
 ( 4, 4 ),
 ( 9.900409499016060538E-07, 0.05658314289920114704 ),
 .UNSPECIFIED. ) ;
#53606=ORIENTED_EDGE ( 'NONE', *, *, #15549, .T. ) ;
#53632=CARTESIAN_POINT ( 'NONE',  ( 0.000000000000000000, 0.000000000000000000, 43.58025477438756212 ) ) ;
#53639=CARTESIAN_POINT ( 'NONE',  ( -27.38060252176762077, -26.82905652391248807, 13.32819397642333215 ) ) ;
#53653=EDGE_CURVE ( 'NONE', #61883, #6204, #6126, .T. ) ;
#53666=EDGE_CURVE ( 'NONE', #41122, #55255, #18784, .T. ) ;
#53670=LINE ( 'NONE', #27638, #46870 ) ;
#53677=ORIENTED_EDGE ( 'NONE', *, *, #4191, .F. ) ;
#53688=DIRECTION ( 'NONE',  ( -0.000000000000000000, -0.000000000000000000, -1.000000000000000000 ) ) ;
#53701=ORIENTED_EDGE ( 'NONE', *, *, #36445, .T. ) ;
#53703=CARTESIAN_POINT ( 'NONE',  ( 40.56810615702079303, 52.87564043450657181, 34.48241824003539335 ) ) ;
#53711=AXIS2_PLACEMENT_3D ( 'NONE', #23643, #44389, #35231 ) ;
#53713=VECTOR ( 'NONE', #37637, 1000.000000000000227 ) ;
#53734=EDGE_CURVE ( 'NONE', #42734, #37998, #59860, .T. ) ;
#53739=CARTESIAN_POINT ( 'NONE',  ( 57.30278335769610010, -48.40406511297319980, 170.0000000000000000 ) ) ;
#53745=EDGE_CURVE ( 'NONE', #11417, #25097, #31757, .T. ) ;
#53764=FACE_OUTER_BOUND ( 'NONE', #54786, .T. ) ;
#53769=DIRECTION ( 'NONE',  ( 0.000000000000000000, 0.000000000000000000, 1.000000000000000000 ) ) ;
#53777=EDGE_LOOP ( 'NONE', ( #63959, #50366, #9555, #51359 ) ) ;
#53779=CYLINDRICAL_SURFACE ( 'NONE', #54337, 65.36598343705435354 ) ;
#53780=ORIENTED_EDGE ( 'NONE', *, *, #66678, .F. ) ;
#53786=ORIENTED_EDGE ( 'NONE', *, *, #17427, .T. ) ;
#53789=DIRECTION ( 'NONE',  ( 0.9362348706397369824, 0.3513748240813435175, 0.000000000000000000 ) ) ;
#53794=CARTESIAN_POINT ( 'NONE',  ( 6.564829507346109594, 24.24955267099648992, 3.061616997868437868E-16 ) ) ;
#53796=EDGE_CURVE ( 'NONE', #25958, #17560, #20600, .T. ) ;
#53797=CARTESIAN_POINT ( 'NONE',  ( -53.60725281709914469, 37.40286400928249577, 43.58025477438756212 ) ) ;
#53798=CARTESIAN_POINT ( 'NONE',  ( 0.000000000000000000, 0.000000000000000000, 2.000000000000000000 ) ) ;
#53802=AXIS2_PLACEMENT_3D ( 'NONE', #63545, #34837, #55935 ) ;
#53809=VECTOR ( 'NONE', #63521, 1000.000000000000000 ) ;
#53814=ORIENTED_EDGE ( 'NONE', *, *, #53036, .F. ) ;
#53819=EDGE_LOOP ( 'NONE', ( #64678, #30124, #45342, #59961, #64219 ) ) ;
#53828=FACE_OUTER_BOUND ( 'NONE', #1418, .T. ) ;
#53835=VECTOR ( 'NONE', #18319, 1000.000000000000000 ) ;
#53839=CARTESIAN_POINT ( 'NONE',  ( 57.25833571151868284, 48.36523237396223607, 41.38025477438755928 ) ) ;
#53851=ORIENTED_EDGE ( 'NONE', *, *, #18014, .F. ) ;
#53852=DIRECTION ( 'NONE',  ( -0.000000000000000000, -0.000000000000000000, -1.000000000000000000 ) ) ;
#53863=CARTESIAN_POINT ( 'NONE',  ( -29.87147652227456263, 100.0000000000000000, 73.58025477438756923 ) ) ;
#53865=ORIENTED_EDGE ( 'NONE', *, *, #63141, .T. ) ;
#53869=B_SPLINE_CURVE_WITH_KNOTS ( 'NONE', 3,
 ( #31633, #26020, #26364, #57687, #62622, #8815 ),
 .UNSPECIFIED., .F., .F.,
 ( 4, 2, 4 ),
 ( 1.095770181108978510E-06, 0.03239442681617710901, 0.06478775786217311206 ),
 .UNSPECIFIED. ) ;
#53870=AXIS2_PLACEMENT_3D ( 'NONE', #51026, #19012, #3875 ) ;
#53873=EDGE_CURVE ( 'NONE', #13204, #44574, #59855, .T. ) ;
#53884=ORIENTED_EDGE ( 'NONE', *, *, #46306, .F. ) ;
#53887=EDGE_CURVE ( 'NONE', #35508, #64034, #12738, .T. ) ;
#53896=ORIENTED_EDGE ( 'NONE', *, *, #14910, .F. ) ;
#53902=ORIENTED_EDGE ( 'NONE', *, *, #32783, .T. ) ;
#53908=CARTESIAN_POINT ( 'NONE',  ( -40.27405704175634327, 63.28161525591265502, 170.0000000000000000 ) ) ;
#53910=VERTEX_POINT ( 'NONE', #17663 ) ;
#53912=DIRECTION ( 'NONE',  ( -1.000000000000000000, -2.309263891220325604E-14, 2.135044278125301096E-16 ) ) ;
#53916=DIRECTION ( 'NONE',  ( -0.000000000000000000, -0.000000000000000000, 1.000000000000000000 ) ) ;
#53919=ORIENTED_EDGE ( 'NONE', *, *, #25435, .F. ) ;
#53920=AXIS2_PLACEMENT_3D ( 'NONE', #22033, #32932, #12186 ) ;
#53945=DIRECTION ( 'NONE',  ( -0.000000000000000000, -0.000000000000000000, -1.000000000000000000 ) ) ;
#53951=CARTESIAN_POINT ( 'NONE',  ( 0.000000000000000000, 0.000000000000000000, 0.000000000000000000 ) ) ;
#53957=CARTESIAN_POINT ( 'NONE',  ( -65.36598343705435354, 0.000000000000000000, 41.38025477438755928 ) ) ;
#53962=EDGE_CURVE ( 'NONE', #2204, #43521, #13347, .T. ) ;
#53967=CARTESIAN_POINT ( 'NONE',  ( -50.88541732109811022, 55.03078243218087806, 41.38025477438755928 ) ) ;
#53990=ORIENTED_EDGE ( 'NONE', *, *, #18185, .F. ) ;
#53998=VERTEX_POINT ( 'NONE', #21879 ) ;
#54001=CARTESIAN_POINT ( 'NONE',  ( -20.93485882276955579, 13.66498028065538861, 0.000000000000000000 ) ) ;
#54009=AXIS2_PLACEMENT_3D ( 'NONE', #58912, #38151, #54675 ) ;
#54012=DIRECTION ( 'NONE',  ( 1.000000000000000000, 0.000000000000000000, 0.000000000000000000 ) ) ;
#54015=AXIS2_PLACEMENT_3D ( 'NONE', #11777, #33252, #54687 ) ;
#54021=EDGE_LOOP ( 'NONE', ( #55460, #37335, #60376, #66930 ) ) ;
#54023=ORIENTED_EDGE ( 'NONE', *, *, #63212, .F. ) ;
#54033=CIRCLE ( 'NONE', #59614, 24.99999999999985434 ) ;
#54048=VERTEX_POINT ( 'NONE', #24602 ) ;
#54056=DIRECTION ( 'NONE',  ( 0.6234898018587431423, -0.7818314824680220321, 0.000000000000000000 ) ) ;
#54057=CARTESIAN_POINT ( 'NONE',  ( -74.75133697335800775, -5.472689625387135770, 41.38025477438755928 ) ) ;
#54058=CARTESIAN_POINT ( 'NONE',  ( -23.85457283326427813, -7.880174245944393974, 3.061616997868437868E-16 ) ) ;
#54061=ADVANCED_FACE ( 'NONE', ( #14716 ), #24937, .T. ) ;
#54067=EDGE_CURVE ( 'NONE', #31009, #40830, #62121, .T. ) ;
#54072=CARTESIAN_POINT ( 'NONE',  ( -64.61430802170482934, -7.070445451048283481, 170.0000000000000000 ) ) ;
#54075=AXIS2_PLACEMENT_3D ( 'NONE', #53798, #38331, #54141 ) ;
#54080=ORIENTED_EDGE ( 'NONE', *, *, #34495, .F. ) ;
#54081=CARTESIAN_POINT ( 'NONE',  ( -68.11501976657811497, -31.41506934893937952, 43.58025477438756212 ) ) ;
#54085=EDGE_LOOP ( 'NONE', ( #37741, #56818, #24620, #14089 ) ) ;
#54093=CARTESIAN_POINT ( 'NONE',  ( -11.01093400780220932, -22.58090174195397992, 0.000000000000000000 ) ) ;
#54099=CARTESIAN_POINT ( 'NONE',  ( 74.01791526339567895, -12.16185512414844716, 170.0000000000000000 ) ) ;
#54102=DIRECTION ( 'NONE',  ( -1.000000000000000000, 0.000000000000000000, 0.000000000000000000 ) ) ;
#54106=CARTESIAN_POINT ( 'NONE',  ( 0.000000000000000000, 0.000000000000000000, 0.000000000000000000 ) ) ;
#54108=DIRECTION ( 'NONE',  ( -0.000000000000000000, -0.000000000000000000, 1.000000000000000000 ) ) ;
#54112=CARTESIAN_POINT ( 'NONE',  ( 7.484861546145933353, -64.56761454192826477, 170.0000000000000000 ) ) ;
#54118=DIRECTION ( 'NONE',  ( -0.000000000000000000, 0.000000000000000000, -1.000000000000000000 ) ) ;
#54119=ORIENTED_EDGE ( 'NONE', *, *, #58057, .F. ) ;
#54121=EDGE_CURVE ( 'NONE', #14469, #13950, #37200, .T. ) ;
#54126=AXIS2_PLACEMENT_3D ( 'NONE', #14085, #57001, #8819 ) ;
#54129=FACE_OUTER_BOUND ( 'NONE', #4770, .T. ) ;
#54130=VECTOR ( 'NONE', #30244, 1000.000000000000000 ) ;
#54134=DIRECTION ( 'NONE',  ( -0.000000000000000000, 0.000000000000000000, -1.000000000000000000 ) ) ;
#54140=CARTESIAN_POINT ( 'NONE',  ( -63.33140416796831573, -16.18162651919485739, 43.58025477438756212 ) ) ;
#54141=DIRECTION ( 'NONE',  ( 1.000000000000000000, 0.000000000000000000, -0.000000000000000000 ) ) ;
#54142=LINE ( 'NONE', #35677, #63826 ) ;
#54144=ORIENTED_EDGE ( 'NONE', *, *, #22305, .F. ) ;
#54146=LINE ( 'NONE', #37641, #20439 ) ;
#54152=ORIENTED_EDGE ( 'NONE', *, *, #27843, .T. ) ;
#54158=VERTEX_POINT ( 'NONE', #254 ) ;
#54161=CARTESIAN_POINT ( 'NONE',  ( -67.03031041878421092, -33.66749151869542089, 170.0000000000000000 ) ) ;
#54163=DIRECTION ( 'NONE',  ( 0.000000000000000000, -0.000000000000000000, -1.000000000000000000 ) ) ;
#54166=CARTESIAN_POINT ( 'NONE',  ( -56.44201257846630426, 32.26641783793562723, 170.0000000000000000 ) ) ;
#54167=B_SPLINE_CURVE_WITH_KNOTS ( 'NONE', 3,
 ( #63624, #58325, #48436, #37567 ),
 .UNSPECIFIED., .F., .F.,
 ( 4, 4 ),
 ( 9.900409499088329389E-07, 0.05658314289920116785 ),
 .UNSPECIFIED. ) ;
#54177=DIRECTION ( 'NONE',  ( -1.000000000000000000, 0.000000000000000000, 0.000000000000000000 ) ) ;
#54178=ORIENTED_EDGE ( 'NONE', *, *, #21593, .F. ) ;
#54183=DIRECTION ( 'NONE',  ( 0.000000000000000000, -5.102127870520020458E-18, -1.000000000000000000 ) ) ;
#54205=LINE ( 'NONE', #12367, #29661 ) ;
#54206=VERTEX_POINT ( 'NONE', #10817 ) ;
#54207=EDGE_LOOP ( 'NONE', ( #43894, #31277, #42128, #5143, #27492, #1501, #36879, #54152, #2228 ) ) ;
#54217=ORIENTED_EDGE ( 'NONE', *, *, #4297, .T. ) ;
#54218=EDGE_CURVE ( 'NONE', #45135, #46531, #11854, .T. ) ;
#54221=DIRECTION ( 'NONE',  ( -1.000000000000000000, 0.000000000000000000, 0.000000000000000000 ) ) ;
#54232=AXIS2_PLACEMENT_3D ( 'NONE', #26876, #63478, #47624 ) ;
#54234=CARTESIAN_POINT ( 'NONE',  ( -63.73419499958998813, 12.83646726144834993, 170.0000000000000000 ) ) ;
#54238=EDGE_CURVE ( 'NONE', #57335, #40013, #23475, .T. ) ;
#54239=DIRECTION ( 'NONE',  ( -1.000000000000000000, 0.000000000000000000, 0.000000000000000000 ) ) ;
#54244=FACE_OUTER_BOUND ( 'NONE', #12604, .T. ) ;
#54246=ORIENTED_EDGE ( 'NONE', *, *, #44051, .T. ) ;
#54268=DIRECTION ( 'NONE',  ( 1.000000000000000000, 0.000000000000000000, 0.000000000000000000 ) ) ;
#54274=DIRECTION ( 'NONE',  ( 0.000000000000000000, 0.000000000000000000, 1.000000000000000000 ) ) ;
#54276=CARTESIAN_POINT ( 'NONE',  ( 0.000000000000000000, 0.000000000000000000, 0.000000000000000000 ) ) ;
#54287=LINE ( 'NONE', #22646, #40846 ) ;
#54298=EDGE_CURVE ( 'NONE', #8257, #14673, #52887, .T. ) ;
#54300=DIRECTION ( 'NONE',  ( 0.000000000000000000, 0.000000000000000000, 1.000000000000000000 ) ) ;
#54314=AXIS2_PLACEMENT_3D ( 'NONE', #21769, #11211, #32679 ) ;
#54319=DIRECTION ( 'NONE',  ( -1.000000000000000000, 0.000000000000000000, 0.000000000000000000 ) ) ;
#54320=PLANE ( 'NONE',  #60213 ) ;
#54321=ORIENTED_EDGE ( 'NONE', *, *, #11596, .T. ) ;
#54329=ORIENTED_EDGE ( 'NONE', *, *, #28997, .F. ) ;
#54332=DIRECTION ( 'NONE',  ( 0.1342332658176522420, 0.9909497617679351444, 0.000000000000000000 ) ) ;
#54337=AXIS2_PLACEMENT_3D ( 'NONE', #7005, #59412, #27403 ) ;
#54342=ORIENTED_EDGE ( 'NONE', *, *, #39922, .F. ) ;
#54354=CARTESIAN_POINT ( 'NONE',  ( -26.83517958587656338, 59.60356471962913361, 41.38025477438755928 ) ) ;
#54361=ADVANCED_FACE ( 'NONE', ( #44914 ), #61097, .T. ) ;
#54363=DIRECTION ( 'NONE',  ( -1.000000000000000000, 0.000000000000000000, 0.000000000000000000 ) ) ;
#54365=ORIENTED_EDGE ( 'NONE', *, *, #3558, .T. ) ;
#54367=PLANE ( 'NONE',  #4603 ) ;
#54374=CARTESIAN_POINT ( 'NONE',  ( 9.068001488962039502, 57.63052748569040062, 27.58472315868180402 ) ) ;
#54393=VERTEX_POINT ( 'NONE', #3731 ) ;
#54412=AXIS2_PLACEMENT_3D ( 'NONE', #44159, #43117, #22369 ) ;
#54417=CARTESIAN_POINT ( 'NONE',  ( -17.90772993695011550, -72.84144224619156205, 170.0000000000000000 ) ) ;
#54422=ADVANCED_FACE ( 'NONE', ( #18880 ), #51586, .T. ) ;
#54423=AXIS2_PLACEMENT_3D ( 'NONE', #3128, #12990, #44980 ) ;
#54425=VECTOR ( 'NONE', #54477, 1000.000000000000114 ) ;
#54427=ORIENTED_EDGE ( 'NONE', *, *, #11096, .F. ) ;
#54431=CARTESIAN_POINT ( 'NONE',  ( -23.03840347525647658, 9.707315041312055470, 0.000000000000000000 ) ) ;
#54434=CARTESIAN_POINT ( 'NONE',  ( 1.667562369267789890, -64.99262834925670518, 170.0000000000000000 ) ) ;
#54436=ORIENTED_EDGE ( 'NONE', *, *, #20313, .T. ) ;
#54438=EDGE_CURVE ( 'NONE', #6453, #35701, #61776, .T. ) ;
#54439=DIRECTION ( 'NONE',  ( -1.156482317317871478E-16, -4.943042645790591857E-17, -1.000000000000000000 ) ) ;
#54457=CARTESIAN_POINT ( 'NONE',  ( 0.000000000000000000, 0.000000000000000000, 170.0000000000000000 ) ) ;
#54459=LINE ( 'NONE', #44264, #47542 ) ;
#54461=ADVANCED_FACE ( 'NONE', ( #46290 ), #2705, .T. ) ;
#54470=AXIS2_PLACEMENT_3D ( 'NONE', #22288, #38466, #45131 ) ;
#54472=VECTOR ( 'NONE', #15331, 1000.000000000000000 ) ;
#54477=DIRECTION ( 'NONE',  ( 0.9839295885986321100, -0.1785568947986229116, 0.000000000000000000 ) ) ;
#54478=CARTESIAN_POINT ( 'NONE',  ( 48.79594074893261535, 16.97828781540491505, 26.66469104408687585 ) ) ;
#54485=VECTOR ( 'NONE', #26600, 1000.000000000000000 ) ;
#54487=ORIENTED_EDGE ( 'NONE', *, *, #56523, .F. ) ;
#54492=CARTESIAN_POINT ( 'NONE',  ( 0.000000000000000000, 0.000000000000000000, 170.0000000000000000 ) ) ;
#54503=DIRECTION ( 'NONE',  ( -0.000000000000000000, -0.000000000000000000, -1.000000000000000000 ) ) ;
#54505=EDGE_CURVE ( 'NONE', #47103, #31912, #42055, .T. ) ;
#54509=ORIENTED_EDGE ( 'NONE', *, *, #8756, .F. ) ;
#54512=DIRECTION ( 'NONE',  ( 0.000000000000000000, 0.000000000000000000, -1.000000000000000000 ) ) ;
#54513=AXIS2_PLACEMENT_3D ( 'NONE', #5592, #10874, #27046 ) ;
#54514=ORIENTED_EDGE ( 'NONE', *, *, #34141, .T. ) ;
#54517=CARTESIAN_POINT ( 'NONE',  ( -72.29721455218883364, -19.95276341750119897, 0.000000000000000000 ) ) ;
#54522=LINE ( 'NONE', #6352, #66019 ) ;
#54525=ADVANCED_FACE ( 'NONE', ( #58913 ), #43075, .T. ) ;
#54529=CARTESIAN_POINT ( 'NONE',  ( -52.13778968636736977, -39.42540649522066332, 43.58025477438756212 ) ) ;
#54531=CARTESIAN_POINT ( 'NONE',  ( -58.33959211651037435, 29.48226216511319464, 43.58025477438756212 ) ) ;
#54533=EDGE_CURVE ( 'NONE', #5941, #16163, #52094, .T. ) ;
#54542=CARTESIAN_POINT ( 'NONE',  ( 75.00000000000000000, -1.250000000000021094, 170.0000000000000000 ) ) ;
#54560=ADVANCED_FACE ( 'NONE', ( #17036 ), #1568, .F. ) ;
#54574=VECTOR ( 'NONE', #55885, 999.9999999999998863 ) ;
#54576=EDGE_LOOP ( 'NONE', ( #17046, #43698, #23221, #36795, #43212, #55315, #5741, #37217, #13620 ) ) ;
#54578=AXIS2_PLACEMENT_3D ( 'NONE', #6927, #60394, #1649 ) ;
#54579=VECTOR ( 'NONE', #10656, 1000.000000000000000 ) ;
#54588=AXIS2_PLACEMENT_3D ( 'NONE', #66263, #16645, #1517 ) ;
#54596=DIRECTION ( 'NONE',  ( 0.000000000000000000, 0.000000000000000000, 1.000000000000000000 ) ) ;
#54600=ORIENTED_EDGE ( 'NONE', *, *, #45524, .T. ) ;
#54603=DIRECTION ( 'NONE',  ( 1.000000000000000000, 0.000000000000000000, 0.000000000000000000 ) ) ;
#54604=CARTESIAN_POINT ( 'NONE',  ( -63.00000000000000000, 0.000000000000000000, 170.0000000000000000 ) ) ;
#54607=ORIENTED_EDGE ( 'NONE', *, *, #47311, .T. ) ;
#54625=PLANE ( 'NONE',  #54588 ) ;
#54637=FACE_OUTER_BOUND ( 'NONE', #56300, .T. ) ;
#54638=CARTESIAN_POINT ( 'NONE',  ( 3.245026581591060388, 33.26789593292490110, 6.893342931642332694 ) ) ;
#54640=VECTOR ( 'NONE', #44009, 1000.000000000000000 ) ;
#54641=DIRECTION ( 'NONE',  ( -0.3090169943749446757, -0.9510565162951544194, 0.000000000000000000 ) ) ;
#54642=ORIENTED_EDGE ( 'NONE', *, *, #52551, .F. ) ;
#54645=CARTESIAN_POINT ( 'NONE',  ( 36.85262215550149278, -53.56030941157680303, 0.000000000000000000 ) ) ;
#54649=CARTESIAN_POINT ( 'NONE',  ( 26.69682282325795697, -59.27986298182186431, 43.58025477438756923 ) ) ;
#54651=EDGE_CURVE ( 'NONE', #60669, #61883, #67004, .T. ) ;
#54658=CARTESIAN_POINT ( 'NONE',  ( -16.43619359402630664, 18.99971924381106092, 0.000000000000000000 ) ) ;
#54670=DIRECTION ( 'NONE',  ( -1.000000000000000000, 0.000000000000000000, 0.000000000000000000 ) ) ;
#54674=VECTOR ( 'NONE', #19206, 1000.000000000000000 ) ;
#54675=DIRECTION ( 'NONE',  ( 0.000000000000000000, 0.000000000000000000, -1.000000000000000000 ) ) ;
#54676=CARTESIAN_POINT ( 'NONE',  ( -65.36598343705435354, 0.000000000000000000, 41.38025477438755928 ) ) ;
#54687=DIRECTION ( 'NONE',  ( -0.3930250316539148359, -0.9195277725514544587, 0.000000000000000000 ) ) ;
#54689=ORIENTED_EDGE ( 'NONE', *, *, #26575, .T. ) ;
#54694=CARTESIAN_POINT ( 'NONE',  ( 4.165045035620147829, 64.88046627338042072, 41.38025477438755928 ) ) ;
#54703=EDGE_CURVE ( 'NONE', #31208, #63543, #68948, .T. ) ;
#54706=CYLINDRICAL_SURFACE ( 'NONE', #14040, 65.00000000000000000 ) ;
#54713=CYLINDRICAL_SURFACE ( 'NONE', #14242, 65.36598343705435354 ) ;
#54714=CARTESIAN_POINT ( 'NONE',  ( 38.31361498191044035, 1.250000000000018652, 13.32819299319724493 ) ) ;
#54720=CARTESIAN_POINT ( 'NONE',  ( 0.000000000000000000, 0.000000000000000000, 40.00000000000003553 ) ) ;
#54724=AXIS2_PLACEMENT_3D ( 'NONE', #57968, #38585, #12821 ) ;
#54725=CARTESIAN_POINT ( 'NONE',  ( -29.47687737404459085, 68.96458294135867106, 0.000000000000000000 ) ) ;
#54733=CARTESIAN_POINT ( 'NONE',  ( 0.000000000000000000, 0.000000000000000000, 43.58025477438756212 ) ) ;
#54736=ORIENTED_EDGE ( 'NONE', *, *, #32310, .T. ) ;
#54737=DIRECTION ( 'NONE',  ( 0.000000000000000000, 0.000000000000000000, 1.000000000000000000 ) ) ;
#54744=CARTESIAN_POINT ( 'NONE',  ( 22.18075376363927020, -11.79626863379931656, 3.061616997868437868E-16 ) ) ;
#54745=CARTESIAN_POINT ( 'NONE',  ( 0.000000000000000000, 0.000000000000000000, 40.00000000000003553 ) ) ;
#54773=CARTESIAN_POINT ( 'NONE',  ( 0.000000000000000000, 0.000000000000000000, 43.58025477438756212 ) ) ;
#54777=AXIS2_PLACEMENT_3D ( 'NONE', #12134, #6847, #54319 ) ;
#54781=VECTOR ( 'NONE', #4620, 1000.000000000000227 ) ;
#54786=EDGE_LOOP ( 'NONE', ( #60479, #67946, #46968, #37106 ) ) ;
#54787=VECTOR ( 'NONE', #11997, 1000.000000000000227 ) ;
#54795=CARTESIAN_POINT ( 'NONE',  ( 35.54014968547473785, 66.04466488925542933, 43.58025477438756212 ) ) ;
#54812=DIRECTION ( 'NONE',  ( 1.000000000000000000, 0.000000000000000000, 0.000000000000000000 ) ) ;
#54827=FACE_OUTER_BOUND ( 'NONE', #11692, .T. ) ;
#54842=ORIENTED_EDGE ( 'NONE', *, *, #20313, .F. ) ;
#54843=CARTESIAN_POINT ( 'NONE',  ( -65.36598343705435354, 0.000000000000000000, 41.38025477438755928 ) ) ;
#54844=ORIENTED_EDGE ( 'NONE', *, *, #33829, .T. ) ;
#54846=DIRECTION ( 'NONE',  ( 1.000000000000000000, -1.421085471520200372E-14, 0.000000000000000000 ) ) ;
#54849=DIRECTION ( 'NONE',  ( 0.000000000000000000, 0.000000000000000000, 1.000000000000000000 ) ) ;
#54857=FACE_OUTER_BOUND ( 'NONE', #45089, .T. ) ;
#54861=CARTESIAN_POINT ( 'NONE',  ( -55.15976438495155776, 34.41253982194033512, 41.38025477438755928 ) ) ;
#54867=ORIENTED_EDGE ( 'NONE', *, *, #65296, .T. ) ;
#54870=CONICAL_SURFACE ( 'NONE', #39184, 65.00000000000000000, 0.7853981633974497223 ) ;
#54874=CARTESIAN_POINT ( 'NONE',  ( 2.112947028648761272, 24.91054906769654664, 0.000000000000000000 ) ) ;
#54875=AXIS2_PLACEMENT_3D ( 'NONE', #32331, #43901, #63986 ) ;
#54882=CARTESIAN_POINT ( 'NONE',  ( 0.000000000000000000, 100.0000000000000000, 0.000000000000000000 ) ) ;
#54892=FACE_OUTER_BOUND ( 'NONE', #19441, .T. ) ;
#54904=FACE_OUTER_BOUND ( 'NONE', #19576, .T. ) ;
#54913=CARTESIAN_POINT ( 'NONE',  ( -4.238248324054826099, 66.51046413633903853, 34.48241823979277143 ) ) ;
#54917=CARTESIAN_POINT ( 'NONE',  ( 55.65793654284683356, -50.28674377798225947, 43.58025477438756212 ) ) ;
#54918=FACE_OUTER_BOUND ( 'NONE', #58586, .T. ) ;
#54922=B_SPLINE_CURVE_WITH_KNOTS ( 'NONE', 3,
 ( #39422, #65468, #55244, #22547 ),
 .UNSPECIFIED., .F., .F.,
 ( 4, 4 ),
 ( 9.900409499066787224E-07, 0.05658314289920114010 ),
 .UNSPECIFIED. ) ;
#54927=AXIS2_PLACEMENT_3D ( 'NONE', #66834, #44297, #13354 ) ;
#54932=DIRECTION ( 'NONE',  ( 0.9362348706397417564, -0.3513748240813305279, 0.000000000000000000 ) ) ;
#54938=EDGE_CURVE ( 'NONE', #3736, #63617, #9422, .T. ) ;
#54941=DIRECTION ( 'NONE',  ( -0.000000000000000000, -0.000000000000000000, 1.000000000000000000 ) ) ;
#54943=CARTESIAN_POINT ( 'NONE',  ( -23.14886993799584047, 9.760512885996790899, 3.061616997868437868E-16 ) ) ;
#54949=DIRECTION ( 'NONE',  ( 1.000000000000000000, 0.000000000000000000, 0.000000000000000000 ) ) ;
#54950=VERTEX_POINT ( 'NONE', #28569 ) ;
#54953=CARTESIAN_POINT ( 'NONE',  ( -47.92160639629907593, -33.27200008537087683, 27.58472315868179692 ) ) ;
#54959=AXIS2_PLACEMENT_3D ( 'NONE', #2399, #66086, #44247 ) ;
#54962=EDGE_CURVE ( 'NONE', #21605, #35550, #55291, .T. ) ;
#54970=DIRECTION ( 'NONE',  ( -1.000000000000000000, 0.000000000000000000, 0.000000000000000000 ) ) ;
#54973=LINE ( 'NONE', #28242, #6285 ) ;
#54974=VERTEX_POINT ( 'NONE', #67267 ) ;
#54975=VERTEX_POINT ( 'NONE', #2881 ) ;
#54983=DIRECTION ( 'NONE',  ( -0.000000000000000000, 0.000000000000000000, -1.000000000000000000 ) ) ;
#54987=DIRECTION ( 'NONE',  ( 0.2225209339563042066, 0.9749279121818259508, 0.000000000000000000 ) ) ;
#54989=ORIENTED_EDGE ( 'NONE', *, *, #61876, .F. ) ;
#54990=CARTESIAN_POINT ( 'NONE',  ( -24.40147488398704567, -5.437648709335880071, 0.000000000000000000 ) ) ;
#54999=ORIENTED_EDGE ( 'NONE', *, *, #40419, .T. ) ;
#55001=LINE ( 'NONE', #39534, #29357 ) ;
#55002=CARTESIAN_POINT ( 'NONE',  ( 0.000000000000000000, 0.000000000000000000, 0.000000000000000000 ) ) ;
#55018=EDGE_CURVE ( 'NONE', #8019, #23880, #45366, .T. ) ;
#55019=DIRECTION ( 'NONE',  ( -0.9195277725514544587, 0.3930250316539147803, 0.000000000000000000 ) ) ;
#55021=EDGE_CURVE ( 'NONE', #15204, #26008, #19053, .T. ) ;
#55022=EDGE_CURVE ( 'NONE', #39395, #51882, #34205, .T. ) ;
#55023=EDGE_LOOP ( 'NONE', ( #12911, #6031, #3765, #2567 ) ) ;
#55028=VECTOR ( 'NONE', #21897, 1000.000000000000000 ) ;
#55044=EDGE_CURVE ( 'NONE', #46155, #20027, #23645, .T. ) ;
#55051=ORIENTED_EDGE ( 'NONE', *, *, #51372, .F. ) ;
#55055=LINE ( 'NONE', #6874, #27525 ) ;
#55057=ORIENTED_EDGE ( 'NONE', *, *, #6049, .T. ) ;
#55059=AXIS2_PLACEMENT_3D ( 'NONE', #69446, #21261, #5432 ) ;
#55060=ORIENTED_EDGE ( 'NONE', *, *, #59061, .T. ) ;
#55063=LINE ( 'NONE', #24469, #51184 ) ;
#55066=CARTESIAN_POINT ( 'NONE',  ( -21.27554331372999741, 61.43430442924864820, 170.0000000000000000 ) ) ;
#55076=VECTOR ( 'NONE', #50131, 1000.000000000000000 ) ;
#55091=PLANE ( 'NONE',  #19949 ) ;
#55092=VECTOR ( 'NONE', #67470, 1000.000000000000114 ) ;
#55097=ORIENTED_EDGE ( 'NONE', *, *, #37465, .F. ) ;
#55099=CARTESIAN_POINT ( 'NONE',  ( 13.24564585880136036, -63.65041531508826012, 170.0000000000000000 ) ) ;
#55103=DIRECTION ( 'NONE',  ( 0.6579387259397136978, -0.7530714660036099684, 0.000000000000000000 ) ) ;
#55110=VECTOR ( 'NONE', #5939, 1000.000000000000000 ) ;
#55116=VERTEX_POINT ( 'NONE', #6332 ) ;
#55129=EDGE_CURVE ( 'NONE', #27252, #33243, #47602, .T. ) ;
#55139=DIRECTION ( 'NONE',  ( 0.04486483035051862939, -0.9989930665413143673, 0.000000000000000000 ) ) ;
#55142=CIRCLE ( 'NONE', #36084, 65.00000000000000000 ) ;
#55150=VERTEX_POINT ( 'NONE', #714 ) ;
#55164=ORIENTED_EDGE ( 'NONE', *, *, #63938, .T. ) ;
#55166=EDGE_LOOP ( 'NONE', ( #43284, #56325, #12639, #47173 ) ) ;
#55167=LINE ( 'NONE', #28088, #18400 ) ;
#55183=DIRECTION ( 'NONE',  ( 0.9909497617679352555, -0.1342332658176522420, 0.000000000000000000 ) ) ;
#55184=DIRECTION ( 'NONE',  ( -1.000000000000000000, 0.000000000000000000, 0.000000000000000000 ) ) ;
#55195=CARTESIAN_POINT ( 'NONE',  ( -51.84164840787185113, 39.21024726209461875, 40.00000000000003553 ) ) ;
#55204=AXIS2_PLACEMENT_3D ( 'NONE', #20046, #36569, #31296 ) ;
#55207=ORIENTED_EDGE ( 'NONE', *, *, #42701, .F. ) ;
#55213=CARTESIAN_POINT ( 'NONE',  ( -61.41100614348627573, -43.07262267896732766, 170.0000000000000000 ) ) ;
#55216=CONICAL_SURFACE ( 'NONE', #6917, 74.95140232871122521, 0.8777644062502172329 ) ;
#55221=CARTESIAN_POINT ( 'NONE',  ( -29.87147652227455552, 100.0000000000000000, 133.5802547743875550 ) ) ;
#55234=ORIENTED_EDGE ( 'NONE', *, *, #26747, .F. ) ;
#55238=VECTOR ( 'NONE', #35232, 1000.000000000000114 ) ;
#55244=CARTESIAN_POINT ( 'NONE',  ( 32.24915246298996863, 20.72408643103235448, 13.32819299319724493 ) ) ;
#55246=DIRECTION ( 'NONE',  ( -0.000000000000000000, -0.000000000000000000, -1.000000000000000000 ) ) ;
#55255=VERTEX_POINT ( 'NONE', #55213 ) ;
#55263=DIRECTION ( 'NONE',  ( 0.000000000000000000, 0.000000000000000000, 1.000000000000000000 ) ) ;
#55264=ADVANCED_FACE ( 'NONE', ( #64373 ), #59092, .T. ) ;
#55265=CARTESIAN_POINT ( 'NONE',  ( -44.26023579658871654, -48.10138582123836670, 43.58025477438756212 ) ) ;
#55271=ORIENTED_EDGE ( 'NONE', *, *, #46142, .T. ) ;
#55274=FACE_OUTER_BOUND ( 'NONE', #29830, .T. ) ;
#55277=EDGE_CURVE ( 'NONE', #54950, #43248, #40428, .T. ) ;
#55279=ORIENTED_EDGE ( 'NONE', *, *, #58368, .F. ) ;
#55284=LINE ( 'NONE', #65505, #510 ) ;
#55288=CARTESIAN_POINT ( 'NONE',  ( 11.30618213853385967, 74.15344055032308290, 73.58025477438755502 ) ) ;
#55291=LINE ( 'NONE', #5711, #29650 ) ;
#55293=CARTESIAN_POINT ( 'NONE',  ( -49.77357484059193382, 41.82599373102802787, 43.58025477438756923 ) ) ;
#55304=CARTESIAN_POINT ( 'NONE',  ( -61.29635759142584561, -21.66977272663583776, 170.0000000000000000 ) ) ;
#55309=EDGE_LOOP ( 'NONE', ( #34848, #16786, #69359, #42171 ) ) ;
#55315=ORIENTED_EDGE ( 'NONE', *, *, #43559, .F. ) ;
#55330=EDGE_CURVE ( 'NONE', #12323, #8257, #28549, .T. ) ;
#55332=EDGE_CURVE ( 'NONE', #50410, #57368, #1765, .T. ) ;
#55343=ADVANCED_FACE ( 'NONE', ( #17938 ), #39391, .T. ) ;
#55348=CARTESIAN_POINT ( 'NONE',  ( -25.10237775011640338, 1.004202417053489116, 3.061616997868437868E-16 ) ) ;
#55350=ORIENTED_EDGE ( 'NONE', *, *, #2155, .T. ) ;
#55351=VERTEX_POINT ( 'NONE', #45004 ) ;
#55352=VECTOR ( 'NONE', #24154, 1000.000000000000227 ) ;
#55353=CARTESIAN_POINT ( 'NONE',  ( -7.486743542470047252, 64.58150799671128084, 43.58025477438756923 ) ) ;
#55359=AXIS2_PLACEMENT_3D ( 'NONE', #23438, #60357, #12178 ) ;
#55361=ADVANCED_FACE ( 'NONE', ( #21989 ), #32547, .T. ) ;
#55364=VERTEX_POINT ( 'NONE', #63273 ) ;
#55370=DIRECTION ( 'NONE',  ( -0.000000000000000000, -0.000000000000000000, -1.000000000000000000 ) ) ;
#55372=DIRECTION ( 'NONE',  ( -1.000000000000000000, 0.000000000000000000, 0.000000000000000000 ) ) ;
#55373=ORIENTED_EDGE ( 'NONE', *, *, #58825, .T. ) ;
#55388=DIRECTION ( 'NONE',  ( -0.000000000000000000, -0.000000000000000000, -1.000000000000000000 ) ) ;
#55394=CIRCLE ( 'NONE', #35166, 24.99999999999985434 ) ;
#55398=VERTEX_POINT ( 'NONE', #62929 ) ;
#55400=LINE ( 'NONE', #13205, #49144 ) ;
#55416=EDGE_CURVE ( 'NONE', #37187, #48528, #17770, .T. ) ;
#55418=CARTESIAN_POINT ( 'NONE',  ( 0.000000000000000000, 0.000000000000000000, 43.58025477438756212 ) ) ;
#55419=DIRECTION ( 'NONE',  ( -1.000000000000000000, 0.000000000000000000, 0.000000000000000000 ) ) ;
#55429=CARTESIAN_POINT ( 'NONE',  ( 10.78925482157233340, 22.68765681156020264, 3.061616997868437868E-16 ) ) ;
#55435=DIRECTION ( 'NONE',  ( 0.000000000000000000, 0.000000000000000000, 1.000000000000000000 ) ) ;
#55455=FACE_OUTER_BOUND ( 'NONE', #27794, .T. ) ;
#55460=ORIENTED_EDGE ( 'NONE', *, *, #4456, .T. ) ;
#55462=VECTOR ( 'NONE', #11306, 1000.000000000000000 ) ;
#55473=SHAPE_REPRESENTATION ( 'y3+', ( #66832 ), #2840 ) ;
#55483=ORIENTED_EDGE ( 'NONE', *, *, #38118, .T. ) ;
#55499=LINE ( 'NONE', #22799, #63431 ) ;
#55503=ADVANCED_FACE ( 'NONE', ( #24444 ), #51516, .T. ) ;
#55506=EDGE_CURVE ( 'NONE', #53998, #27278, #13193, .T. ) ;
#55521=CYLINDRICAL_SURFACE ( 'NONE', #20589, 65.00000000000000000 ) ;
#55532=VERTEX_POINT ( 'NONE', #8947 ) ;
#55549=VECTOR ( 'NONE', #43590, 1000.000000000000114 ) ;
#55551=LINE ( 'NONE', #65781, #43091 ) ;
#55564=CARTESIAN_POINT ( 'NONE',  ( 60.82895951008336510, 30.68107831874607072, 170.0000000000000000 ) ) ;
#55567=B_SPLINE_CURVE_WITH_KNOTS ( 'NONE', 3,
 ( #10171, #6274, #5580, #42530, #27033, #54093 ),
 .UNSPECIFIED., .F., .F.,
 ( 4, 2, 4 ),
 ( 1.095770181117380865E-06, 0.03239442681617711595, 0.06478775786217311206 ),
 .UNSPECIFIED. ) ;
#55568=ADVANCED_FACE ( 'NONE', ( #62409, #30063 ), #2628, .F. ) ;
#55569=ORIENTED_EDGE ( 'NONE', *, *, #38589, .T. ) ;
#55573=ADVANCED_FACE ( 'NONE', ( #14564 ), #68383, .T. ) ;
#55576=LINE ( 'NONE', #54161, #12830 ) ;
#55591=DIRECTION ( 'NONE',  ( -0.000000000000000000, -0.000000000000000000, 1.000000000000000000 ) ) ;
#55594=AXIS2_PLACEMENT_3D ( 'NONE', #36061, #3018, #40989 ) ;
#55597=CIRCLE ( 'NONE', #37768, 65.36598343705435354 ) ;
#55615=DIRECTION ( 'NONE',  ( 1.000000000000000000, 0.000000000000000000, 0.000000000000000000 ) ) ;
#55619=CARTESIAN_POINT ( 'NONE',  ( -2.374459999240554620, 25.00999262126967437, 3.061616997868437868E-16 ) ) ;
#55620=VERTEX_POINT ( 'NONE', #13534 ) ;
#55621=ORIENTED_EDGE ( 'NONE', *, *, #48949, .T. ) ;
#55623=CARTESIAN_POINT ( 'NONE',  ( -16.04603980063842883, -64.68484481756375715, 34.48241795236666007 ) ) ;
#55639=DIRECTION ( 'NONE',  ( -0.000000000000000000, -0.000000000000000000, -1.000000000000000000 ) ) ;
#55655=EDGE_LOOP ( 'NONE', ( #67523, #43040, #65939, #43743 ) ) ;
#55669=ORIENTED_EDGE ( 'NONE', *, *, #61052, .F. ) ;
#55674=EDGE_CURVE ( 'NONE', #49213, #68160, #9285, .T. ) ;
#55681=ORIENTED_EDGE ( 'NONE', *, *, #13430, .T. ) ;
#55685=CARTESIAN_POINT ( 'NONE',  ( 0.000000000000000000, 0.000000000000000000, 40.00000000000003553 ) ) ;
#55689=CARTESIAN_POINT ( 'NONE',  ( -65.36598343705435354, 0.000000000000000000, 41.38025477438755928 ) ) ;
#55714=CARTESIAN_POINT ( 'NONE',  ( -14.27739063142107589, 30.22315691998191056, 6.893342933292202268 ) ) ;
#55720=ORIENTED_EDGE ( 'NONE', *, *, #21156, .F. ) ;
#55730=DIRECTION ( 'NONE',  ( -1.000000000000000000, 0.000000000000000000, 0.000000000000000000 ) ) ;
#55734=ORIENTED_EDGE ( 'NONE', *, *, #40356, .F. ) ;
#55737=CARTESIAN_POINT ( 'NONE',  ( -64.97888516016278970, 7.103257987405393159, 41.38025477438755928 ) ) ;
#55738=CARTESIAN_POINT ( 'NONE',  ( 26.69682282325795697, -59.27986298182186431, 0.000000000000000000 ) ) ;
#55740=EDGE_LOOP ( 'NONE', ( #54514, #61222, #14311, #58412 ) ) ;
#55742=DIRECTION ( 'NONE',  ( 1.000000000000000000, 0.000000000000000000, 0.000000000000000000 ) ) ;
#55745=CIRCLE ( 'NONE', #27659, 65.00000000000000000 ) ;
#55755=ADVANCED_FACE ( 'NONE', ( #37738 ), #451, .T. ) ;
#55757=VECTOR ( 'NONE', #39644, 1000.000000000000227 ) ;
#55770=ORIENTED_EDGE ( 'NONE', *, *, #56278, .F. ) ;
#55773=EDGE_CURVE ( 'NONE', #61844, #51807, #26338, .T. ) ;
#55774=EDGE_LOOP ( 'NONE', ( #31884, #33610, #39430, #15820 ) ) ;
#55776=LINE ( 'NONE', #62077, #46961 ) ;
#55779=CARTESIAN_POINT ( 'NONE',  ( 57.25833571151937207, -48.36523237396138342, 41.38025477438755928 ) ) ;
#55783=DIRECTION ( 'NONE',  ( -0.000000000000000000, -0.000000000000000000, -1.000000000000000000 ) ) ;
#55784=ORIENTED_EDGE ( 'NONE', *, *, #35419, .T. ) ;
#55785=ORIENTED_EDGE ( 'NONE', *, *, #40753, .F. ) ;
#55789=DIRECTION ( 'NONE',  ( 0.7530714660036099684, 0.6579387259397136978, 0.000000000000000000 ) ) ;
#55790=CARTESIAN_POINT ( 'NONE',  ( 30.47484983475695586, 59.26962220273969706, 34.48241823991043020 ) ) ;
#55803=CARTESIAN_POINT ( 'NONE',  ( -33.37998494234739155, 1.749200548590775117, 6.893342931535256568 ) ) ;
#55807=VECTOR ( 'NONE', #31235, 1000.000000000000000 ) ;
#55809=LINE ( 'NONE', #67078, #66381 ) ;
#55810=CARTESIAN_POINT ( 'NONE',  ( 44.98017955506416854, 25.41829140422818156, 26.66469104408689006 ) ) ;
#55825=DIRECTION ( 'NONE',  ( 0.8584487936018728726, -0.5128992774058949156, 0.000000000000000000 ) ) ;
#55829=ORIENTED_EDGE ( 'NONE', *, *, #31364, .T. ) ;
#55831=EDGE_CURVE ( 'NONE', #33798, #19006, #44243, .T. ) ;
#55834=EDGE_CURVE ( 'NONE', #32488, #33166, #34215, .T. ) ;
#55837=EDGE_LOOP ( 'NONE', ( #21041, #59965, #61168, #57312 ) ) ;
#55847=EDGE_LOOP ( 'NONE', ( #19188, #40874, #17057, #27804 ) ) ;
#55850=EDGE_CURVE ( 'NONE', #64355, #49951, #39479, .T. ) ;
#55852=CIRCLE ( 'NONE', #59185, 25.12245591505646303 ) ;
#55858=EDGE_CURVE ( 'NONE', #6300, #28769, #44046, .T. ) ;
#55860=AXIS2_PLACEMENT_3D ( 'NONE', #51948, #12946, #3762 ) ;
#55862=VECTOR ( 'NONE', #67565, 999.9999999999998863 ) ;
#55864=AXIS2_PLACEMENT_3D ( 'NONE', #5747, #15966, #48994 ) ;
#55870=VERTEX_POINT ( 'NONE', #17322 ) ;
#55871=ORIENTED_EDGE ( 'NONE', *, *, #50276, .F. ) ;
#55872=CARTESIAN_POINT ( 'NONE',  ( -63.58578643762691485, 7.787012983210697559E-15, 41.41421356237313489 ) ) ;
#55873=FACE_OUTER_BOUND ( 'NONE', #22456, .T. ) ;
#55877=DIRECTION ( 'NONE',  ( -0.9009688679024155933, -0.4338837391175656699, 0.000000000000000000 ) ) ;
#55885=DIRECTION ( 'NONE',  ( 0.9362348706397369824, 0.3513748240813435175, 0.000000000000000000 ) ) ;
#55888=DIRECTION ( 'NONE',  ( 0.000000000000000000, 0.000000000000000000, -1.000000000000000000 ) ) ;
#55893=ORIENTED_EDGE ( 'NONE', *, *, #27843, .F. ) ;
#55894=CARTESIAN_POINT ( 'NONE',  ( -30.62628708973388569, 68.47330165179126027, 170.0000000000000000 ) ) ;
#55897=ORIENTED_EDGE ( 'NONE', *, *, #16653, .F. ) ;
#55898=CARTESIAN_POINT ( 'NONE',  ( 24.34427655538957680, -5.688250960945929080, 0.000000000000000000 ) ) ;
#55914=AXIS2_PLACEMENT_3D ( 'NONE', #54166, #38357, #5989 ) ;
#55923=CARTESIAN_POINT ( 'NONE',  ( 0.000000000000000000, 0.000000000000000000, 40.00000000000003553 ) ) ;
#55926=DIRECTION ( 'NONE',  ( -0.000000000000000000, -0.000000000000000000, 1.000000000000000000 ) ) ;
#55933=ORIENTED_EDGE ( 'NONE', *, *, #69325, .F. ) ;
#55935=DIRECTION ( 'NONE',  ( 1.000000000000000000, 0.000000000000000000, 0.000000000000000000 ) ) ;
#55937=ADVANCED_FACE ( 'NONE', ( #65172 ), #33862, .T. ) ;
#55942=CARTESIAN_POINT ( 'NONE',  ( -39.09764951710990744, -70.01774562958885895, 73.58025477438756923 ) ) ;
#55958=CARTESIAN_POINT ( 'NONE',  ( -2.113472939310175658, 74.92159864268209901, 41.38025477438755928 ) ) ;
#55961=CARTESIAN_POINT ( 'NONE',  ( -22.06416059020174103, -12.01293505575318044, 3.061616997868437868E-16 ) ) ;
#55965=DIRECTION ( 'NONE',  ( -0.000000000000000000, -0.000000000000000000, -1.000000000000000000 ) ) ;
#55973=CARTESIAN_POINT ( 'NONE',  ( -25.87147652227456263, 70.00000000000000000, 77.58025477438755502 ) ) ;
#55976=CARTESIAN_POINT ( 'NONE',  ( -34.75846525698938194, -54.92585086258257121, 170.0000000000000000 ) ) ;
#55978=LINE ( 'NONE', #25012, #30773 ) ;
#55986=EDGE_CURVE ( 'NONE', #45254, #59777, #2547, .T. ) ;
#55993=FACE_OUTER_BOUND ( 'NONE', #11420, .T. ) ;
#56013=EDGE_LOOP ( 'NONE', ( #52458, #30820, #51315, #36192 ) ) ;
#56020=VERTEX_POINT ( 'NONE', #49198 ) ;
#56024=ORIENTED_EDGE ( 'NONE', *, *, #21156, .T. ) ;
#56025=EDGE_CURVE ( 'NONE', #49164, #24416, #7007, .T. ) ;
#56028=CARTESIAN_POINT ( 'NONE',  ( 0.000000000000000000, 0.000000000000000000, 170.0000000000000000 ) ) ;
#56038=DIRECTION ( 'NONE',  ( -0.000000000000000000, -0.000000000000000000, 1.000000000000000000 ) ) ;
#56039=DIRECTION ( 'NONE',  ( -1.000000000000000000, 0.000000000000000000, 0.000000000000000000 ) ) ;
#56042=CARTESIAN_POINT ( 'NONE',  ( -4.164416015344991173, -64.86646004871191451, 40.00000000000003553 ) ) ;
#56044=VERTEX_POINT ( 'NONE', #28460 ) ;
#56052=EDGE_CURVE ( 'NONE', #7827, #37858, #44277, .T. ) ;
#56054=ADVANCED_FACE ( 'NONE', ( #33748 ), #52192, .T. ) ;
#56056=FACE_OUTER_BOUND ( 'NONE', #27363, .T. ) ;
#56058=ORIENTED_EDGE ( 'NONE', *, *, #59329, .F. ) ;
#56060=EDGE_CURVE ( 'NONE', #57871, #5356, #34099, .T. ) ;
#56062=CARTESIAN_POINT ( 'NONE',  ( -33.15588667008874779, -4.239136283579393982, 6.893342931535249463 ) ) ;
#56064=EDGE_CURVE ( 'NONE', #35550, #56478, #65762, .T. ) ;
#56070=CARTESIAN_POINT ( 'NONE',  ( 45.78444578632068840, -59.41672343742509810, 170.0000000000000000 ) ) ;
#56087=DIRECTION ( 'NONE',  ( -0.000000000000000000, -0.000000000000000000, -1.000000000000000000 ) ) ;
#56090=PLANE ( 'NONE',  #46159 ) ;
#56091=VERTEX_POINT ( 'NONE', #22836 ) ;
#56095=CARTESIAN_POINT ( 'NONE',  ( -55.15976438495157197, 34.41253982194030669, 170.0000000000000000 ) ) ;
#56101=DIRECTION ( 'NONE',  ( 0.5508969814520944253, 0.8345732537213078617, 0.000000000000000000 ) ) ;
#56111=ORIENTED_EDGE ( 'NONE', *, *, #716, .F. ) ;
#56120=CARTESIAN_POINT ( 'NONE',  ( -15.47041015649658213, 73.39774458108210808, 43.58025477438756212 ) ) ;
#56123=ORIENTED_EDGE ( 'NONE', *, *, #56214, .T. ) ;
#56128=CARTESIAN_POINT ( 'NONE',  ( -30.60309003827877916, -68.41902945196855512, 41.38025477438755928 ) ) ;
#56129=DIRECTION ( 'NONE',  ( -0.6910626489868685329, 0.7227948638273878901, 0.000000000000000000 ) ) ;
#56134=VERTEX_POINT ( 'NONE', #38310 ) ;
#56135=ORIENTED_EDGE ( 'NONE', *, *, #2875, .F. ) ;
#56136=EDGE_CURVE ( 'NONE', #67695, #68560, #49547, .T. ) ;
#56165=LINE ( 'NONE', #17845, #55757 ) ;
#56180=ORIENTED_EDGE ( 'NONE', *, *, #36509, .F. ) ;
#56190=AXIS2_PLACEMENT_3D ( 'NONE', #35072, #68468, #67440 ) ;
#56193=EDGE_CURVE ( 'NONE', #69067, #2052, #16851, .T. ) ;
#56200=ORIENTED_EDGE ( 'NONE', *, *, #28250, .F. ) ;
#56203=VECTOR ( 'NONE', #52581, 1000.000000000000000 ) ;
#56208=PLANE ( 'NONE',  #10081 ) ;
#56209=EDGE_CURVE ( 'NONE', #56892, #66979, #14318, .T. ) ;
#56210=CARTESIAN_POINT ( 'NONE',  ( 22.93737758745385946, -9.943676855698914352, 0.000000000000000000 ) ) ;
#56212=VERTEX_POINT ( 'NONE', #46662 ) ;
#56214=EDGE_CURVE ( 'NONE', #59078, #25903, #13963, .T. ) ;
#56218=ORIENTED_EDGE ( 'NONE', *, *, #49262, .T. ) ;
#56219=DIRECTION ( 'NONE',  ( 1.000000000000000000, 0.000000000000000000, 0.000000000000000000 ) ) ;
#56234=VERTEX_POINT ( 'NONE', #18901 ) ;
#56235=CARTESIAN_POINT ( 'NONE',  ( -59.09450113343203270, -27.07101652673575032, 170.0000000000000000 ) ) ;
#56244=EDGE_CURVE ( 'NONE', #29654, #37239, #15141, .T. ) ;
#56250=CARTESIAN_POINT ( 'NONE',  ( 0.000000000000000000, 0.000000000000000000, 41.38025477438755928 ) ) ;
#56255=DIRECTION ( 'NONE',  ( -1.000000000000000000, 0.000000000000000000, 0.000000000000000000 ) ) ;
#56260=VECTOR ( 'NONE', #47840, 1000.000000000000000 ) ;
#56270=DIRECTION ( 'NONE',  ( -0.000000000000000000, -0.000000000000000000, -1.000000000000000000 ) ) ;
#56273=DIRECTION ( 'NONE',  ( -0.3930250316539148359, -0.9195277725514544587, 0.000000000000000000 ) ) ;
#56274=ORIENTED_EDGE ( 'NONE', *, *, #57470, .F. ) ;
#56275=EDGE_CURVE ( 'NONE', #43209, #11718, #62853, .T. ) ;
#56278=EDGE_CURVE ( 'NONE', #7321, #38915, #12895, .T. ) ;
#56293=DIRECTION ( 'NONE',  ( 2.312964634635743450E-16, -0.000000000000000000, 1.000000000000000000 ) ) ;
#56300=EDGE_LOOP ( 'NONE', ( #61490, #63185, #53286, #53851 ) ) ;
#56301=LINE ( 'NONE', #51033, #18353 ) ;
#56306=CARTESIAN_POINT ( 'NONE',  ( 61.62594073580542897, 21.79346734965000820, 43.58025477438756212 ) ) ;
#56307=DIRECTION ( 'NONE',  ( -1.000000000000000000, 0.000000000000000000, 0.000000000000000000 ) ) ;
#56308=CARTESIAN_POINT ( 'NONE',  ( 54.16778967912048159, -21.66464655980577803, 27.58472315868180402 ) ) ;
#56309=CIRCLE ( 'NONE', #64176, 65.00000000000000000 ) ;
#56311=CIRCLE ( 'NONE', #12528, 65.00000000000000000 ) ;
#56317=DIRECTION ( 'NONE',  ( -1.000000000000000000, 0.000000000000000000, 0.000000000000000000 ) ) ;
#56321=DIRECTION ( 'NONE',  ( 0.000000000000000000, 0.000000000000000000, 1.000000000000000000 ) ) ;
#56323=CONICAL_SURFACE ( 'NONE', #65315, 74.95140232871122521, 0.8777644062502172329 ) ;
#56325=ORIENTED_EDGE ( 'NONE', *, *, #35751, .F. ) ;
#56326=EDGE_CURVE ( 'NONE', #17465, #11802, #9520, .T. ) ;
#56327=EDGE_CURVE ( 'NONE', #62331, #24824, #40687, .T. ) ;
#56333=EDGE_CURVE ( 'NONE', #4891, #53557, #57573, .T. ) ;
#56335=ORIENTED_EDGE ( 'NONE', *, *, #67051, .F. ) ;
#56336=DIRECTION ( 'NONE',  ( -0.000000000000000000, -0.000000000000000000, 1.000000000000000000 ) ) ;
#56357=VECTOR ( 'NONE', #69489, 999.9999999999998863 ) ;
#56358=ORIENTED_EDGE ( 'NONE', *, *, #41309, .T. ) ;
#56360=CARTESIAN_POINT ( 'NONE',  ( 0.000000000000000000, 0.000000000000000000, 0.000000000000000000 ) ) ;
#56362=DIRECTION ( 'NONE',  ( -1.000000000000000000, 0.000000000000000000, 0.000000000000000000 ) ) ;
#56367=ORIENTED_EDGE ( 'NONE', *, *, #53745, .T. ) ;
#56372=CARTESIAN_POINT ( 'NONE',  ( -15.45727656667583005, -73.34020256436187424, 41.38025477438755928 ) ) ;
#56385=EDGE_CURVE ( 'NONE', #37545, #65974, #48792, .T. ) ;
#56393=EDGE_CURVE ( 'NONE', #67708, #26725, #10067, .T. ) ;
#56414=FACE_OUTER_BOUND ( 'NONE', #38051, .T. ) ;
#56417=VECTOR ( 'NONE', #34075, 1000.000000000000000 ) ;
#56419=ORIENTED_EDGE ( 'NONE', *, *, #46306, .T. ) ;
#56424=CARTESIAN_POINT ( 'NONE',  ( 61.91366885787816443, -28.42865614898931881, 0.000000000000000000 ) ) ;
#56428=DIRECTION ( 'NONE',  ( 0.9195277725514489076, 0.3930250316539278810, 5.102127870520022769E-18 ) ) ;
#56433=DIRECTION ( 'NONE',  ( -0.000000000000000000, -0.000000000000000000, -1.000000000000000000 ) ) ;
#56435=CARTESIAN_POINT ( 'NONE',  ( 2.051824250824025420, -73.54888393769144272, 133.5802547743875550 ) ) ;
#56446=EDGE_CURVE ( 'NONE', #925, #10198, #68797, .T. ) ;
#56466=ORIENTED_EDGE ( 'NONE', *, *, #61076, .T. ) ;
#56467=ADVANCED_FACE ( 'NONE', ( #20969 ), #64216, .F. ) ;
#56478=VERTEX_POINT ( 'NONE', #42421 ) ;
#56480=ORIENTED_EDGE ( 'NONE', *, *, #45610, .F. ) ;
#56491=ORIENTED_EDGE ( 'NONE', *, *, #56193, .T. ) ;
#56492=CARTESIAN_POINT ( 'NONE',  ( 33.08880980852370612, -4.734317562933250123, 6.893342931793783102 ) ) ;
#56505=LINE ( 'NONE', #7290, #56870 ) ;
#56511=VECTOR ( 'NONE', #55825, 1000.000000000000227 ) ;
#56514=VECTOR ( 'NONE', #4261, 1000.000000000000000 ) ;
#56518=CARTESIAN_POINT ( 'NONE',  ( 33.53140065650502066, -18.57796444702716343, 13.32819299319723072 ) ) ;
#56521=AXIS2_PLACEMENT_3D ( 'NONE', #68828, #43481, #15725 ) ;
#56523=EDGE_CURVE ( 'NONE', #59923, #58815, #69490, .T. ) ;
#56525=DIRECTION ( 'NONE',  ( 1.000000000000000000, 0.000000000000000000, 0.000000000000000000 ) ) ;
#56532=EDGE_CURVE ( 'NONE', #64743, #39418, #42756, .T. ) ;
#56540=ORIENTED_EDGE ( 'NONE', *, *, #21450, .F. ) ;
#56562=AXIS2_PLACEMENT_3D ( 'NONE', #15672, #172, #42403 ) ;
#56566=B_SPLINE_CURVE_WITH_KNOTS ( 'NONE', 3,
 ( #20511, #19835, #30048, #4004, #41292, #58155 ),
 .UNSPECIFIED., .F., .F.,
 ( 4, 2, 4 ),
 ( 0.03218932480516803474, 0.06469831007220622210, 0.09720729533924440946 ),
 .UNSPECIFIED. ) ;
#56569=ORIENTED_EDGE ( 'NONE', *, *, #11015, .F. ) ;
#56583=FACE_OUTER_BOUND ( 'NONE', #21922, .T. ) ;
#56599=SURFACE_SIDE_STYLE ('',( #56958 ) ) ;
#56608=DIRECTION ( 'NONE',  ( 0.04486483035051862939, -0.9989930665413143673, 0.000000000000000000 ) ) ;
#56609=AXIS2_PLACEMENT_3D ( 'NONE', #22229, #27851, #22577 ) ;
#56613=AXIS2_PLACEMENT_3D ( 'NONE', #12755, #32813, #54603 ) ;
#56616=DIRECTION ( 'NONE',  ( -0.000000000000000000, -0.000000000000000000, -1.000000000000000000 ) ) ;
#56618=VECTOR ( 'NONE', #17855, 1000.000000000000000 ) ;
#56623=CARTESIAN_POINT ( 'NONE',  ( 64.98797965777978902, 1.250000000000011990, 40.00000000000003553 ) ) ;
#56633=EDGE_CURVE ( 'NONE', #31912, #63750, #45197, .T. ) ;
#56637=ORIENTED_EDGE ( 'NONE', *, *, #59414, .T. ) ;
#56641=CARTESIAN_POINT ( 'NONE',  ( 17.14961137969540772, -48.73599164036525622, 26.66469066592269499 ) ) ;
#56643=B_SPLINE_CURVE_WITH_KNOTS ( 'NONE', 3,
 ( #29049, #50489, #18482, #2652 ),
 .UNSPECIFIED., .F., .F.,
 ( 4, 4 ),
 ( 9.900409499053008115E-07, 0.05658314289920116785 ),
 .UNSPECIFIED. ) ;
#56651=VECTOR ( 'NONE', #33363, 1000.000000000000114 ) ;
#56662=AXIS2_PLACEMENT_3D ( 'NONE', #65233, #27242, #48675 ) ;
#56664=CARTESIAN_POINT ( 'NONE',  ( -51.84164840787185113, 39.21024726209461875, 170.0000000000000000 ) ) ;
#56665=VERTEX_POINT ( 'NONE', #19858 ) ;
#56671=CARTESIAN_POINT ( 'NONE',  ( 13.02837909493185720, 36.05214288467553985, 13.32819397642332326 ) ) ;
#56673=CONICAL_SURFACE ( 'NONE', #52197, 65.00000000000000000, 0.7853981633974497223 ) ;
#56675=FACE_OUTER_BOUND ( 'NONE', #65646, .T. ) ;
#56677=CARTESIAN_POINT ( 'NONE',  ( -24.75616454008743972, 3.483147608716851806, 0.000000000000000000 ) ) ;
#56689=CARTESIAN_POINT ( 'NONE',  ( -1.683356153843273750, 65.34430428700410687, 6.377659838150135158E-18 ) ) ;
#56690=CARTESIAN_POINT ( 'NONE',  ( 36.44731223145974752, 20.32014051031833191, 13.79046340968177908 ) ) ;
#56698=ADVANCED_FACE ( 'NONE', ( #15612 ), #53219, .F. ) ;
#56701=VECTOR ( 'NONE', #37157, 1000.000000000000000 ) ;
#56706=EDGE_CURVE ( 'NONE', #29231, #35096, #31445, .T. ) ;
#56708=DIRECTION ( 'NONE',  ( 0.000000000000000000, 1.000000000000000000, 0.000000000000000000 ) ) ;
#56713=ORIENTED_EDGE ( 'NONE', *, *, #16888, .F. ) ;
#56715=VECTOR ( 'NONE', #55183, 999.9999999999998863 ) ;
#56716=FACE_OUTER_BOUND ( 'NONE', #16197, .T. ) ;
#56718=AXIS2_PLACEMENT_3D ( 'NONE', #7231, #13209, #2309 ) ;
#56722=CARTESIAN_POINT ( 'NONE',  ( 0.1230226671127766652, 25.12215469714594107, 0.000000000000000000 ) ) ;
#56723=ORIENTED_EDGE ( 'NONE', *, *, #53495, .T. ) ;
#56726=ORIENTED_EDGE ( 'NONE', *, *, #17630, .T. ) ;
#56743=CARTESIAN_POINT ( 'NONE',  ( -34.75846525699014933, 54.92585086258208804, 170.0000000000000000 ) ) ;
#56752=VERTEX_POINT ( 'NONE', #58500 ) ;
#56753=EDGE_LOOP ( 'NONE', ( #32641, #55669, #19030, #30997 ) ) ;
#56764=CIRCLE ( 'NONE', #43271, 65.00000000000000000 ) ;
#56766=DIRECTION ( 'NONE',  ( -0.000000000000000000, 0.000000000000000000, -1.000000000000000000 ) ) ;
#56779=DIRECTION ( 'NONE',  ( -0.000000000000000000, -0.000000000000000000, -1.000000000000000000 ) ) ;
#56780=CARTESIAN_POINT ( 'NONE',  ( 63.72039997003709288, 12.83396383267841223, 40.00000000000003553 ) ) ;
#56790=ORIENTED_EDGE ( 'NONE', *, *, #9396, .F. ) ;
#56793=EDGE_CURVE ( 'NONE', #27253, #57871, #59886, .T. ) ;
#56794=DIRECTION ( 'NONE',  ( -1.000000000000000000, 0.000000000000000000, 0.000000000000000000 ) ) ;
#56795=VERTEX_POINT ( 'NONE', #48619 ) ;
#56797=EDGE_CURVE ( 'NONE', #1734, #57856, #60249, .T. ) ;
#56813=CARTESIAN_POINT ( 'NONE',  ( 4.165045035620114966, 64.88046627338042072, 170.0000000000000000 ) ) ;
#56818=ORIENTED_EDGE ( 'NONE', *, *, #14530, .F. ) ;
#56823=CIRCLE ( 'NONE', #68027, 10.00000000000000000 ) ;
#56828=AXIS2_PLACEMENT_3D ( 'NONE', #55689, #54983, #1897 ) ;
#56833=DIRECTION ( 'NONE',  ( 1.000000000000000000, 0.000000000000000000, -0.000000000000000000 ) ) ;
#56841=ORIENTED_EDGE ( 'NONE', *, *, #23843, .F. ) ;
#56859=EDGE_CURVE ( 'NONE', #67530, #11439, #1874, .T. ) ;
#56864=PRODUCT_CONTEXT ( 'NONE', #10707, 'mechanical' ) ;
#56870=VECTOR ( 'NONE', #45260, 1000.000000000000000 ) ;
#56876=AXIS2_PLACEMENT_3D ( 'NONE', #741, #17254, #54177 ) ;
#56879=VECTOR ( 'NONE', #60197, 1000.000000000000227 ) ;
#56882=VERTEX_POINT ( 'NONE', #65899 ) ;
#56886=CARTESIAN_POINT ( 'NONE',  ( -41.21054189337212392, 41.29403905406989850, 27.58472369436602634 ) ) ;
#56887=LINE ( 'NONE', #62850, #41575 ) ;
#56889=DIRECTION ( 'NONE',  ( -0.000000000000000000, -0.000000000000000000, -1.000000000000000000 ) ) ;
#56892=VERTEX_POINT ( 'NONE', #461 ) ;
#56907=ORIENTED_EDGE ( 'NONE', *, *, #60280, .T. ) ;
#56908=EDGE_LOOP ( 'NONE', ( #14771, #65158, #27132, #51482 ) ) ;
#56909=CIRCLE ( 'NONE', #28845, 65.00000000000000000 ) ;
#56911=CARTESIAN_POINT ( 'NONE',  ( -39.55079474733702227, 51.59997227570980982, 170.0000000000000000 ) ) ;
#56914=CARTESIAN_POINT ( 'NONE',  ( -52.13778968636795241, 39.42540649521991014, 43.58025477438756212 ) ) ;
#56916=DIRECTION ( 'NONE',  ( -0.5128992774059071280, 0.8584487936018656562, 2.500042656554809847E-16 ) ) ;
#56934=ADVANCED_FACE ( 'NONE', ( #16976 ), #3941, .T. ) ;
#56935=ORIENTED_EDGE ( 'NONE', *, *, #25327, .F. ) ;
#56948=ORIENTED_EDGE ( 'NONE', *, *, #6251, .T. ) ;
#56949=EDGE_CURVE ( 'NONE', #35096, #31093, #24626, .T. ) ;
#56958=SURFACE_STYLE_FILL_AREA ( #67511 ) ;
#56959=CIRCLE ( 'NONE', #33356, 24.99999999999985434 ) ;
#56969=ORIENTED_EDGE ( 'NONE', *, *, #68466, .F. ) ;
#56972=EDGE_LOOP ( 'NONE', ( #62779, #23404, #26017, #15974 ) ) ;
#56976=LINE ( 'NONE', #52034, #38792 ) ;
#56984=CARTESIAN_POINT ( 'NONE',  ( 34.43940527065477397, -66.63700071734618291, 170.0000000000000000 ) ) ;
#56989=ORIENTED_EDGE ( 'NONE', *, *, #19381, .T. ) ;
#57000=CARTESIAN_POINT ( 'NONE',  ( 10.01137213834966921, -64.59476928204590251, 41.38025477438755928 ) ) ;
#57001=DIRECTION ( 'NONE',  ( -0.000000000000000000, -0.000000000000000000, 1.000000000000000000 ) ) ;
#57002=LINE ( 'NONE', #13737, #60163 ) ;
#57016=ORIENTED_EDGE ( 'NONE', *, *, #66990, .T. ) ;
#57018=AXIS2_PLACEMENT_3D ( 'NONE', #32404, #11622, #65103 ) ;
#57025=CARTESIAN_POINT ( 'NONE',  ( 8.904582680623983393, 23.36040254969773144, 0.000000000000000000 ) ) ;
#57028=CARTESIAN_POINT ( 'NONE',  ( -59.42430146430427840, 27.22983999535709998, 3.125053320693569132E-16 ) ) ;
#57033=ORIENTED_EDGE ( 'NONE', *, *, #31675, .T. ) ;
#57041=ORIENTED_EDGE ( 'NONE', *, *, #55834, .F. ) ;
#57048=CIRCLE ( 'NONE', #6474, 74.95140232871122521 ) ;
#57050=FACE_OUTER_BOUND ( 'NONE', #25170, .T. ) ;
#57055=DIRECTION ( 'NONE',  ( 0.6234898018587431423, -0.7818314824680220321, 0.000000000000000000 ) ) ;
#57058=ORIENTED_EDGE ( 'NONE', *, *, #51929, .F. ) ;
#57064=CARTESIAN_POINT ( 'NONE',  ( 0.000000000000000000, 0.000000000000000000, 40.00000000000003553 ) ) ;
#57071=CARTESIAN_POINT ( 'NONE',  ( 0.000000000000000000, 0.000000000000000000, 41.38025477438755928 ) ) ;
#57080=CARTESIAN_POINT ( 'NONE',  ( -53.17301625261200826, -40.17754262171835933, 34.48241823999801881 ) ) ;
#57083=CARTESIAN_POINT ( 'NONE',  ( -68.11501976657856972, 31.41506934893843805, 170.0000000000000000 ) ) ;
#57084=PLANE ( 'NONE',  #45496 ) ;
#57085=EDGE_CURVE ( 'NONE', #23953, #55398, #56976, .T. ) ;
#57090=ORIENTED_EDGE ( 'NONE', *, *, #53199, .T. ) ;
#57099=EDGE_CURVE ( 'NONE', #68971, #43782, #35862, .T. ) ;
#57102=B_SPLINE_CURVE_WITH_KNOTS ( 'NONE', 3,
 ( #68663, #4991, #47537, #22116 ),
 .UNSPECIFIED., .F., .F.,
 ( 4, 4 ),
 ( 0.1259919275528357807, 0.1829744153748745217 ),
 .UNSPECIFIED. ) ;
#57103=VECTOR ( 'NONE', #45083, 1000.000000000000114 ) ;
#57105=DIRECTION ( 'NONE',  ( -0.000000000000000000, -0.000000000000000000, -1.000000000000000000 ) ) ;
#57121=EDGE_CURVE ( 'NONE', #68876, #59075, #59371, .T. ) ;
#57123=VERTEX_POINT ( 'NONE', #10152 ) ;
#57130=EDGE_CURVE ( 'NONE', #22437, #51470, #53391, .T. ) ;
#57131=DIRECTION ( 'NONE',  ( -0.000000000000000000, -0.000000000000000000, -1.000000000000000000 ) ) ;
#57132=EDGE_CURVE ( 'NONE', #43717, #23495, #59025, .T. ) ;
#57136=DIRECTION ( 'NONE',  ( -0.2225209339563041788, -0.9749279121818259508, 0.000000000000000000 ) ) ;
#57138=VERTEX_POINT ( 'NONE', #63642 ) ;
#57142=ORIENTED_EDGE ( 'NONE', *, *, #18682, .T. ) ;
#57145=CARTESIAN_POINT ( 'NONE',  ( 4.165045035620114966, 64.88046627338042072, 170.0000000000000000 ) ) ;
#57146=DIRECTION ( 'NONE',  ( 0.5128992774059071280, -0.8584487936018656562, 5.102127870520019688E-18 ) ) ;
#57162=CARTESIAN_POINT ( 'NONE',  ( -11.01093400780220932, -22.58090174195397992, 0.000000000000000000 ) ) ;
#57163=CARTESIAN_POINT ( 'NONE',  ( 0.000000000000000000, 0.000000000000000000, 41.38025477438755928 ) ) ;
#57165=CARTESIAN_POINT ( 'NONE',  ( 55.14772863908675049, -34.40534879854660488, 40.00000000000003553 ) ) ;
#57166=DIRECTION ( 'NONE',  ( 1.000000000000000000, 0.000000000000000000, -0.000000000000000000 ) ) ;
#57177=CARTESIAN_POINT ( 'NONE',  ( -62.31345272479909880, 18.49415068377641447, 170.0000000000000000 ) ) ;
#57182=VERTEX_POINT ( 'NONE', #54431 ) ;
#57185=ADVANCED_FACE ( 'NONE', ( #15779 ), #11807, .T. ) ;
#57186=DIRECTION ( 'NONE',  ( -1.000000000000000000, 0.000000000000000000, 0.000000000000000000 ) ) ;
#57197=CARTESIAN_POINT ( 'NONE',  ( 24.91130694661015710, -3.250319586706349018, 3.061616997868437868E-16 ) ) ;
#57201=CARTESIAN_POINT ( 'NONE',  ( 0.000000000000000000, 0.000000000000000000, 40.00000000000003553 ) ) ;
#57215=ADVANCED_FACE ( 'NONE', ( #28410 ), #7320, .T. ) ;
#57229=ORIENTED_EDGE ( 'NONE', *, *, #24622, .F. ) ;
#57230=CARTESIAN_POINT ( 'NONE',  ( -21.27554331372911278, -61.43430442924894663, 43.58025477438756923 ) ) ;
#57231=EDGE_LOOP ( 'NONE', ( #67357, #5766, #7163, #44119, #1412, #33292, #62491, #41845, #46358 ) ) ;
#57236=VERTEX_POINT ( 'NONE', #23147 ) ;
#57240=ORIENTED_EDGE ( 'NONE', *, *, #44624, .F. ) ;
#57248=VECTOR ( 'NONE', #13887, 1000.000000000000114 ) ;
#57252=CARTESIAN_POINT ( 'NONE',  ( 0.000000000000000000, 0.000000000000000000, 43.58025477438756212 ) ) ;
#57259=CARTESIAN_POINT ( 'NONE',  ( -28.32746765835526048, 69.45586423092609607, 170.0000000000000000 ) ) ;
#57271=LINE ( 'NONE', #41436, #7512 ) ;
#57278=ORIENTED_EDGE ( 'NONE', *, *, #60993, .T. ) ;
#57283=CARTESIAN_POINT ( 'NONE',  ( 55.65793654284612302, 50.28674377798304107, 170.0000000000000000 ) ) ;
#57288=ORIENTED_EDGE ( 'NONE', *, *, #43529, .T. ) ;
#57290=AXIS2_PLACEMENT_3D ( 'NONE', #54720, #1266, #12177 ) ;
#57301=B_SPLINE_CURVE_WITH_KNOTS ( 'NONE', 3,
 ( #3773, #8723, #47359, #42098, #19966, #4127 ),
 .UNSPECIFIED., .F., .F.,
 ( 4, 2, 4 ),
 ( 1.095770181094175974E-06, 0.03239442681617710207, 0.06478775786217311206 ),
 .UNSPECIFIED. ) ;
#57302=LINE ( 'NONE', #14725, #43618 ) ;
#57312=ORIENTED_EDGE ( 'NONE', *, *, #31365, .T. ) ;
#57313=CARTESIAN_POINT ( 'NONE',  ( 0.000000000000000000, 0.000000000000000000, 0.000000000000000000 ) ) ;
#57316=ORIENTED_EDGE ( 'NONE', *, *, #27889, .T. ) ;
#57323=EDGE_CURVE ( 'NONE', #27253, #11718, #50029, .T. ) ;
#57326=CARTESIAN_POINT ( 'NONE',  ( 34.76618902119824384, -54.93755186520707667, 170.0000000000000000 ) ) ;
#57334=DIRECTION ( 'NONE',  ( -0.000000000000000000, -0.000000000000000000, 1.000000000000000000 ) ) ;
#57335=VERTEX_POINT ( 'NONE', #68806 ) ;
#57342=CARTESIAN_POINT ( 'NONE',  ( -34.75846525698938194, -54.92585086258257121, 40.00000000000003553 ) ) ;
#57343=LINE ( 'NONE', #4902, #16796 ) ;
#57345=DIRECTION ( 'NONE',  ( 0.000000000000000000, 0.000000000000000000, 1.000000000000000000 ) ) ;
#57347=CARTESIAN_POINT ( 'NONE',  ( -51.82969867401513397, 54.20961478705410030, 0.000000000000000000 ) ) ;
#57350=EDGE_CURVE ( 'NONE', #29070, #62258, #47692, .T. ) ;
#57355=LINE ( 'NONE', #14447, #3032 ) ;
#57356=DIRECTION ( 'NONE',  ( -0.000000000000000000, -0.000000000000000000, -1.000000000000000000 ) ) ;
#57357=ORIENTED_EDGE ( 'NONE', *, *, #69324, .T. ) ;
#57365=FACE_OUTER_BOUND ( 'NONE', #57822, .T. ) ;
#57366=DIRECTION ( 'NONE',  ( 4.691548276051942630E-18, 2.005263967813518922E-18, -1.000000000000000000 ) ) ;
#57368=VERTEX_POINT ( 'NONE', #66686 ) ;
#57370=ORIENTED_EDGE ( 'NONE', *, *, #61066, .F. ) ;
#57378=ORIENTED_EDGE ( 'NONE', *, *, #1044, .T. ) ;
#57396=CARTESIAN_POINT ( 'NONE',  ( -60.41792053122280493, 24.01035990323433822, 41.38025477438755928 ) ) ;
#57400=LINE ( 'NONE', #25061, #54781 ) ;
#57408=ORIENTED_EDGE ( 'NONE', *, *, #61218, .T. ) ;
#57410=AXIS2_PLACEMENT_3D ( 'NONE', #6921, #5524, #64618 ) ;
#57417=CARTESIAN_POINT ( 'NONE',  ( 60.82895951008428170, -30.68107831874537084, 170.0000000000000000 ) ) ;
#57423=CIRCLE ( 'NONE', #27079, 25.12245591505646303 ) ;
#57425=CARTESIAN_POINT ( 'NONE',  ( 13.24564585880038514, 63.65041531508843065, 170.0000000000000000 ) ) ;
#57431=ORIENTED_EDGE ( 'NONE', *, *, #65288, .T. ) ;
#57438=FACE_OUTER_BOUND ( 'NONE', #63602, .T. ) ;
#57462=FACE_OUTER_BOUND ( 'NONE', #509, .T. ) ;
#57470=EDGE_CURVE ( 'NONE', #4530, #25239, #61726, .T. ) ;
#57477=ORIENTED_EDGE ( 'NONE', *, *, #12155, .T. ) ;
#57483=DIRECTION ( 'NONE',  ( -0.7818314824680311359, 0.6234898018587318180, 2.500042656554809847E-16 ) ) ;
#57494=CARTESIAN_POINT ( 'NONE',  ( -41.50537345350632279, -50.04124777106357413, 170.0000000000000000 ) ) ;
#57502=EDGE_CURVE ( 'NONE', #31099, #28345, #40617, .T. ) ;
#57512=ORIENTED_EDGE ( 'NONE', *, *, #18743, .T. ) ;
#57513=VERTEX_POINT ( 'NONE', #62778 ) ;
#57514=EDGE_CURVE ( 'NONE', #22341, #34424, #64645, .T. ) ;
#57530=VECTOR ( 'NONE', #28756, 1000.000000000000000 ) ;
#57532=CARTESIAN_POINT ( 'NONE',  ( -17.90772993695118132, 72.84144224619132046, 43.58025477438756923 ) ) ;
#57534=CARTESIAN_POINT ( 'NONE',  ( 74.39890044415652426, -7.951074708186081530, 41.38025477438755928 ) ) ;
#57535=VECTOR ( 'NONE', #5901, 1000.000000000000227 ) ;
#57546=DIRECTION ( 'NONE',  ( -0.000000000000000000, -0.000000000000000000, 1.000000000000000000 ) ) ;
#57549=ORIENTED_EDGE ( 'NONE', *, *, #22814, .F. ) ;
#57553=LINE ( 'NONE', #30471, #54472 ) ;
#57556=ORIENTED_EDGE ( 'NONE', *, *, #17114, .F. ) ;
#57561=ORIENTED_EDGE ( 'NONE', *, *, #33124, .T. ) ;
#57573=LINE ( 'NONE', #9383, #30860 ) ;
#57586=ORIENTED_EDGE ( 'NONE', *, *, #42926, .T. ) ;
#57592=CARTESIAN_POINT ( 'NONE',  ( 74.39890044415652426, -7.951074708186050444, 170.0000000000000000 ) ) ;
#57602=EDGE_CURVE ( 'NONE', #13054, #27636, #5055, .T. ) ;
#57604=CARTESIAN_POINT ( 'NONE',  ( -16.68907004672281502, -73.11959341363693454, 43.58025477438756212 ) ) ;
#57605=CARTESIAN_POINT ( 'NONE',  ( -66.97713359923356791, 33.64188291208976977, 41.38025477438755928 ) ) ;
#57615=FACE_OUTER_BOUND ( 'NONE', #44067, .T. ) ;
#57624=VERTEX_POINT ( 'NONE', #475 ) ;
#57626=ORIENTED_EDGE ( 'NONE', *, *, #4908, .F. ) ;
#57632=CARTESIAN_POINT ( 'NONE',  ( -37.04655464516844177, 53.85410457537858520, 43.58025477438756212 ) ) ;
#57635=VECTOR ( 'NONE', #51830, 1000.000000000000114 ) ;
#57639=DIRECTION ( 'NONE',  ( 0.000000000000000000, -1.000000000000000000, 5.102127870520020458E-18 ) ) ;
#57650=ORIENTED_EDGE ( 'NONE', *, *, #8349, .F. ) ;
#57652=DIRECTION ( 'NONE',  ( 0.9639628606958550172, -0.2660368455666687892, 0.000000000000000000 ) ) ;
#57654=DIRECTION ( 'NONE',  ( -0.1342332658176522420, -0.9909497617679352555, 0.000000000000000000 ) ) ;
#57657=EDGE_CURVE ( 'NONE', #24361, #66914, #56823, .T. ) ;
#57664=ADVANCED_FACE ( 'NONE', ( #31120 ), #31455, .T. ) ;
#57671=AXIS2_PLACEMENT_3D ( 'NONE', #20315, #20660, #41779 ) ;
#57672=VERTEX_POINT ( 'NONE', #5408 ) ;
#57678=CARTESIAN_POINT ( 'NONE',  ( 0.000000000000000000, 0.000000000000000000, 170.0000000000000000 ) ) ;
#57682=ORIENTED_EDGE ( 'NONE', *, *, #4681, .F. ) ;
#57687=CARTESIAN_POINT ( 'NONE',  ( -27.92096212090788399, 31.01184537397639929, 13.79046340968177908 ) ) ;
#57690=EDGE_CURVE ( 'NONE', #49450, #56234, #10722, .T. ) ;
#57695=CARTESIAN_POINT ( 'NONE',  ( 60.74750367560205433, 24.13405452624939329, 43.58025477438756212 ) ) ;
#57696=ORIENTED_EDGE ( 'NONE', *, *, #42418, .F. ) ;
#57700=CARTESIAN_POINT ( 'NONE',  ( 0.000000000000000000, 0.000000000000000000, 0.000000000000000000 ) ) ;
#57711=DIRECTION ( 'NONE',  ( -0.000000000000000000, -0.000000000000000000, -1.000000000000000000 ) ) ;
#57723=EDGE_CURVE ( 'NONE', #695, #19391, #10330, .T. ) ;
#57738=ORIENTED_EDGE ( 'NONE', *, *, #66253, .F. ) ;
#57757=CARTESIAN_POINT ( 'NONE',  ( 4.165045035621076863, -64.88046627338039229, 41.38025477438755928 ) ) ;
#57759=VECTOR ( 'NONE', #20925, 1000.000000000000227 ) ;
#57761=AXIS2_PLACEMENT_3D ( 'NONE', #21968, #49031, #26563 ) ;
#57764=CARTESIAN_POINT ( 'NONE',  ( 51.85299110299440173, 39.21848821248450179, 41.38025477438755928 ) ) ;
#57776=ORIENTED_EDGE ( 'NONE', *, *, #69525, .F. ) ;
#57778=ORIENTED_EDGE ( 'NONE', *, *, #44777, .F. ) ;
#57789=CARTESIAN_POINT ( 'NONE',  ( 50.59696764854425766, 10.45241199037308455, 26.66469066592268433 ) ) ;
#57797=DIRECTION ( 'NONE',  ( -1.000000000000000000, 0.000000000000000000, 0.000000000000000000 ) ) ;
#57809=CARTESIAN_POINT ( 'NONE',  ( 11.30618213853490239, -74.15344055032291237, 170.0000000000000000 ) ) ;
#57815=AXIS2_PLACEMENT_3D ( 'NONE', #26901, #48327, #33588 ) ;
#57819=AXIS2_PLACEMENT_3D ( 'NONE', #42073, #48028, #58932 ) ;
#57822=EDGE_LOOP ( 'NONE', ( #59925, #56790, #9075, #31689, #67062, #23318, #22385, #32022, #30694 ) ) ;
#57823=AXIS2_PLACEMENT_3D ( 'NONE', #25487, #46926, #54512 ) ;
#57830=CARTESIAN_POINT ( 'NONE',  ( -48.12872802574264597, 43.70867239603710885, 3.061616997868437868E-16 ) ) ;
#57844=ORIENTED_EDGE ( 'NONE', *, *, #33829, .F. ) ;
#57845=ORIENTED_EDGE ( 'NONE', *, *, #15570, .T. ) ;
#57855=ORIENTED_EDGE ( 'NONE', *, *, #36906, .T. ) ;
#57856=VERTEX_POINT ( 'NONE', #23674 ) ;
#57871=VERTEX_POINT ( 'NONE', #60607 ) ;
#57876=LINE ( 'NONE', #3378, #18076 ) ;
#57880=CARTESIAN_POINT ( 'NONE',  ( -65.36598343705435354, 0.000000000000000000, 41.38025477438755928 ) ) ;
#57887=EDGE_CURVE ( 'NONE', #23937, #31009, #13000, .T. ) ;
#57893=DIRECTION ( 'NONE',  ( -0.000000000000000000, 0.000000000000000000, -1.000000000000000000 ) ) ;
#57897=ORIENTED_EDGE ( 'NONE', *, *, #15410, .F. ) ;
#57905=CARTESIAN_POINT ( 'NONE',  ( -40.27405704175546930, -63.28161525591320924, 170.0000000000000000 ) ) ;
#57941=ADVANCED_FACE ( 'NONE', ( #12079 ), #54625, .T. ) ;
#57952=CARTESIAN_POINT ( 'NONE',  ( 39.48989092546764823, -13.48566889876655672, 13.79046412312118974 ) ) ;
#57955=LINE ( 'NONE', #62193, #19251 ) ;
#57959=AXIS2_PLACEMENT_3D ( 'NONE', #33240, #13175, #33591 ) ;
#57961=ORIENTED_EDGE ( 'NONE', *, *, #15549, .F. ) ;
#57968=CARTESIAN_POINT ( 'NONE',  ( 45.82394788922798767, 46.11928342727497210, 170.0000000000000000 ) ) ;
#57972=EDGE_CURVE ( 'NONE', #66237, #32020, #54973, .T. ) ;
#57981=DIRECTION ( 'NONE',  ( 0.000000000000000000, 0.000000000000000000, 1.000000000000000000 ) ) ;
#57983=ORIENTED_EDGE ( 'NONE', *, *, #809, .F. ) ;
#58012=PLANE ( 'NONE',  #31700 ) ;
#58014=CARTESIAN_POINT ( 'NONE',  ( 51.65020379092739944, 1.250000000000015099, 26.66469066592269499 ) ) ;
#58031=EDGE_LOOP ( 'NONE', ( #38627, #45738, #20083, #24516 ) ) ;
#58032=ADVANCED_FACE ( 'NONE', ( #34924 ), #8575, .T. ) ;
#58042=ORIENTED_EDGE ( 'NONE', *, *, #47796, .T. ) ;
#58044=CARTESIAN_POINT ( 'NONE',  ( -2.368959188627552503, -24.88750755625419941, 0.000000000000000000 ) ) ;
#58053=VECTOR ( 'NONE', #26113, 1000.000000000000000 ) ;
#58057=EDGE_CURVE ( 'NONE', #57368, #33912, #51451, .T. ) ;
#58059=ORIENTED_EDGE ( 'NONE', *, *, #11970, .F. ) ;
#58060=DIRECTION ( 'NONE',  ( 0.04486483035051862939, -0.9989930665413143673, 0.000000000000000000 ) ) ;
#58061=VECTOR ( 'NONE', #67007, 1000.000000000000000 ) ;
#58062=VERTEX_POINT ( 'NONE', #56722 ) ;
#58067=CIRCLE ( 'NONE', #35734, 65.00000000000000000 ) ;
#58070=VERTEX_POINT ( 'NONE', #13129 ) ;
#58079=EDGE_CURVE ( 'NONE', #66442, #22625, #67979, .T. ) ;
#58093=LINE ( 'NONE', #26085, #17415 ) ;
#58105=DIRECTION ( 'NONE',  ( -0.9749279121818227312, -0.2225209339563184729, 2.500042656554810833E-16 ) ) ;
#58110=DIRECTION ( 'NONE',  ( 0.000000000000000000, 0.000000000000000000, 1.000000000000000000 ) ) ;
#58120=VERTEX_POINT ( 'NONE', #4625 ) ;
#58122=EDGE_LOOP ( 'NONE', ( #23163, #49148, #56723, #23500 ) ) ;
#58125=FACE_OUTER_BOUND ( 'NONE', #8752, .T. ) ;
#58129=DIRECTION ( 'NONE',  ( -1.000000000000000000, 0.000000000000000000, 0.000000000000000000 ) ) ;
#58130=DIRECTION ( 'NONE',  ( 0.000000000000000000, 0.000000000000000000, 1.000000000000000000 ) ) ;
#58136=LINE ( 'NONE', #8918, #51037 ) ;
#58139=EDGE_CURVE ( 'NONE', #35639, #56892, #44507, .T. ) ;
#58143=CARTESIAN_POINT ( 'NONE',  ( -65.36598343705435354, 0.000000000000000000, 41.38025477438755928 ) ) ;
#58144=VECTOR ( 'NONE', #45889, 1000.000000000000114 ) ;
#58151=ORIENTED_EDGE ( 'NONE', *, *, #39858, .F. ) ;
#58155=CARTESIAN_POINT ( 'NONE',  ( -2.113472939309121834, -74.92159864268212743, 41.38025477438755928 ) ) ;
#58163=EDGE_LOOP ( 'NONE', ( #21438, #26003, #49391, #6262 ) ) ;
#58169=ORIENTED_EDGE ( 'NONE', *, *, #55277, .T. ) ;
#58171=DIRECTION ( 'NONE',  ( -0.3930250316539148359, -0.9195277725514544587, 0.000000000000000000 ) ) ;
#58191=AXIS2_PLACEMENT_3D ( 'NONE', #59245, #60300, #511 ) ;
#58200=EDGE_CURVE ( 'NONE', #20027, #35779, #58772, .T. ) ;
#58204=CARTESIAN_POINT ( 'NONE',  ( -62.31345272479909880, 18.49415068377641447, 170.0000000000000000 ) ) ;
#58209=ORIENTED_EDGE ( 'NONE', *, *, #61795, .T. ) ;
#58210=AXIS2_PLACEMENT_3D ( 'NONE', #5349, #12012, #26803 ) ;
#58211=DIRECTION ( 'NONE',  ( -0.000000000000000000, -0.000000000000000000, -1.000000000000000000 ) ) ;
#58215=EDGE_CURVE ( 'NONE', #9408, #56892, #9000, .T. ) ;
#58219=FACE_OUTER_BOUND ( 'NONE', #19599, .T. ) ;
#58223=CARTESIAN_POINT ( 'NONE',  ( 12.99074365121421692, 21.50298515537768296, 0.000000000000000000 ) ) ;
#58227=LINE ( 'NONE', #37806, #22001 ) ;
#58236=VERTEX_POINT ( 'NONE', #9573 ) ;
#58253=CARTESIAN_POINT ( 'NONE',  ( 2.112947028649122760, -24.91054906769651112, 0.000000000000000000 ) ) ;
#58254=ORIENTED_EDGE ( 'NONE', *, *, #29392, .T. ) ;
#58257=CARTESIAN_POINT ( 'NONE',  ( 41.49663191311347532, 50.03028622612080767, 40.00000000000003553 ) ) ;
#58282=ORIENTED_EDGE ( 'NONE', *, *, #32132, .F. ) ;
#58288=EDGE_CURVE ( 'NONE', #42865, #38399, #41106, .T. ) ;
#58290=DIRECTION ( 'NONE',  ( 0.5877852522924686962, 0.8090169943749506709, 5.102127870520021228E-18 ) ) ;
#58291=AXIS2_PLACEMENT_3D ( 'NONE', #6439, #1871, #44771 ) ;
#58299=DIRECTION ( 'NONE',  ( -0.000000000000000000, 0.000000000000000000, -1.000000000000000000 ) ) ;
#58302=CARTESIAN_POINT ( 'NONE',  ( -50.88541732109732862, -55.03078243218159571, 41.38025477438755928 ) ) ;
#58308=ORIENTED_EDGE ( 'NONE', *, *, #16732, .F. ) ;
#58320=ORIENTED_EDGE ( 'NONE', *, *, #11464, .F. ) ;
#58325=CARTESIAN_POINT ( 'NONE',  ( -42.52062419515534941, 29.34795682323898092, 26.66469066592269144 ) ) ;
#58326=ORIENTED_EDGE ( 'NONE', *, *, #64005, .T. ) ;
#58329=ORIENTED_EDGE ( 'NONE', *, *, #7472, .F. ) ;
#58333=CARTESIAN_POINT ( 'NONE',  ( 0.000000000000000000, 0.000000000000000000, 41.38025477438755928 ) ) ;
#58336=ORIENTED_EDGE ( 'NONE', *, *, #56793, .F. ) ;
#58338=CARTESIAN_POINT ( 'NONE',  ( 14.77197008895680597, 49.50853412630286954, 26.66469066592269144 ) ) ;
#58340=DIRECTION ( 'NONE',  ( -0.000000000000000000, -0.000000000000000000, -1.000000000000000000 ) ) ;
#58351=EDGE_LOOP ( 'NONE', ( #23635, #531, #44387, #57586 ) ) ;
#58358=CARTESIAN_POINT ( 'NONE',  ( 0.000000000000000000, 0.000000000000000000, 41.38025477438755928 ) ) ;
#58359=DIRECTION ( 'NONE',  ( 0.1342332658176522420, 0.9909497617679351444, 0.000000000000000000 ) ) ;
#58360=DIRECTION ( 'NONE',  ( 1.000000000000000000, 0.000000000000000000, -0.000000000000000000 ) ) ;
#58361=CARTESIAN_POINT ( 'NONE',  ( 26.98325939156676867, -31.83109271837644627, 13.79046412397660859 ) ) ;
#58362=CARTESIAN_POINT ( 'NONE',  ( 0.000000000000000000, 0.000000000000000000, 40.00000000000003553 ) ) ;
#58368=EDGE_CURVE ( 'NONE', #28358, #64523, #69205, .T. ) ;
#58378=B_SPLINE_CURVE_WITH_KNOTS ( 'NONE', 3,
 ( #23100, #12901, #66031, #17099 ),
 .UNSPECIFIED., .F., .F.,
 ( 4, 4 ),
 ( 9.900409499088329389E-07, 0.05658314289920115397 ),
 .UNSPECIFIED. ) ;
#58379=LINE ( 'NONE', #42882, #12841 ) ;
#58382=ORIENTED_EDGE ( 'NONE', *, *, #53734, .T. ) ;
#58387=ORIENTED_EDGE ( 'NONE', *, *, #55506, .T. ) ;
#58388=CIRCLE ( 'NONE', #38155, 65.00000000000000000 ) ;
#58399=DIRECTION ( 'NONE',  ( 1.000000000000000000, 3.730349362740526607E-14, 0.000000000000000000 ) ) ;
#58400=CARTESIAN_POINT ( 'NONE',  ( -84.49322488516129681, 0.000000000000000000, 43.58025477438756212 ) ) ;
#58402=CARTESIAN_POINT ( 'NONE',  ( -50.92620509423012720, -55.07344309828840068, 170.0000000000000000 ) ) ;
#58404=CONICAL_SURFACE ( 'NONE', #28075, 65.00000000000000000, 0.7853981633974497223 ) ;
#58408=DIRECTION ( 'NONE',  ( -2.477416674922659623E-16, -3.355888904728274975E-17, 1.000000000000000000 ) ) ;
#58412=ORIENTED_EDGE ( 'NONE', *, *, #52121, .T. ) ;
#58430=ORIENTED_EDGE ( 'NONE', *, *, #30929, .T. ) ;
#58431=CIRCLE ( 'NONE', #27965, 65.36598343705435354 ) ;
#58437=CARTESIAN_POINT ( 'NONE',  ( -53.31111153860302210, 37.18770477615724701, 40.00000000000003553 ) ) ;
#58439=DIRECTION ( 'NONE',  ( -4.492911005741634170E-18, -2.417738509769586184E-18, -1.000000000000000000 ) ) ;
#58443=VERTEX_POINT ( 'NONE', #2829 ) ;
#58446=ORIENTED_EDGE ( 'NONE', *, *, #5009, .F. ) ;
#58451=CARTESIAN_POINT ( 'NONE',  ( 11.51073115475400677, -31.38130280396068983, 6.893342932533044198 ) ) ;
#58455=EDGE_CURVE ( 'NONE', #33141, #65664, #31013, .T. ) ;
#58474=CARTESIAN_POINT ( 'NONE',  ( 34.41143668122512622, -66.58502636910473882, 41.38025477438755928 ) ) ;
#58485=DIRECTION ( 'NONE',  ( -1.000000000000000000, 0.000000000000000000, 0.000000000000000000 ) ) ;
#58493=EDGE_LOOP ( 'NONE', ( #40949, #28145, #37266, #1862 ) ) ;
#58495=CARTESIAN_POINT ( 'NONE',  ( 37.47470427701602347, -8.071072281209895394, 13.32819397642332504 ) ) ;
#58500=CARTESIAN_POINT ( 'NONE',  ( -64.61430802170482934, -7.070445451048283481, 40.00000000000003553 ) ) ;
#58505=VECTOR ( 'NONE', #32828, 1000.000000000000000 ) ;
#58517=ADVANCED_FACE ( 'NONE', ( #31299 ), #64582, .T. ) ;
#58519=CARTESIAN_POINT ( 'NONE',  ( 29.86848256228606502, -58.14280299503694494, 43.58025477438756212 ) ) ;
#58520=CARTESIAN_POINT ( 'NONE',  ( 8.820885042878503057, -74.43053605947400797, 41.38025477438755928 ) ) ;
#58521=DIRECTION ( 'NONE',  ( -0.000000000000000000, -0.000000000000000000, -1.000000000000000000 ) ) ;
#58522=CARTESIAN_POINT ( 'NONE',  ( 0.000000000000000000, 0.000000000000000000, 43.58025477438756212 ) ) ;
#58535=EDGE_CURVE ( 'NONE', #61844, #55150, #10508, .T. ) ;
#58539=ORIENTED_EDGE ( 'NONE', *, *, #53962, .T. ) ;
#58540=ORIENTED_EDGE ( 'NONE', *, *, #16721, .T. ) ;
#58551=CARTESIAN_POINT ( 'NONE',  ( 6.381648998658842054, 37.79907703206831826, 13.32819397642332859 ) ) ;
#58552=DIRECTION ( 'NONE',  ( 0.7530714660036099684, 0.6579387259397136978, 0.000000000000000000 ) ) ;
#58553=DIRECTION ( 'NONE',  ( 0.000000000000000000, 0.000000000000000000, 1.000000000000000000 ) ) ;
#58556=CARTESIAN_POINT ( 'NONE',  ( 48.11816970607300448, -43.69944786993950459, 170.0000000000000000 ) ) ;
#58558=AXIS2_PLACEMENT_3D ( 'NONE', #8185, #51100, #39165 ) ;
#58562=CIRCLE ( 'NONE', #67582, 74.95140232871122521 ) ;
#58569=ORIENTED_EDGE ( 'NONE', *, *, #816, .F. ) ;
#58577=VERTEX_POINT ( 'NONE', #6546 ) ;
#58586=EDGE_LOOP ( 'NONE', ( #54080, #58151, #20074, #9477, #19326, #55060, #33119, #1777, #62396 ) ) ;
#58590=ADVANCED_FACE ( 'NONE', ( #33978 ), #60354, .T. ) ;
#58598=ORIENTED_EDGE ( 'NONE', *, *, #37816, .T. ) ;
#58601=AXIS2_PLACEMENT_3D ( 'NONE', #39941, #8978, #3350 ) ;
#58602=AXIS2_PLACEMENT_3D ( 'NONE', #8492, #56321, #18002 ) ;
#58605=DIRECTION ( 'NONE',  ( -1.000000000000000000, 0.000000000000000000, 0.000000000000000000 ) ) ;
#58613=DIRECTION ( 'NONE',  ( 0.000000000000000000, 0.000000000000000000, 1.000000000000000000 ) ) ;
#58615=CARTESIAN_POINT ( 'NONE',  ( 22.93737758745371735, 9.943676855699235873, 0.000000000000000000 ) ) ;
#58626=DIRECTION ( 'NONE',  ( 1.000000000000000000, 0.000000000000000000, 0.000000000000000000 ) ) ;
#58629=DIRECTION ( 'NONE',  ( 2.213730317917102779E-18, 4.596858371395816895E-18, -1.000000000000000000 ) ) ;
#58631=DIRECTION ( 'NONE',  ( 1.000000000000000000, 0.000000000000000000, 0.000000000000000000 ) ) ;
#58632=CARTESIAN_POINT ( 'NONE',  ( -8.663926357539105894, 23.45072237844991747, 0.000000000000000000 ) ) ;
#58643=ORIENTED_EDGE ( 'NONE', *, *, #32863, .F. ) ;
#58649=EDGE_CURVE ( 'NONE', #64355, #45918, #55597, .T. ) ;
#58654=AXIS2_PLACEMENT_3D ( 'NONE', #65094, #34142, #59797 ) ;
#58656=EDGE_CURVE ( 'NONE', #41223, #49197, #17801, .T. ) ;
#58669=VECTOR ( 'NONE', #26254, 1000.000000000000000 ) ;
#58670=ORIENTED_EDGE ( 'NONE', *, *, #59213, .F. ) ;
#58682=ORIENTED_EDGE ( 'NONE', *, *, #30411, .T. ) ;
#58687=VERTEX_POINT ( 'NONE', #56120 ) ;
#58698=CARTESIAN_POINT ( 'NONE',  ( -60.41792053122248518, -24.01035990323518021, 170.0000000000000000 ) ) ;
#58700=CARTESIAN_POINT ( 'NONE',  ( 0.000000000000000000, 0.000000000000000000, 73.58025477438756923 ) ) ;
#58711=CIRCLE ( 'NONE', #67734, 65.36598343705435354 ) ;
#58715=EDGE_CURVE ( 'NONE', #8339, #62331, #7937, .T. ) ;
#58716=DIRECTION ( 'NONE',  ( -0.000000000000000000, -0.000000000000000000, -1.000000000000000000 ) ) ;
#58719=VERTEX_POINT ( 'NONE', #17077 ) ;
#58725=ORIENTED_EDGE ( 'NONE', *, *, #31825, .T. ) ;
#58732=DIRECTION ( 'NONE',  ( 0.000000000000000000, 0.000000000000000000, 1.000000000000000000 ) ) ;
#58737=VERTEX_POINT ( 'NONE', #29388 ) ;
#58743=EDGE_CURVE ( 'NONE', #23096, #42469, #50844, .T. ) ;
#58753=EDGE_LOOP ( 'NONE', ( #26360, #69294, #33491, #52288 ) ) ;
#58764=ORIENTED_EDGE ( 'NONE', *, *, #24952, .T. ) ;
#58765=CARTESIAN_POINT ( 'NONE',  ( 0.000000000000000000, 0.000000000000000000, 0.000000000000000000 ) ) ;
#58772=LINE ( 'NONE', #57757, #65874 ) ;
#58775=CARTESIAN_POINT ( 'NONE',  ( 74.01791526339553684, 12.16185512414947034, 170.0000000000000000 ) ) ;
#58780=CYLINDRICAL_SURFACE ( 'NONE', #61775, 65.36598343705435354 ) ;
#58789=ORIENTED_EDGE ( 'NONE', *, *, #34739, .T. ) ;
#58795=LINE ( 'NONE', #32770, #51503 ) ;
#58796=CARTESIAN_POINT ( 'NONE',  ( -24.39249304643357519, -60.24953346690487166, 40.00000000000003553 ) ) ;
#58803=LINE ( 'NONE', #47552, #2653 ) ;
#58805=AXIS2_PLACEMENT_3D ( 'NONE', #66026, #23097, #17820 ) ;
#58807=AXIS2_PLACEMENT_3D ( 'NONE', #26227, #10379, #68450 ) ;
#58813=VECTOR ( 'NONE', #61344, 1000.000000000000000 ) ;
#58815=VERTEX_POINT ( 'NONE', #41336 ) ;
#58825=EDGE_CURVE ( 'NONE', #45918, #3538, #4047, .T. ) ;
#58826=ADVANCED_FACE ( 'NONE', ( #20551 ), #43386, .T. ) ;
#58827=ORIENTED_EDGE ( 'NONE', *, *, #59236, .F. ) ;
#58828=LINE ( 'NONE', #50377, #57103 ) ;
#58829=CARTESIAN_POINT ( 'NONE',  ( 0.000000000000000000, 0.000000000000000000, 40.00000000000003553 ) ) ;
#58839=ORIENTED_EDGE ( 'NONE', *, *, #63068, .F. ) ;
#58846=VECTOR ( 'NONE', #34267, 1000.000000000000000 ) ;
#58850=EDGE_CURVE ( 'NONE', #23357, #38023, #3938, .T. ) ;
#58867=PLANE ( 'NONE',  #34374 ) ;
#58877=CARTESIAN_POINT ( 'NONE',  ( -67.03031041878422513, -33.66749151869545642, 43.58025477438756923 ) ) ;
#58889=DIRECTION ( 'NONE',  ( 1.000000000000000000, 2.575717417130363489E-14, 0.000000000000000000 ) ) ;
#58895=ORIENTED_EDGE ( 'NONE', *, *, #211, .F. ) ;
#58904=EDGE_CURVE ( 'NONE', #54048, #34240, #43726, .T. ) ;
#58910=EDGE_CURVE ( 'NONE', #30082, #47961, #49698, .T. ) ;
#58912=CARTESIAN_POINT ( 'NONE',  ( 56.48035995027147749, -49.34540444547771187, 0.000000000000000000 ) ) ;
#58913=FACE_OUTER_BOUND ( 'NONE', #20588, .T. ) ;
#58917=ORIENTED_EDGE ( 'NONE', *, *, #52575, .F. ) ;
#58921=ORIENTED_EDGE ( 'NONE', *, *, #67658, .T. ) ;
#58927=LINE ( 'NONE', #64565, #18744 ) ;
#58928=CARTESIAN_POINT ( 'NONE',  ( 0.000000000000000000, 0.000000000000000000, 41.38025477438755928 ) ) ;
#58929=ADVANCED_FACE ( 'NONE', ( #54637 ), #7304, .T. ) ;
#58932=DIRECTION ( 'NONE',  ( -1.000000000000000000, 0.000000000000000000, 0.000000000000000000 ) ) ;
#58935=ORIENTED_EDGE ( 'NONE', *, *, #55332, .T. ) ;
#58937=VECTOR ( 'NONE', #62444, 1000.000000000000000 ) ;
#58941=VECTOR ( 'NONE', #48272, 1000.000000000000000 ) ;
#58944=LINE ( 'NONE', #10763, #6063 ) ;
#58947=EDGE_LOOP ( 'NONE', ( #24355, #57897, #14666, #30229, #2032, #25717, #16548, #20047, #3727 ) ) ;
#58954=CARTESIAN_POINT ( 'NONE',  ( -38.04732649588432736, -4.679373836065037651, 13.32819299319724493 ) ) ;
#58955=VECTOR ( 'NONE', #69062, 1000.000000000000000 ) ;
#58958=ORIENTED_EDGE ( 'NONE', *, *, #1499, .T. ) ;
#58967=CARTESIAN_POINT ( 'NONE',  ( 17.05487753766634285, -34.33113485734955361, 13.32819397642332504 ) ) ;
#58973=VERTEX_POINT ( 'NONE', #56042 ) ;
#58976=DIRECTION ( 'NONE',  ( 1.000000000000000000, 0.000000000000000000, 0.000000000000000000 ) ) ;
#58981=CARTESIAN_POINT ( 'NONE',  ( 26.69682282325795697, -59.27986298182186431, 170.0000000000000000 ) ) ;
#58985=ORIENTED_EDGE ( 'NONE', *, *, #871, .T. ) ;
#58989=CARTESIAN_POINT ( 'NONE',  ( -38.27142574863722047, -2.189438189322980843, 13.32819397642333037 ) ) ;
#58996=ORIENTED_EDGE ( 'NONE', *, *, #31073, .F. ) ;
#59014=DIRECTION ( 'NONE',  ( -0.9639628606958550172, 0.2660368455666687892, 0.000000000000000000 ) ) ;
#59020=DIRECTION ( 'NONE',  ( -1.000000000000000000, 0.000000000000000000, 0.000000000000000000 ) ) ;
#59025=LINE ( 'NONE', #38265, #8468 ) ;
#59028=CARTESIAN_POINT ( 'NONE',  ( 18.89356949897823768, 62.19351277735707839, 40.00000000000003553 ) ) ;
#59030=ORIENTED_EDGE ( 'NONE', *, *, #8179, .F. ) ;
#59032=LINE ( 'NONE', #10853, #47688 ) ;
#59035=ORIENTED_EDGE ( 'NONE', *, *, #2326, .F. ) ;
#59049=EDGE_CURVE ( 'NONE', #41081, #43897, #52144, .T. ) ;
#59055=ORIENTED_EDGE ( 'NONE', *, *, #10165, .F. ) ;
#59061=EDGE_CURVE ( 'NONE', #52558, #17523, #43295, .T. ) ;
#59067=CARTESIAN_POINT ( 'NONE',  ( -4.164416015344991173, -64.86646004871191451, 40.00000000000003553 ) ) ;
#59069=ORIENTED_EDGE ( 'NONE', *, *, #47545, .T. ) ;
#59074=ADVANCED_FACE ( 'NONE', ( #69355 ), #31384, .F. ) ;
#59075=VERTEX_POINT ( 'NONE', #15888 ) ;
#59078=VERTEX_POINT ( 'NONE', #53152 ) ;
#59085=DIRECTION ( 'NONE',  ( 1.000000000000000000, 1.776356839400250465E-14, 0.000000000000000000 ) ) ;
#59092=CYLINDRICAL_SURFACE ( 'NONE', #16180, 65.00000000000000000 ) ;
#59098=VERTEX_POINT ( 'NONE', #25772 ) ;
#59100=VECTOR ( 'NONE', #50151, 999.9999999999998863 ) ;
#59105=VECTOR ( 'NONE', #14525, 1000.000000000000000 ) ;
#59108=FACE_OUTER_BOUND ( 'NONE', #7995, .T. ) ;
#59120=CARTESIAN_POINT ( 'NONE',  ( -40.24154210098712525, -63.23235722614506216, 41.38025477438755928 ) ) ;
#59122=CARTESIAN_POINT ( 'NONE',  ( 0.000000000000000000, 0.000000000000000000, 170.0000000000000000 ) ) ;
#59127=PLANE ( 'NONE',  #24949 ) ;
#59136=DIRECTION ( 'NONE',  ( 0.000000000000000000, 0.000000000000000000, 1.000000000000000000 ) ) ;
#59145=AXIS2_PLACEMENT_3D ( 'NONE', #66233, #33855, #65882 ) ;
#59146=CARTESIAN_POINT ( 'NONE',  ( 0.000000000000000000, 0.000000000000000000, 41.38025477438755928 ) ) ;
#59152=CARTESIAN_POINT ( 'NONE',  ( 61.28323125814100081, 21.66484633135460669, 170.0000000000000000 ) ) ;
#59154=VECTOR ( 'NONE', #43115, 1000.000000000000000 ) ;
#59155=DIRECTION ( 'NONE',  ( 1.000000000000000000, 0.000000000000000000, 0.000000000000000000 ) ) ;
#59157=B_SPLINE_CURVE_WITH_KNOTS ( 'NONE', 3,
 ( #14521, #58451, #69007, #68669, #20144, #47544 ),
 .UNSPECIFIED., .F., .F.,
 ( 4, 2, 4 ),
 ( 0.03218935267740785644, 0.06469833035354445594, 0.09720730802968105544 ),
 .UNSPECIFIED. ) ;
#59165=CARTESIAN_POINT ( 'NONE',  ( 10.78925482157266913, -22.68765681156003566, 0.000000000000000000 ) ) ;
#59168=B_SPLINE_CURVE_WITH_KNOTS ( 'NONE', 3,
 ( #28500, #66850, #6345, #23578 ),
 .UNSPECIFIED., .F., .F.,
 ( 4, 4 ),
 ( 9.900409499146238914E-07, 0.05658314289920116785 ),
 .UNSPECIFIED. ) ;
#59182=CARTESIAN_POINT ( 'NONE',  ( -65.00200000000002376, -1.250000000000021760, 41.38025477438755928 ) ) ;
#59184=ORIENTED_EDGE ( 'NONE', *, *, #51217, .F. ) ;
#59185=AXIS2_PLACEMENT_3D ( 'NONE', #66042, #44565, #32280 ) ;
#59210=DIRECTION ( 'NONE',  ( 1.000000000000000000, 0.000000000000000000, 0.000000000000000000 ) ) ;
#59211=ADVANCED_FACE ( 'NONE', ( #24654 ), #29921, .F. ) ;
#59213=EDGE_CURVE ( 'NONE', #1085, #67017, #35194, .T. ) ;
#59219=ORIENTED_EDGE ( 'NONE', *, *, #34578, .T. ) ;
#59236=EDGE_CURVE ( 'NONE', #55870, #35197, #1678, .T. ) ;
#59238=DIRECTION ( 'NONE',  ( -0.3930250316539148359, -0.9195277725514544587, 0.000000000000000000 ) ) ;
#59243=EDGE_CURVE ( 'NONE', #39395, #9288, #14079, .T. ) ;
#59244=VECTOR ( 'NONE', #15954, 1000.000000000000114 ) ;
#59245=CARTESIAN_POINT ( 'NONE',  ( 0.000000000000000000, 0.000000000000000000, 43.58025477438756212 ) ) ;
#59251=DIRECTION ( 'NONE',  ( -0.000000000000000000, -0.000000000000000000, 1.000000000000000000 ) ) ;
#59252=FACE_OUTER_BOUND ( 'NONE', #42539, .T. ) ;
#59253=DIRECTION ( 'NONE',  ( -0.7227948638273978821, 0.6910626489868580968, 0.000000000000000000 ) ) ;
#59256=VERTEX_POINT ( 'NONE', #17498 ) ;
#59257=DIRECTION ( 'NONE',  ( 0.08963930890342654279, 0.9959742939952397345, 0.000000000000000000 ) ) ;
#59265=PLANE ( 'NONE',  #52714 ) ;
#59272=DIRECTION ( 'NONE',  ( -0.000000000000000000, -0.000000000000000000, 1.000000000000000000 ) ) ;
#59287=VECTOR ( 'NONE', #57981, 1000.000000000000000 ) ;
#59293=ORIENTED_EDGE ( 'NONE', *, *, #4673, .F. ) ;
#59295=CARTESIAN_POINT ( 'NONE',  ( 26.69682282325711853, 59.27986298182223379, 3.061616997868437868E-16 ) ) ;
#59299=EDGE_CURVE ( 'NONE', #6300, #1969, #48072, .T. ) ;
#59316=CARTESIAN_POINT ( 'NONE',  ( 6.837601902335299187, 41.16505653441733870, 13.79046340968177553 ) ) ;
#59329=EDGE_CURVE ( 'NONE', #4465, #16163, #15392, .T. ) ;
#59351=DIRECTION ( 'NONE',  ( -0.000000000000000000, -0.000000000000000000, -1.000000000000000000 ) ) ;
#59358=VERTEX_POINT ( 'NONE', #1637 ) ;
#59368=EDGE_CURVE ( 'NONE', #23953, #68299, #58378, .T. ) ;
#59371=LINE ( 'NONE', #21737, #49978 ) ;
#59374=FACE_OUTER_BOUND ( 'NONE', #44173, .T. ) ;
#59390=AXIS2_PLACEMENT_3D ( 'NONE', #50935, #34069, #17528 ) ;
#59395=PLANE ( 'NONE',  #4463 ) ;
#59400=ORIENTED_EDGE ( 'NONE', *, *, #41240, .T. ) ;
#59401=PLANE ( 'NONE',  #41941 ) ;
#59410=ORIENTED_EDGE ( 'NONE', *, *, #64243, .T. ) ;
#59412=DIRECTION ( 'NONE',  ( -0.000000000000000000, -0.000000000000000000, -1.000000000000000000 ) ) ;
#59414=EDGE_CURVE ( 'NONE', #28608, #37838, #20701, .T. ) ;
#59421=ORIENTED_EDGE ( 'NONE', *, *, #61939, .F. ) ;
#59422=ORIENTED_EDGE ( 'NONE', *, *, #36445, .F. ) ;
#59424=LINE ( 'NONE', #68610, #23323 ) ;
#59429=CARTESIAN_POINT ( 'NONE',  ( 0.000000000000000000, 0.000000000000000000, 41.38025477438755928 ) ) ;
#59433=ORIENTED_EDGE ( 'NONE', *, *, #63454, .F. ) ;
#59436=CARTESIAN_POINT ( 'NONE',  ( -24.87827947785777383, -3.494138152041991408, 3.061616997868437868E-16 ) ) ;
#59437=LINE ( 'NONE', #27430, #21595 ) ;
#59452=VECTOR ( 'NONE', #61897, 1000.000000000000114 ) ;
#59459=CARTESIAN_POINT ( 'NONE',  ( 36.85262215550070408, 53.56030941157735015, 43.58025477438756923 ) ) ;
#59462=CARTESIAN_POINT ( 'NONE',  ( 62.82395629628391731, 22.24309010993259861, 34.48241795236666007 ) ) ;
#59467=CARTESIAN_POINT ( 'NONE',  ( 0.000000000000000000, 0.000000000000000000, 170.0000000000000000 ) ) ;
#59473=DIRECTION ( 'NONE',  ( 0.000000000000000000, 0.000000000000000000, -1.000000000000000000 ) ) ;
#59475=DIRECTION ( 'NONE',  ( 1.000000000000000000, 0.000000000000000000, 0.000000000000000000 ) ) ;
#59485=AXIS2_PLACEMENT_3D ( 'NONE', #56028, #61645, #1512 ) ;
#59498=DIRECTION ( 'NONE',  ( -0.5128992774058949156, -0.8584487936018728726, 0.000000000000000000 ) ) ;
#59499=DIRECTION ( 'NONE',  ( -0.6910626489868580968, -0.7227948638273978821, 0.000000000000000000 ) ) ;
#59508=CARTESIAN_POINT ( 'NONE',  ( 14.66690460840479027, 20.39656099473415551, 3.061616997868437868E-16 ) ) ;
#59511=ORIENTED_EDGE ( 'NONE', *, *, #28907, .F. ) ;
#59516=DIRECTION ( 'NONE',  ( 0.000000000000000000, 0.000000000000000000, 1.000000000000000000 ) ) ;
#59520=CARTESIAN_POINT ( 'NONE',  ( 0.000000000000000000, 0.000000000000000000, 41.38025477438755928 ) ) ;
#59526=CARTESIAN_POINT ( 'NONE',  ( -1.666933348992581942, 64.97862212458815634, 40.00000000000003553 ) ) ;
#59527=EDGE_CURVE ( 'NONE', #4383, #2042, #37701, .T. ) ;
#59528=CARTESIAN_POINT ( 'NONE',  ( 4.606779575613957789, 24.69646479044443765, 0.000000000000000000 ) ) ;
#59538=ORIENTED_EDGE ( 'NONE', *, *, #43887, .T. ) ;
#59548=VECTOR ( 'NONE', #10696, 1000.000000000000114 ) ;
#59556=DIRECTION ( 'NONE',  ( 1.000000000000000000, 7.105427357601001859E-15, 0.000000000000000000 ) ) ;
#59562=CARTESIAN_POINT ( 'NONE',  ( -50.12142462338810134, -12.53590381416902311, 26.66469104408688651 ) ) ;
#59565=VECTOR ( 'NONE', #5091, 1000.000000000000000 ) ;
#59578=ORIENTED_EDGE ( 'NONE', *, *, #45480, .T. ) ;
#59584=CARTESIAN_POINT ( 'NONE',  ( 31.89651141207616192, -56.63578868294582946, 170.0000000000000000 ) ) ;
#59587=CARTESIAN_POINT ( 'NONE',  ( 0.000000000000000000, 0.000000000000000000, 133.5802547743875550 ) ) ;
#59596=ORIENTED_EDGE ( 'NONE', *, *, #67592, .T. ) ;
#59614=AXIS2_PLACEMENT_3D ( 'NONE', #69440, #46958, #31142 ) ;
#59634=DIRECTION ( 'NONE',  ( -0.000000000000000000, -0.000000000000000000, -1.000000000000000000 ) ) ;
#59643=AXIS2_PLACEMENT_3D ( 'NONE', #27773, #18274, #54846 ) ;
#59645=DIRECTION ( 'NONE',  ( 1.000000000000000000, 0.000000000000000000, 0.000000000000000000 ) ) ;
#59668=CARTESIAN_POINT ( 'NONE',  ( 25.02868068539619628, 33.38981722302369093, 13.79046412397660148 ) ) ;
#59681=DIRECTION ( 'NONE',  ( -1.000000000000000000, 0.000000000000000000, 0.000000000000000000 ) ) ;
#59682=DIRECTION ( 'NONE',  ( 2.201526392813417799E-16, -1.184691869787064686E-16, 1.000000000000000000 ) ) ;
#59687=CARTESIAN_POINT ( 'NONE',  ( -41.50537345350708307, 50.04124777106294886, 41.38025477438755928 ) ) ;
#59698=CARTESIAN_POINT ( 'NONE',  ( 0.000000000000000000, 0.000000000000000000, 170.0000000000000000 ) ) ;
#59714=DIRECTION ( 'NONE',  ( -0.000000000000000000, -0.000000000000000000, -1.000000000000000000 ) ) ;
#59719=EDGE_CURVE ( 'NONE', #28906, #39565, #42145, .T. ) ;
#59720=CARTESIAN_POINT ( 'NONE',  ( -71.90777365577110913, -21.14201501538416395, 41.38025477438755928 ) ) ;
#59721=LINE ( 'NONE', #49511, #17369 ) ;
#59724=ORIENTED_EDGE ( 'NONE', *, *, #28827, .F. ) ;
#59729=CARTESIAN_POINT ( 'NONE',  ( -36.84489839129339828, 53.54860840895182150, 40.00000000000003553 ) ) ;
#59744=AXIS2_PLACEMENT_3D ( 'NONE', #55923, #60495, #18629 ) ;
#59746=FACE_OUTER_BOUND ( 'NONE', #42074, .T. ) ;
#59750=CARTESIAN_POINT ( 'NONE',  ( -59.94154301275508345, -45.09516516490472071, 43.58025477438756923 ) ) ;
#59752=CARTESIAN_POINT ( 'NONE',  ( -63.73419499958998813, 12.83646726144838013, 43.58025477438756923 ) ) ;
#59772=CYLINDRICAL_SURFACE ( 'NONE', #16715, 65.36598343705435354 ) ;
#59777=VERTEX_POINT ( 'NONE', #52753 ) ;
#59780=FACE_OUTER_BOUND ( 'NONE', #5894, .T. ) ;
#59791=CARTESIAN_POINT ( 'NONE',  ( 2.129405171194075130, 25.03204795498856683, 3.061616997868437868E-16 ) ) ;
#59792=VECTOR ( 'NONE', #37475, 999.9999999999998863 ) ;
#59797=DIRECTION ( 'NONE',  ( -1.000000000000000000, 0.000000000000000000, 0.000000000000000000 ) ) ;
#59802=AXIS2_PLACEMENT_3D ( 'NONE', #51638, #41428, #19619 ) ;
#59823=CARTESIAN_POINT ( 'NONE',  ( 60.40479419793764038, 24.00543350795394915, 170.0000000000000000 ) ) ;
#59826=VERTEX_POINT ( 'NONE', #42558 ) ;
#59827=CARTESIAN_POINT ( 'NONE',  ( 9.962235950565768050, -64.23203137738408941, 40.00000000000003553 ) ) ;
#59846=PRODUCT_DEFINITION_CONTEXT ( 'detailed design', #11623, 'design' ) ;
#59849=VERTEX_POINT ( 'NONE', #39031 ) ;
#59850=CARTESIAN_POINT ( 'NONE',  ( 0.000000000000000000, 0.000000000000000000, 41.38025477438755928 ) ) ;
#59854=B_SPLINE_CURVE_WITH_KNOTS ( 'NONE', 3,
 ( #64157, #54638, #6465, #12091, #65560, #49350 ),
 .UNSPECIFIED., .F., .F.,
 ( 4, 2, 4 ),
 ( 0.03218932929355815264, 0.06469831333814429764, 0.09720729738273045650 ),
 .UNSPECIFIED. ) ;
#59855=LINE ( 'NONE', #6407, #25099 ) ;
#59857=CARTESIAN_POINT ( 'NONE',  ( -62.97854483871554976, -16.08424353203763957, 170.0000000000000000 ) ) ;
#59860=CIRCLE ( 'NONE', #9316, 65.00000000000000000 ) ;
#59863=ORIENTED_EDGE ( 'NONE', *, *, #46363, .F. ) ;
#59877=DIRECTION ( 'NONE',  ( -0.000000000000000000, -0.000000000000000000, 1.000000000000000000 ) ) ;
#59878=CARTESIAN_POINT ( 'NONE',  ( 16.62148331457488837, 18.83783649008728744, 0.000000000000000000 ) ) ;
#59881=VERTEX_POINT ( 'NONE', #33753 ) ;
#59886=LINE ( 'NONE', #33179, #18554 ) ;
#59911=ORIENTED_EDGE ( 'NONE', *, *, #11730, .T. ) ;
#59919=CARTESIAN_POINT ( 'NONE',  ( 10.06749493632500503, -74.32123213259498584, 43.58025477438756212 ) ) ;
#59923=VERTEX_POINT ( 'NONE', #52679 ) ;
#59924=EDGE_CURVE ( 'NONE', #6513, #54974, #51191, .T. ) ;
#59925=ORIENTED_EDGE ( 'NONE', *, *, #12069, .F. ) ;
#59926=DIRECTION ( 'NONE',  ( 0.8090169943749422332, 0.5877852522924802425, 0.000000000000000000 ) ) ;
#59938=CARTESIAN_POINT ( 'NONE',  ( -52.73319225379862019, -53.34578647582125654, 170.0000000000000000 ) ) ;
#59939=DIRECTION ( 'NONE',  ( -0.9009688679024218105, 0.4338837391175525693, 0.000000000000000000 ) ) ;
#59949=CARTESIAN_POINT ( 'NONE',  ( -42.36049017605959932, 61.90437280228238137, 170.0000000000000000 ) ) ;
#59951=DIRECTION ( 'NONE',  ( -0.000000000000000000, -0.000000000000000000, -1.000000000000000000 ) ) ;
#59956=ORIENTED_EDGE ( 'NONE', *, *, #30331, .T. ) ;
#59961=ORIENTED_EDGE ( 'NONE', *, *, #46855, .T. ) ;
#59964=DIRECTION ( 'NONE',  ( -1.000000000000000000, 0.000000000000000000, 0.000000000000000000 ) ) ;
#59965=ORIENTED_EDGE ( 'NONE', *, *, #44150, .F. ) ;
#59966=CARTESIAN_POINT ( 'NONE',  ( 0.000000000000000000, 0.000000000000000000, 41.38025477438755928 ) ) ;
#59973=ORIENTED_EDGE ( 'NONE', *, *, #49305, .T. ) ;
#59985=CARTESIAN_POINT ( 'NONE',  ( 39.54205320694339321, 51.58901073076764021, 40.00000000000003553 ) ) ;
#59991=AXIS2_PLACEMENT_3D ( 'NONE', #46239, #5317, #14920 ) ;
#59999=DIRECTION ( 'NONE',  ( 0.1342332658176522697, 0.9909497617679352555, 0.000000000000000000 ) ) ;
#60000=CARTESIAN_POINT ( 'NONE',  ( 0.000000000000000000, 0.000000000000000000, 40.00000000000003553 ) ) ;
#60003=DIRECTION ( 'NONE',  ( -0.000000000000000000, -0.000000000000000000, -1.000000000000000000 ) ) ;
#60005=AXIS2_PLACEMENT_3D ( 'NONE', #4575, #26040, #47471 ) ;
#60008=ORIENTED_EDGE ( 'NONE', *, *, #38854, .T. ) ;
#60009=VECTOR ( 'NONE', #52198, 999.9999999999998863 ) ;
#60013=DIRECTION ( 'NONE',  ( -1.000000000000000000, 0.000000000000000000, 0.000000000000000000 ) ) ;
#60021=CARTESIAN_POINT ( 'NONE',  ( -19.15041341282721632, 47.98507848106410734, 26.66469104408690072 ) ) ;
#60025=EDGE_LOOP ( 'NONE', ( #41156, #63122, #21792, #19676 ) ) ;
#60031=CARTESIAN_POINT ( 'NONE',  ( 39.71871809564405709, -33.04132994422423764, 26.66469066592269854 ) ) ;
#60038=EDGE_CURVE ( 'NONE', #3538, #52894, #28026, .T. ) ;
#60053=VECTOR ( 'NONE', #58553, 1000.000000000000000 ) ;
#60059=ORIENTED_EDGE ( 'NONE', *, *, #61052, .T. ) ;
#60060=VERTEX_POINT ( 'NONE', #33327 ) ;
#60068=LINE ( 'NONE', #54795, #30608 ) ;
#60073=ADVANCED_FACE ( 'NONE', ( #28377 ), #12916, .F. ) ;
#60079=ORIENTED_EDGE ( 'NONE', *, *, #34403, .T. ) ;
#60093=CIRCLE ( 'NONE', #9606, 65.36598343705435354 ) ;
#60102=ADVANCED_FACE ( 'NONE', ( #55455 ), #61089, .T. ) ;
#60106=CARTESIAN_POINT ( 'NONE',  ( -63.73419499958998813, 12.83646726144834993, 170.0000000000000000 ) ) ;
#60108=ORIENTED_EDGE ( 'NONE', *, *, #68466, .T. ) ;
#60111=ORIENTED_EDGE ( 'NONE', *, *, #62722, .T. ) ;
#60118=VECTOR ( 'NONE', #45739, 1000.000000000000114 ) ;
#60120=B_SPLINE_CURVE_WITH_KNOTS ( 'NONE', 3,
 ( #9524, #20412, #26394, #47142 ),
 .UNSPECIFIED., .F., .F.,
 ( 4, 4 ),
 ( 0.1259919275528359750, 0.1829744153748750768 ),
 .UNSPECIFIED. ) ;
#60124=ADVANCED_FACE ( 'NONE', ( #18528 ), #34716, .F. ) ;
#60127=FACE_OUTER_BOUND ( 'NONE', #28066, .T. ) ;
#60129=CARTESIAN_POINT ( 'NONE',  ( 70.65683382808195745, 25.18281821780106711, 170.0000000000000000 ) ) ;
#60134=PLANE ( 'NONE',  #54927 ) ;
#60135=FACE_OUTER_BOUND ( 'NONE', #30742, .T. ) ;
#60138=ORIENTED_EDGE ( 'NONE', *, *, #44777, .T. ) ;
#60141=CARTESIAN_POINT ( 'NONE',  ( 12.99074365121421692, 21.50298515537768296, 0.000000000000000000 ) ) ;
#60144=CARTESIAN_POINT ( 'NONE',  ( -36.53690438256411710, 73.43472186181504924, 73.58025477438756923 ) ) ;
#60145=ORIENTED_EDGE ( 'NONE', *, *, #62889, .T. ) ;
#60152=VECTOR ( 'NONE', #5932, 1000.000000000000000 ) ;
#60155=CARTESIAN_POINT ( 'NONE',  ( 5.694488332793534724, 51.35054872415687299, 26.66469066592269499 ) ) ;
#60159=DIRECTION ( 'NONE',  ( -0.000000000000000000, 0.000000000000000000, -1.000000000000000000 ) ) ;
#60163=VECTOR ( 'NONE', #57345, 1000.000000000000000 ) ;
#60165=CARTESIAN_POINT ( 'NONE',  ( -68.11501976657858393, 31.41506934893840963, 43.58025477438756923 ) ) ;
#60177=CARTESIAN_POINT ( 'NONE',  ( 15.68296563925591514, -63.09411298019745828, 43.58025477438756923 ) ) ;
#60187=ORIENTED_EDGE ( 'NONE', *, *, #15500, .T. ) ;
#60191=ADVANCED_FACE ( 'NONE', ( #20939 ), #63508, .T. ) ;
#60194=PLANE ( 'NONE',  #58210 ) ;
#60195=DIRECTION ( 'NONE',  ( -0.000000000000000000, -0.000000000000000000, -1.000000000000000000 ) ) ;
#60197=DIRECTION ( 'NONE',  ( 0.9839295885986295565, 0.1785568947986370392, 0.000000000000000000 ) ) ;
#60201=ORIENTED_EDGE ( 'NONE', *, *, #56446, .T. ) ;
#60204=CARTESIAN_POINT ( 'NONE',  ( 46.76173513940573656, -58.63736118510165340, 43.58025477438756212 ) ) ;
#60210=VERTEX_POINT ( 'NONE', #64189 ) ;
#60213=AXIS2_PLACEMENT_3D ( 'NONE', #16700, #10382, #37817 ) ;
#60222=EDGE_CURVE ( 'NONE', #55351, #44519, #872, .T. ) ;
#60225=CIRCLE ( 'NONE', #47862, 65.00000000000000000 ) ;
#60229=DIRECTION ( 'NONE',  ( -0.4738686624729966379, -0.8805955318567391110, 0.000000000000000000 ) ) ;
#60233=CARTESIAN_POINT ( 'NONE',  ( 37.92109554537579896, -5.611248133931618476, 13.32819299319724493 ) ) ;
#60238=ORIENTED_EDGE ( 'NONE', *, *, #42196, .F. ) ;
#60240=CARTESIAN_POINT ( 'NONE',  ( -27.75784438064426141, -18.62216945641829469, 6.893343212288923993 ) ) ;
#60242=ORIENTED_EDGE ( 'NONE', *, *, #6049, .F. ) ;
#60249=LINE ( 'NONE', #1161, #51152 ) ;
#60264=AXIS2_PLACEMENT_3D ( 'NONE', #24521, #30140, #14302 ) ;
#60266=DIRECTION ( 'NONE',  ( 1.000000000000000000, 0.000000000000000000, 0.000000000000000000 ) ) ;
#60267=CARTESIAN_POINT ( 'NONE',  ( -13.32397999418070178, 63.99361958670517225, 43.58025477438756212 ) ) ;
#60271=VECTOR ( 'NONE', #4828, 1000.000000000000000 ) ;
#60280=EDGE_CURVE ( 'NONE', #6453, #31099, #1782, .T. ) ;
#60281=ORIENTED_EDGE ( 'NONE', *, *, #66197, .T. ) ;
#60300=DIRECTION ( 'NONE',  ( -0.000000000000000000, -0.000000000000000000, -1.000000000000000000 ) ) ;
#60307=CARTESIAN_POINT ( 'NONE',  ( 0.000000000000000000, 0.000000000000000000, 0.000000000000000000 ) ) ;
#60309=VERTEX_POINT ( 'NONE', #16000 ) ;
#60310=AXIS2_PLACEMENT_3D ( 'NONE', #36514, #9786, #63595 ) ;
#60323=VECTOR ( 'NONE', #68484, 1000.000000000000000 ) ;
#60327=ORIENTED_EDGE ( 'NONE', *, *, #11199, .T. ) ;
#60341=DIRECTION ( 'NONE',  ( -0.000000000000000000, -0.000000000000000000, -1.000000000000000000 ) ) ;
#60342=CARTESIAN_POINT ( 'NONE',  ( 21.98745393275193294, 71.71550996510526943, 170.0000000000000000 ) ) ;
#60345=EDGE_CURVE ( 'NONE', #42019, #6204, #58227, .T. ) ;
#60349=LINE ( 'NONE', #59295, #59154 ) ;
#60354=PLANE ( 'NONE',  #40995 ) ;
#60357=DIRECTION ( 'NONE',  ( 1.000000000000000000, 0.000000000000000000, 0.000000000000000000 ) ) ;
#60360=ADVANCED_FACE ( 'NONE', ( #32529 ), #38147, .F. ) ;
#60361=ORIENTED_EDGE ( 'NONE', *, *, #31364, .F. ) ;
#60364=EDGE_CURVE ( 'NONE', #42365, #68939, #15321, .T. ) ;
#60372=CIRCLE ( 'NONE', #57018, 63.00000000000000000 ) ;
#60375=CARTESIAN_POINT ( 'NONE',  ( 10.01137213834968165, -64.59476928204590251, 43.58025477438756212 ) ) ;
#60376=ORIENTED_EDGE ( 'NONE', *, *, #42701, .T. ) ;
#60389=LINE ( 'NONE', #23464, #48790 ) ;
#60391=DIRECTION ( 'NONE',  ( -0.000000000000000000, -0.000000000000000000, -1.000000000000000000 ) ) ;
#60394=DIRECTION ( 'NONE',  ( -0.000000000000000000, 0.000000000000000000, -1.000000000000000000 ) ) ;
#60399=CARTESIAN_POINT ( 'NONE',  ( -44.26023579658871654, -48.10138582123836670, 3.125053320693551875E-16 ) ) ;
#60411=DIRECTION ( 'NONE',  ( 0.9839295885986295565, 0.1785568947986370392, 0.000000000000000000 ) ) ;
#60417=VECTOR ( 'NONE', #61036, 1000.000000000000227 ) ;
#60419=VERTEX_POINT ( 'NONE', #39897 ) ;
#60421=EDGE_CURVE ( 'NONE', #36461, #4465, #19749, .T. ) ;
#60426=ADVANCED_FACE ( 'NONE', ( #45166 ), #50456, .T. ) ;
#60429=ORIENTED_EDGE ( 'NONE', *, *, #871, .F. ) ;
#60430=DIRECTION ( 'NONE',  ( -1.000000000000000000, 0.000000000000000000, 0.000000000000000000 ) ) ;
#60431=ADVANCED_FACE ( 'NONE', ( #50793 ), #23027, .F. ) ;
#60432=PLANE ( 'NONE',  #45170 ) ;
#60435=CARTESIAN_POINT ( 'NONE',  ( -63.89980896331448434, -18.93195718737547750, 34.48241823982459664 ) ) ;
#60446=LINE ( 'NONE', #39685, #12218 ) ;
#60469=DIRECTION ( 'NONE',  ( 0.9909497617679352555, -0.1342332658176522697, 5.102127870520022769E-18 ) ) ;
#60473=ORIENTED_EDGE ( 'NONE', *, *, #49395, .F. ) ;
#60479=ORIENTED_EDGE ( 'NONE', *, *, #30665, .T. ) ;
#60483=CARTESIAN_POINT ( 'NONE',  ( -23.14886993799567705, -9.760512885997105315, 0.000000000000000000 ) ) ;
#60485=EDGE_CURVE ( 'NONE', #52661, #43797, #18443, .T. ) ;
#60487=DIRECTION ( 'NONE',  ( 0.000000000000000000, 0.000000000000000000, 1.000000000000000000 ) ) ;
#60488=CARTESIAN_POINT ( 'NONE',  ( -72.62976060914745347, 18.74780984163036024, 170.0000000000000000 ) ) ;
#60495=DIRECTION ( 'NONE',  ( -0.000000000000000000, -0.000000000000000000, 1.000000000000000000 ) ) ;
#60498=LINE ( 'NONE', #33434, #41958 ) ;
#60499=ORIENTED_EDGE ( 'NONE', *, *, #15034, .F. ) ;
#60500=ADVANCED_FACE ( 'NONE', ( #6839 ), #61354, .T. ) ;
#60525=ORIENTED_EDGE ( 'NONE', *, *, #24760, .F. ) ;
#60526=ADVANCED_FACE ( 'NONE', ( #44111 ), #43377, .T. ) ;
#60529=EDGE_CURVE ( 'NONE', #6992, #40870, #46903, .T. ) ;
#60533=LINE ( 'NONE', #19260, #54787 ) ;
#60558=LINE ( 'NONE', #66215, #411 ) ;
#60559=VECTOR ( 'NONE', #42427, 1000.000000000000000 ) ;
#60577=LINE ( 'NONE', #55293, #23986 ) ;
#60578=CONICAL_SURFACE ( 'NONE', #42645, 65.00000000000000000, 0.7853981633974497223 ) ;
#60583=CARTESIAN_POINT ( 'NONE',  ( -58.33959211651038146, 29.48226216511319464, 41.38025477438755928 ) ) ;
#60585=EDGE_CURVE ( 'NONE', #59881, #4077, #68026, .T. ) ;
#60588=DIRECTION ( 'NONE',  ( 1.000000000000000000, 0.000000000000000000, 0.000000000000000000 ) ) ;
#60594=LINE ( 'NONE', #23325, #41983 ) ;
#60595=VECTOR ( 'NONE', #52981, 999.9999999999998863 ) ;
#60607=CARTESIAN_POINT ( 'NONE',  ( 64.08056813503694116, 12.89932471814516290, 43.58025477438756212 ) ) ;
#60608=ORIENTED_EDGE ( 'NONE', *, *, #32463, .F. ) ;
#60610=EDGE_CURVE ( 'NONE', #24540, #20416, #61376, .T. ) ;
#60618=EDGE_CURVE ( 'NONE', #67945, #13204, #21538, .T. ) ;
#60623=VERTEX_POINT ( 'NONE', #42315 ) ;
#60624=CARTESIAN_POINT ( 'NONE',  ( -21.27554331372908081, -61.43430442924895374, 170.0000000000000000 ) ) ;
#60628=DIRECTION ( 'NONE',  ( -0.8090169943749507819, 0.5877852522924685852, 0.000000000000000000 ) ) ;
#60631=CARTESIAN_POINT ( 'NONE',  ( 73.95984195137799588, -12.15131637179793955, 41.38025477438755928 ) ) ;
#60632=DIRECTION ( 'NONE',  ( 0.3930250316539278255, -0.9195277725514487965, 0.000000000000000000 ) ) ;
#60635=ORIENTED_EDGE ( 'NONE', *, *, #34347, .T. ) ;
#60644=CARTESIAN_POINT ( 'NONE',  ( 0.000000000000000000, 0.000000000000000000, 41.38025477438755928 ) ) ;
#60653=CARTESIAN_POINT ( 'NONE',  ( 21.96921518829288900, -71.65937688154161833, 41.38025477438755928 ) ) ;
#60654=DIRECTION ( 'NONE',  ( -0.000000000000000000, -0.000000000000000000, -1.000000000000000000 ) ) ;
#60660=DIRECTION ( 'NONE',  ( -0.000000000000000000, 0.000000000000000000, -1.000000000000000000 ) ) ;
#60667=EDGE_CURVE ( 'NONE', #36599, #34263, #4095, .T. ) ;
#60669=VERTEX_POINT ( 'NONE', #11326 ) ;
#60682=LINE ( 'NONE', #65982, #55076 ) ;
#60689=FACE_OUTER_BOUND ( 'NONE', #43650, .T. ) ;
#60704=CARTESIAN_POINT ( 'NONE',  ( 73.57152302639913444, -14.62167909564502821, 43.58025477438756212 ) ) ;
#60718=ORIENTED_EDGE ( 'NONE', *, *, #716, .T. ) ;
#60728=CARTESIAN_POINT ( 'NONE',  ( 61.91366885787816443, -28.42865614898931881, 43.58025477438756923 ) ) ;
#60729=CARTESIAN_POINT ( 'NONE',  ( -4.164416015345870470, 64.86646004871185767, 170.0000000000000000 ) ) ;
#60741=AXIS2_PLACEMENT_3D ( 'NONE', #2085, #23538, #55888 ) ;
#60742=CARTESIAN_POINT ( 'NONE',  ( 35.16506403794528524, -22.46626249432251399, 13.79046340968178264 ) ) ;
#60749=LINE ( 'NONE', #6236, #30764 ) ;
#60760=CARTESIAN_POINT ( 'NONE',  ( 1.667562369266826661, 64.99262834925669097, 41.38025477438755928 ) ) ;
#60763=EDGE_LOOP ( 'NONE', ( #13309, #63714, #61151, #68456 ) ) ;
#60781=ORIENTED_EDGE ( 'NONE', *, *, #68893, .F. ) ;
#60789=CARTESIAN_POINT ( 'NONE',  ( 64.98797965777978902, -1.250000000000021094, 170.0000000000000000 ) ) ;
#60798=LINE ( 'NONE', #66804, #54574 ) ;
#60810=DIRECTION ( 'NONE',  ( 0.9195277725514489076, 0.3930250316539278810, -0.000000000000000000 ) ) ;
#60811=CARTESIAN_POINT ( 'NONE',  ( -84.49322488516129681, 0.000000000000000000, 43.58025477438756212 ) ) ;
#60821=ADVANCED_FACE ( 'NONE', ( #69215 ), #46378, .T. ) ;
#60826=DIRECTION ( 'NONE',  ( -0.7530714660036099684, -0.6579387259397136978, 0.000000000000000000 ) ) ;
#60834=AXIS2_PLACEMENT_3D ( 'NONE', #26300, #65942, #65578 ) ;
#60835=ORIENTED_EDGE ( 'NONE', *, *, #19522, .F. ) ;
#60836=EDGE_CURVE ( 'NONE', #40116, #41223, #21040, .T. ) ;
#60838=ORIENTED_EDGE ( 'NONE', *, *, #38118, .F. ) ;
#60840=CARTESIAN_POINT ( 'NONE',  ( 0.000000000000000000, 0.000000000000000000, 41.38025477438755928 ) ) ;
#60841=DIRECTION ( 'NONE',  ( -1.000000000000000000, 0.000000000000000000, 0.000000000000000000 ) ) ;
#60848=ORIENTED_EDGE ( 'NONE', *, *, #8483, .F. ) ;
#60863=VERTEX_POINT ( 'NONE', #8774 ) ;
#60866=ORIENTED_EDGE ( 'NONE', *, *, #5150, .F. ) ;
#60878=AXIS2_PLACEMENT_3D ( 'NONE', #9928, #62707, #42277 ) ;
#60880=AXIS2_PLACEMENT_3D ( 'NONE', #17564, #27763, #22142 ) ;
#60887=CONICAL_SURFACE ( 'NONE', #9223, 74.95140232871122521, 0.8777644062502172329 ) ;
#60896=ORIENTED_EDGE ( 'NONE', *, *, #55044, .F. ) ;
#60899=EDGE_CURVE ( 'NONE', #9934, #18701, #46730, .T. ) ;
#60907=ORIENTED_EDGE ( 'NONE', *, *, #48949, .F. ) ;
#60914=ADVANCED_BREP_SHAPE_REPRESENTATION ( '', ( #18268, #66832 ), #2840 ) ;
#60916=B_SPLINE_CURVE_WITH_KNOTS ( 'NONE', 3,
 ( #58520, #3348, #24808, #46243, #62785, #20212 ),
 .UNSPECIFIED., .F., .F.,
 ( 4, 2, 4 ),
 ( 1.095770181118598899E-06, 0.03239442681617712289, 0.06478775786217312593 ),
 .UNSPECIFIED. ) ;
#60918=CARTESIAN_POINT ( 'NONE',  ( 0.000000000000000000, 0.000000000000000000, 41.38025477438755928 ) ) ;
#60921=DIRECTION ( 'NONE',  ( 1.000000000000000000, 7.993605777301127091E-15, 0.000000000000000000 ) ) ;
#60925=EDGE_CURVE ( 'NONE', #45135, #28312, #14182, .T. ) ;
#60928=ORIENTED_EDGE ( 'NONE', *, *, #41241, .F. ) ;
#60929=DIRECTION ( 'NONE',  ( -0.000000000000000000, 0.000000000000000000, -1.000000000000000000 ) ) ;
#60936=CARTESIAN_POINT ( 'NONE',  ( -34.47910271558636452, -23.50544947846431043, 13.79046340968177020 ) ) ;
#60956=VERTEX_POINT ( 'NONE', #38243 ) ;
#60965=DIRECTION ( 'NONE',  ( -1.000000000000000000, 0.000000000000000000, 0.000000000000000000 ) ) ;
#60967=EDGE_CURVE ( 'NONE', #47893, #48012, #38959, .T. ) ;
#60976=CIRCLE ( 'NONE', #62131, 25.12245591505646303 ) ;
#60981=EDGE_CURVE ( 'NONE', #34764, #41788, #56165, .T. ) ;
#60984=CIRCLE ( 'NONE', #29505, 74.95140232871122521 ) ;
#60988=CARTESIAN_POINT ( 'NONE',  ( -36.59702023225411693, 36.46867370448659784, 26.66469066592269144 ) ) ;
#60993=EDGE_CURVE ( 'NONE', #52661, #12758, #56505, .T. ) ;
#61001=CARTESIAN_POINT ( 'NONE',  ( 4.590321433069001422, -24.57496590315233931, 0.000000000000000000 ) ) ;
#61008=ORIENTED_EDGE ( 'NONE', *, *, #52551, .T. ) ;
#61009=DIRECTION ( 'NONE',  ( 0.04486483035050447404, 0.9989930665413151445, -0.000000000000000000 ) ) ;
#61019=ORIENTED_EDGE ( 'NONE', *, *, #2875, .T. ) ;
#61028=VECTOR ( 'NONE', #65650, 1000.000000000000000 ) ;
#61036=DIRECTION ( 'NONE',  ( -0.2225209339563184452, 0.9749279121818226201, 5.146830507070804164E-17 ) ) ;
#61041=ORIENTED_EDGE ( 'NONE', *, *, #31048, .T. ) ;
#61047=DIRECTION ( 'NONE',  ( 0.000000000000000000, 0.000000000000000000, 1.000000000000000000 ) ) ;
#61048=DIRECTION ( 'NONE',  ( -1.000000000000000000, 0.000000000000000000, 0.000000000000000000 ) ) ;
#61052=EDGE_CURVE ( 'NONE', #23096, #13308, #11962, .T. ) ;
#61054=ORIENTED_EDGE ( 'NONE', *, *, #4456, .F. ) ;
#61058=CARTESIAN_POINT ( 'NONE',  ( -72.62976060914719767, -18.74780984163136566, 170.0000000000000000 ) ) ;
#61059=DIRECTION ( 'NONE',  ( -0.000000000000000000, -0.000000000000000000, 1.000000000000000000 ) ) ;
#61060=CARTESIAN_POINT ( 'NONE',  ( -24.53636015449790264, 60.58612729876396941, 6.377659838150179840E-18 ) ) ;
#61061=DIRECTION ( 'NONE',  ( -1.000000000000000000, 0.000000000000000000, 0.000000000000000000 ) ) ;
#61066=EDGE_CURVE ( 'NONE', #9408, #58973, #65864, .T. ) ;
#61076=EDGE_CURVE ( 'NONE', #5356, #15020, #40673, .T. ) ;
#61077=DIRECTION ( 'NONE',  ( -0.000000000000000000, 0.000000000000000000, -1.000000000000000000 ) ) ;
#61088=AXIS2_PLACEMENT_3D ( 'NONE', #31402, #41950, #26117 ) ;
#61089=CYLINDRICAL_SURFACE ( 'NONE', #6276, 65.00000000000000000 ) ;
#61091=VECTOR ( 'NONE', #8154, 1000.000000000000000 ) ;
#61093=AXIS2_PLACEMENT_3D ( 'NONE', #10298, #11335, #10994 ) ;
#61097=CYLINDRICAL_SURFACE ( 'NONE', #11604, 65.36598343705435354 ) ;
#61108=DIRECTION ( 'NONE',  ( 1.000000000000000000, 0.000000000000000000, 0.000000000000000000 ) ) ;
#61109=ORIENTED_EDGE ( 'NONE', *, *, #46122, .T. ) ;
#61112=DIRECTION ( 'NONE',  ( 1.000000000000000000, 0.000000000000000000, 0.000000000000000000 ) ) ;
#61117=VERTEX_POINT ( 'NONE', #21978 ) ;
#61128=AXIS2_PLACEMENT_3D ( 'NONE', #60811, #29162, #50612 ) ;
#61132=ADVANCED_FACE ( 'NONE', ( #5112 ), #54320, .F. ) ;
#61139=DIRECTION ( 'NONE',  ( 0.000000000000000000, 0.000000000000000000, 1.000000000000000000 ) ) ;
#61141=ORIENTED_EDGE ( 'NONE', *, *, #34429, .F. ) ;
#61142=ORIENTED_EDGE ( 'NONE', *, *, #65288, .F. ) ;
#61148=CARTESIAN_POINT ( 'NONE',  ( 43.10136218933562446, -39.31639513875150982, 27.58472315868180402 ) ) ;
#61150=EDGE_CURVE ( 'NONE', #32488, #9160, #42740, .T. ) ;
#61151=ORIENTED_EDGE ( 'NONE', *, *, #56333, .T. ) ;
#61153=VERTEX_POINT ( 'NONE', #53967 ) ;
#61163=CARTESIAN_POINT ( 'NONE',  ( 73.57152302639893549, 14.62167909564604429, 170.0000000000000000 ) ) ;
#61164=CARTESIAN_POINT ( 'NONE',  ( 47.73902449248994628, 57.85799893277891215, 170.0000000000000000 ) ) ;
#61166=FACE_OUTER_BOUND ( 'NONE', #34894, .T. ) ;
#61168=ORIENTED_EDGE ( 'NONE', *, *, #26104, .T. ) ;
#61173=DIRECTION ( 'NONE',  ( 0.6910626489868685329, -0.7227948638273878901, 0.000000000000000000 ) ) ;
#61185=PLANE ( 'NONE',  #40878 ) ;
#61190=AXIS2_PLACEMENT_3D ( 'NONE', #41400, #14654, #4109 ) ;
#61191=LINE ( 'NONE', #60488, #23680 ) ;
#61197=DIRECTION ( 'NONE',  ( 0.9362348706397417564, -0.3513748240813305279, 0.000000000000000000 ) ) ;
#61203=VERTEX_POINT ( 'NONE', #12135 ) ;
#61211=EDGE_CURVE ( 'NONE', #14663, #17465, #28302, .T. ) ;
#61216=CARTESIAN_POINT ( 'NONE',  ( 74.62299871641508275, -5.461138973197949831, 170.0000000000000000 ) ) ;
#61218=EDGE_CURVE ( 'NONE', #64743, #10732, #8565, .T. ) ;
#61222=ORIENTED_EDGE ( 'NONE', *, *, #24163, .F. ) ;
#61223=CARTESIAN_POINT ( 'NONE',  ( -15.67984581960975632, -63.08044415722883969, 40.00000000000003553 ) ) ;
#61231=VECTOR ( 'NONE', #14962, 1000.000000000000000 ) ;
#61241=CARTESIAN_POINT ( 'NONE',  ( -12.77952633087691403, 21.62918162951106993, 0.000000000000000000 ) ) ;
#61243=ORIENTED_EDGE ( 'NONE', *, *, #25435, .T. ) ;
#61248=DIRECTION ( 'NONE',  ( -0.9989930665413143673, -0.04486483035051862939, 0.000000000000000000 ) ) ;
#61249=PLANE ( 'NONE',  #45717 ) ;
#61250=CARTESIAN_POINT ( 'NONE',  ( 61.94551923608091926, -24.58367728653112039, 34.48241795236666718 ) ) ;
#61257=DIRECTION ( 'NONE',  ( 1.000000000000000000, 0.000000000000000000, 0.000000000000000000 ) ) ;
#61262=VERTEX_POINT ( 'NONE', #66657 ) ;
#61269=VECTOR ( 'NONE', #20802, 1000.000000000000227 ) ;
#61271=DIRECTION ( 'NONE',  ( -0.000000000000000000, -0.000000000000000000, -1.000000000000000000 ) ) ;
#61284=EDGE_LOOP ( 'NONE', ( #36811, #46695, #8535, #55483 ) ) ;
#61285=DIRECTION ( 'NONE',  ( 0.000000000000000000, 0.000000000000000000, -1.000000000000000000 ) ) ;
#61296=ORIENTED_EDGE ( 'NONE', *, *, #34141, .F. ) ;
#61299=DIRECTION ( 'NONE',  ( -0.000000000000000000, -0.000000000000000000, -1.000000000000000000 ) ) ;
#61304=CARTESIAN_POINT ( 'NONE',  ( 70.21761529798065737, -26.35311180609978976, 43.58025477438756212 ) ) ;
#61307=EDGE_CURVE ( 'NONE', #36964, #39147, #40255, .T. ) ;
#61318=EDGE_LOOP ( 'NONE', ( #27004, #29040, #32042, #21711 ) ) ;
#61323=EDGE_CURVE ( 'NONE', #48110, #14951, #23400, .T. ) ;
#61324=DIRECTION ( 'NONE',  ( 1.000000000000000000, 0.000000000000000000, 0.000000000000000000 ) ) ;
#61328=VECTOR ( 'NONE', #6498, 1000.000000000000114 ) ;
#61329=VECTOR ( 'NONE', #43686, 999.9999999999998863 ) ;
#61331=CARTESIAN_POINT ( 'NONE',  ( -26.83517958587657404, 59.60356471962912650, 3.125053320693570118E-16 ) ) ;
#61344=DIRECTION ( 'NONE',  ( -0.000000000000000000, -0.000000000000000000, -1.000000000000000000 ) ) ;
#61345=ORIENTED_EDGE ( 'NONE', *, *, #40726, .T. ) ;
#61347=CARTESIAN_POINT ( 'NONE',  ( -74.58602291351357394, -7.967916035252126328, 43.58025477438756923 ) ) ;
#61354=CYLINDRICAL_SURFACE ( 'NONE', #2937, 65.36598343705435354 ) ;
#61359=CARTESIAN_POINT ( 'NONE',  ( 0.000000000000000000, 0.000000000000000000, 40.00000000000003553 ) ) ;
#61360=CARTESIAN_POINT ( 'NONE',  ( -9.291678301352696678, 76.94361032721405991, 133.5802547743875550 ) ) ;
#61364=ORIENTED_EDGE ( 'NONE', *, *, #30355, .T. ) ;
#61367=DIRECTION ( 'NONE',  ( -1.000000000000000000, 0.000000000000000000, 0.000000000000000000 ) ) ;
#61372=AXIS2_PLACEMENT_3D ( 'NONE', #24328, #19032, #7795 ) ;
#61376=CIRCLE ( 'NONE', #35521, 65.00000000000000000 ) ;
#61382=EDGE_CURVE ( 'NONE', #33141, #30832, #2620, .T. ) ;
#61383=CARTESIAN_POINT ( 'NONE',  ( 18.89356949897907967, -62.19351277735683681, 40.00000000000003553 ) ) ;
#61384=AXIS2_PLACEMENT_3D ( 'NONE', #31560, #9423, #64258 ) ;
#61398=CARTESIAN_POINT ( 'NONE',  ( -41.50537345350635121, -50.04124777106355282, 43.58025477438756923 ) ) ;
#61402=VERTEX_POINT ( 'NONE', #9634 ) ;
#61417=ORIENTED_EDGE ( 'NONE', *, *, #20577, .T. ) ;
#61419=CONICAL_SURFACE ( 'NONE', #24369, 74.95140232871122521, 0.8777644062502172329 ) ;
#61420=LINE ( 'NONE', #29410, #67816 ) ;
#61422=CARTESIAN_POINT ( 'NONE',  ( 15.68296563925591869, -63.09411298019745828, 0.000000000000000000 ) ) ;
#61433=VECTOR ( 'NONE', #12885, 1000.000000000000000 ) ;
#61449=ORIENTED_EDGE ( 'NONE', *, *, #2073, .T. ) ;
#61455=VERTEX_POINT ( 'NONE', #30741 ) ;
#61459=CARTESIAN_POINT ( 'NONE',  ( -84.49322488516129681, 0.000000000000000000, 43.58025477438756212 ) ) ;
#61461=DIRECTION ( 'NONE',  ( 0.000000000000000000, 0.000000000000000000, 1.000000000000000000 ) ) ;
#61473=EDGE_CURVE ( 'NONE', #60060, #69323, #67691, .T. ) ;
#61476=ORIENTED_EDGE ( 'NONE', *, *, #22732, .T. ) ;
#61480=CIRCLE ( 'NONE', #28899, 24.99999999999985434 ) ;
#61485=CARTESIAN_POINT ( 'NONE',  ( 0.000000000000000000, 0.000000000000000000, 0.000000000000000000 ) ) ;
#61490=ORIENTED_EDGE ( 'NONE', *, *, #19462, .T. ) ;
#61493=EDGE_CURVE ( 'NONE', #1734, #58973, #9278, .T. ) ;
#61499=LINE ( 'NONE', #57259, #23892 ) ;
#61503=ORIENTED_EDGE ( 'NONE', *, *, #20577, .F. ) ;
#61504=DIRECTION ( 'NONE',  ( -0.000000000000000000, -0.000000000000000000, -1.000000000000000000 ) ) ;
#61509=CARTESIAN_POINT ( 'NONE',  ( -4.613603609464500543, -74.86839895266049894, 43.58025477438756212 ) ) ;
#61526=VECTOR ( 'NONE', #67346, 1000.000000000000114 ) ;
#61546=ORIENTED_EDGE ( 'NONE', *, *, #45250, .T. ) ;
#61560=LINE ( 'NONE', #7756, #7003 ) ;
#61571=CARTESIAN_POINT ( 'NONE',  ( 24.34685647903079442, -70.88683439560421107, 41.38025477438755928 ) ) ;
#61572=ORIENTED_EDGE ( 'NONE', *, *, #60585, .T. ) ;
#61574=CIRCLE ( 'NONE', #38003, 65.36598343705435354 ) ;
#61578=AXIS2_PLACEMENT_3D ( 'NONE', #16897, #11617, #33089 ) ;
#61583=EDGE_CURVE ( 'NONE', #11134, #67683, #7819, .T. ) ;
#61596=CARTESIAN_POINT ( 'NONE',  ( 38.61145306061725080, -15.82625577337686629, 13.79046340968177731 ) ) ;
#61603=PLANE ( 'NONE',  #11958 ) ;
#61618=ORIENTED_EDGE ( 'NONE', *, *, #64852, .F. ) ;
#61620=CARTESIAN_POINT ( 'NONE',  ( 65.02478361689782105, -37.39438481343979959, 170.0000000000000000 ) ) ;
#61622=CARTESIAN_POINT ( 'NONE',  ( -65.00000000000000000, 0.000000000000000000, 170.0000000000000000 ) ) ;
#61630=CARTESIAN_POINT ( 'NONE',  ( 18.89356949897907967, -62.19351277735683681, 170.0000000000000000 ) ) ;
#61633=CARTESIAN_POINT ( 'NONE',  ( -21.03405120204953960, -13.73704776265678440, 0.000000000000000000 ) ) ;
#61637=EDGE_CURVE ( 'NONE', #41626, #36843, #50178, .T. ) ;
#61643=LINE ( 'NONE', #12767, #46912 ) ;
#61645=DIRECTION ( 'NONE',  ( -0.000000000000000000, -0.000000000000000000, -1.000000000000000000 ) ) ;
#61662=ORIENTED_EDGE ( 'NONE', *, *, #40527, .F. ) ;
#61665=ORIENTED_EDGE ( 'NONE', *, *, #24634, .F. ) ;
#61666=AXIS2_PLACEMENT_3D ( 'NONE', #17405, #48697, #38517 ) ;
#61698=EDGE_CURVE ( 'NONE', #26839, #40972, #66766, .T. ) ;
#61704=CARTESIAN_POINT ( 'NONE',  ( -12.71191147681863143, 50.07707417820910933, 26.66469066592269499 ) ) ;
#61705=DIRECTION ( 'NONE',  ( -0.3930250316539278255, 0.9195277725514487965, 0.000000000000000000 ) ) ;
#61710=CARTESIAN_POINT ( 'NONE',  ( 41.49663191311347532, 50.03028622612080767, 170.0000000000000000 ) ) ;
#61726=LINE ( 'NONE', #13552, #65811 ) ;
#61729=VECTOR ( 'NONE', #61814, 1000.000000000000114 ) ;
#61732=DIRECTION ( 'NONE',  ( -0.3930250316539148359, -0.9195277725514544587, 0.000000000000000000 ) ) ;
#61737=CARTESIAN_POINT ( 'NONE',  ( 0.000000000000000000, 0.000000000000000000, 41.38025477438755928 ) ) ;
#61741=CARTESIAN_POINT ( 'NONE',  ( -65.00200000000002376, 1.250000000000011102, 43.58025477438756923 ) ) ;
#61750=ORIENTED_EDGE ( 'NONE', *, *, #57972, .T. ) ;
#61758=CARTESIAN_POINT ( 'NONE',  ( -29.70166638324964126, 57.83280658984259048, 41.38025477438755928 ) ) ;
#61775=AXIS2_PLACEMENT_3D ( 'NONE', #10595, #64415, #11285 ) ;
#61776=LINE ( 'NONE', #4089, #50944 ) ;
#61778=CARTESIAN_POINT ( 'NONE',  ( -63.00000000000000000, 0.000000000000000000, 170.0000000000000000 ) ) ;
#61783=VECTOR ( 'NONE', #61836, 1000.000000000000114 ) ;
#61790=ORIENTED_EDGE ( 'NONE', *, *, #47627, .T. ) ;
#61795=EDGE_CURVE ( 'NONE', #5941, #21329, #7195, .T. ) ;
#61797=CARTESIAN_POINT ( 'NONE',  ( 26.12852347772543737, 100.0000000000000000, 129.5802547743875550 ) ) ;
#61798=LINE ( 'NONE', #68137, #40636 ) ;
#61799=DIRECTION ( 'NONE',  ( -0.000000000000000000, -0.000000000000000000, -1.000000000000000000 ) ) ;
#61803=ORIENTED_EDGE ( 'NONE', *, *, #31365, .F. ) ;
#61812=LINE ( 'NONE', #13981, #51351 ) ;
#61814=DIRECTION ( 'NONE',  ( 0.8584487936018655452, 0.5128992774059070170, 0.000000000000000000 ) ) ;
#61818=ORIENTED_EDGE ( 'NONE', *, *, #32018, .T. ) ;
#61828=DIRECTION ( 'NONE',  ( -0.9639628606958512425, -0.2660368455666826670, 0.000000000000000000 ) ) ;
#61829=ORIENTED_EDGE ( 'NONE', *, *, #5405, .F. ) ;
#61834=DIRECTION ( 'NONE',  ( -0.1785568947986370669, 0.9839295885986296675, 2.500042656554809847E-16 ) ) ;
#61836=DIRECTION ( 'NONE',  ( 0.3090169943749582759, -0.9510565162951499785, 0.000000000000000000 ) ) ;
#61838=CARTESIAN_POINT ( 'NONE',  ( -24.98026281234600887, 0.9932118737287082277, 0.000000000000000000 ) ) ;
#61844=VERTEX_POINT ( 'NONE', #4952 ) ;
#61845=DIRECTION ( 'NONE',  ( -1.000000000000000000, 0.000000000000000000, 0.000000000000000000 ) ) ;
#61874=CIRCLE ( 'NONE', #51789, 24.17157287525367693 ) ;
#61875=EDGE_CURVE ( 'NONE', #28828, #28769, #57271, .T. ) ;
#61876=EDGE_CURVE ( 'NONE', #24043, #12796, #15537, .T. ) ;
#61877=ADVANCED_FACE ( 'NONE', ( #46014 ), #67481, .T. ) ;
#61878=STYLED_ITEM ( 'NONE', ( #29874 ), #18268 ) ;
#61879=ORIENTED_EDGE ( 'NONE', *, *, #53495, .F. ) ;
#61880=ADVANCED_FACE ( 'NONE', ( #40732 ), #62191, .T. ) ;
#61883=VERTEX_POINT ( 'NONE', #14008 ) ;
#61884=CARTESIAN_POINT ( 'NONE',  ( -29.70166638324964126, 57.83280658984259048, 43.58025477438756923 ) ) ;
#61892=ORIENTED_EDGE ( 'NONE', *, *, #18012, .T. ) ;
#61893=PLANE ( 'NONE',  #52444 ) ;
#61897=DIRECTION ( 'NONE',  ( 0.1342332658176667304, -0.9909497617679331460, 0.000000000000000000 ) ) ;
#61900=EDGE_LOOP ( 'NONE', ( #44287, #50723, #30783, #51965 ) ) ;
#61903=VERTEX_POINT ( 'NONE', #62892 ) ;
#61915=DIRECTION ( 'NONE',  ( -0.000000000000000000, -0.000000000000000000, -1.000000000000000000 ) ) ;
#61920=DIRECTION ( 'NONE',  ( 0.7530714660036099684, 0.6579387259397136978, 0.000000000000000000 ) ) ;
#61929=ADVANCED_FACE ( 'NONE', ( #41089 ), #40091, .T. ) ;
#61934=CARTESIAN_POINT ( 'NONE',  ( -35.06172987636333005, -15.49744386972411903, 13.32819397642333570 ) ) ;
#61935=AXIS2_PLACEMENT_3D ( 'NONE', #32861, #12809, #59926 ) ;
#61939=EDGE_CURVE ( 'NONE', #37998, #28498, #19629, .T. ) ;
#61940=ADVANCED_FACE ( 'NONE', ( #14361 ), #68509, .T. ) ;
#61947=DIRECTION ( 'NONE',  ( 1.000000000000000000, 0.000000000000000000, 0.000000000000000000 ) ) ;
#61953=DIRECTION ( 'NONE',  ( -0.000000000000000000, -0.000000000000000000, -1.000000000000000000 ) ) ;
#61958=EDGE_LOOP ( 'NONE', ( #23148, #32691 ) ) ;
#61963=DIRECTION ( 'NONE',  ( -5.055952397801347160E-18, -6.848752866792398399E-19, -1.000000000000000000 ) ) ;
#61966=CARTESIAN_POINT ( 'NONE',  ( 69.68177367721199289, -20.52767805628082698, 170.0000000000000000 ) ) ;
#61978=CIRCLE ( 'NONE', #67621, 25.12245591505646303 ) ;
#61983=CONICAL_SURFACE ( 'NONE', #41815, 65.00000000000000000, 0.7853981633974497223 ) ;
#61994=DIRECTION ( 'NONE',  ( 0.000000000000000000, 0.000000000000000000, 1.000000000000000000 ) ) ;
#61996=EDGE_CURVE ( 'NONE', #65404, #2078, #58927, .T. ) ;
#62003=ORIENTED_EDGE ( 'NONE', *, *, #32573, .T. ) ;
#62006=ORIENTED_EDGE ( 'NONE', *, *, #43254, .T. ) ;
#62016=VERTEX_POINT ( 'NONE', #38885 ) ;
#62017=EDGE_CURVE ( 'NONE', #25506, #19578, #1587, .T. ) ;
#62023=EDGE_CURVE ( 'NONE', #34941, #36964, #23412, .T. ) ;
#62040=CARTESIAN_POINT ( 'NONE',  ( 1.667562369266826661, 64.99262834925669097, 43.58025477438756923 ) ) ;
#62044=DIRECTION ( 'NONE',  ( -0.9909497617679351444, 0.1342332658176522420, 0.000000000000000000 ) ) ;
#62050=ORIENTED_EDGE ( 'NONE', *, *, #17565, .F. ) ;
#62052=DIRECTION ( 'NONE',  ( -1.000000000000000000, 0.000000000000000000, 0.000000000000000000 ) ) ;
#62077=CARTESIAN_POINT ( 'NONE',  ( 55.46196446482078812, 34.59309596431376121, 3.125053320693586388E-16 ) ) ;
#62094=CIRCLE ( 'NONE', #23990, 65.00000000000000000 ) ;
#62095=LINE ( 'NONE', #61058, #61433 ) ;
#62118=CARTESIAN_POINT ( 'NONE',  ( -65.36598343705435354, 0.000000000000000000, 41.38025477438755928 ) ) ;
#62120=VECTOR ( 'NONE', #60810, 1000.000000000000227 ) ;
#62121=B_SPLINE_CURVE_WITH_KNOTS ( 'NONE', 3,
 ( #29866, #51329, #2788, #46035, #46727, #9104 ),
 .UNSPECIFIED., .F., .F.,
 ( 4, 2, 4 ),
 ( 1.095770181109612726E-06, 0.03239442681617711595, 0.06478775786217311206 ),
 .UNSPECIFIED. ) ;
#62123=AXIS2_PLACEMENT_3D ( 'NONE', #64425, #59136, #41592 ) ;
#62127=CARTESIAN_POINT ( 'NONE',  ( -31.90315521289065970, -56.64813493366050068, 43.58025477438756923 ) ) ;
#62131=AXIS2_PLACEMENT_3D ( 'NONE', #12526, #50508, #1622 ) ;
#62132=ORIENTED_EDGE ( 'NONE', *, *, #30440, .F. ) ;
#62146=CARTESIAN_POINT ( 'NONE',  ( 64.52696037203355672, 10.43950074664854633, 6.377659838150160580E-18 ) ) ;
#62148=EDGE_CURVE ( 'NONE', #30444, #64346, #52542, .T. ) ;
#62167=ORIENTED_EDGE ( 'NONE', *, *, #1499, .F. ) ;
#62191=PLANE ( 'NONE',  #46811 ) ;
#62192=CARTESIAN_POINT ( 'NONE',  ( 16.00641379534997455, -64.51123194475178479, 73.58025477438755502 ) ) ;
#62193=CARTESIAN_POINT ( 'NONE',  ( -29.70166638324878150, -57.83280658984300970, 0.000000000000000000 ) ) ;
#62201=DIRECTION ( 'NONE',  ( -0.3930250316539278255, 0.9195277725514487965, 0.000000000000000000 ) ) ;
#62202=CARTESIAN_POINT ( 'NONE',  ( 65.02478361689730946, 37.39438481344068776, 43.58025477438756212 ) ) ;
#62214=ORIENTED_EDGE ( 'NONE', *, *, #48862, .T. ) ;
#62223=VECTOR ( 'NONE', #41272, 1000.000000000000000 ) ;
#62225=CARTESIAN_POINT ( 'NONE',  ( -9.964117946888961797, -64.24592483216726180, 41.38025477438755928 ) ) ;
#62232=VECTOR ( 'NONE', #11342, 1000.000000000000114 ) ;
#62244=EDGE_LOOP ( 'NONE', ( #63081, #60499, #5821, #39446 ) ) ;
#62254=ADVANCED_FACE ( 'NONE', ( #52872 ), #10316, .T. ) ;
#62258=VERTEX_POINT ( 'NONE', #25139 ) ;
#62261=CARTESIAN_POINT ( 'NONE',  ( 21.27121078971695312, -61.42097029141944375, 40.00000000000003553 ) ) ;
#62272=ORIENTED_EDGE ( 'NONE', *, *, #10483, .T. ) ;
#62284=ORIENTED_EDGE ( 'NONE', *, *, #40527, .T. ) ;
#62298=ORIENTED_EDGE ( 'NONE', *, *, #10248, .T. ) ;
#62299=CARTESIAN_POINT ( 'NONE',  ( 45.78444578632068840, -59.41672343742509810, 170.0000000000000000 ) ) ;
#62314=CARTESIAN_POINT ( 'NONE',  ( 8.828807734115066808, -74.48902371486708773, 43.58025477438756212 ) ) ;
#62316=ORIENTED_EDGE ( 'NONE', *, *, #64138, .F. ) ;
#62319=EDGE_CURVE ( 'NONE', #52558, #57335, #61480, .T. ) ;
#62325=ORIENTED_EDGE ( 'NONE', *, *, #50276, .T. ) ;
#62329=VECTOR ( 'NONE', #60965, 1000.000000000000000 ) ;
#62330=VECTOR ( 'NONE', #42729, 1000.000000000000227 ) ;
#62331=VERTEX_POINT ( 'NONE', #51352 ) ;
#62333=EDGE_CURVE ( 'NONE', #3736, #25681, #2465, .T. ) ;
#62396=ORIENTED_EDGE ( 'NONE', *, *, #16335, .F. ) ;
#62403=EDGE_LOOP ( 'NONE', ( #21299, #39338, #61665, #22797 ) ) ;
#62408=EDGE_CURVE ( 'NONE', #7321, #62016, #25999, .T. ) ;
#62409=FACE_BOUND ( 'NONE', #14726, .T. ) ;
#62418=DIRECTION ( 'NONE',  ( -0.000000000000000000, -0.000000000000000000, -1.000000000000000000 ) ) ;
#62423=ORIENTED_EDGE ( 'NONE', *, *, #43014, .F. ) ;
#62425=AXIS2_PLACEMENT_3D ( 'NONE', #45559, #13559, #13898 ) ;
#62426=DIRECTION ( 'NONE',  ( -0.000000000000000000, -0.000000000000000000, 1.000000000000000000 ) ) ;
#62430=CARTESIAN_POINT ( 'NONE',  ( 57.25833571151868284, 48.36523237396223607, 41.38025477438755928 ) ) ;
#62436=VERTEX_POINT ( 'NONE', #49151 ) ;
#62444=DIRECTION ( 'NONE',  ( 0.9639628606958550172, -0.2660368455666687892, 0.000000000000000000 ) ) ;
#62456=CARTESIAN_POINT ( 'NONE',  ( 11.30618213853492904, -74.15344055032291237, 43.58025477438756923 ) ) ;
#62458=ORIENTED_EDGE ( 'NONE', *, *, #6969, .T. ) ;
#62460=CARTESIAN_POINT ( 'NONE',  ( 0.000000000000000000, 0.000000000000000000, 41.38025477438755928 ) ) ;
#62471=CARTESIAN_POINT ( 'NONE',  ( 65.02478361689784947, -37.39438481343977116, 43.58025477438756923 ) ) ;
#62475=DIRECTION ( 'NONE',  ( -0.000000000000000000, 0.000000000000000000, -1.000000000000000000 ) ) ;
#62483=LINE ( 'NONE', #50544, #66063 ) ;
#62485=DIRECTION ( 'NONE',  ( -0.000000000000000000, -0.000000000000000000, -1.000000000000000000 ) ) ;
#62491=ORIENTED_EDGE ( 'NONE', *, *, #54298, .F. ) ;
#62492=ADVANCED_FACE ( 'NONE', ( #66421 ), #24195, .F. ) ;
#62498=AXIS2_PLACEMENT_3D ( 'NONE', #2854, #25494, #43579 ) ;
#62501=EDGE_LOOP ( 'NONE', ( #51443, #2245, #53447, #11716 ) ) ;
#62506=CARTESIAN_POINT ( 'NONE',  ( 0.000000000000000000, 0.000000000000000000, 0.000000000000000000 ) ) ;
#62510=CARTESIAN_POINT ( 'NONE',  ( -2.368959188627906887, 24.88750755625416744, 0.000000000000000000 ) ) ;
#62512=ORIENTED_EDGE ( 'NONE', *, *, #133, .F. ) ;
#62537=PLANE ( 'NONE',  #5632 ) ;
#62538=EDGE_LOOP ( 'NONE', ( #215, #13324, #41487, #16726 ) ) ;
#62545=ORIENTED_EDGE ( 'NONE', *, *, #17391, .F. ) ;
#62547=AXIS2_PLACEMENT_3D ( 'NONE', #17553, #11560, #17907 ) ;
#62551=CARTESIAN_POINT ( 'NONE',  ( 0.000000000000000000, 0.000000000000000000, 41.38025477438755928 ) ) ;
#62557=ORIENTED_EDGE ( 'NONE', *, *, #7211, .F. ) ;
#62560=CARTESIAN_POINT ( 'NONE',  ( -42.52062450115279546, -29.34795704556003670, 26.66469104408689361 ) ) ;
#62563=VERTEX_POINT ( 'NONE', #23058 ) ;
#62575=ORIENTED_EDGE ( 'NONE', *, *, #45250, .F. ) ;
#62583=EDGE_CURVE ( 'NONE', #31341, #14491, #42386, .T. ) ;
#62595=B_SPLINE_CURVE_WITH_KNOTS ( 'NONE', 3,
 ( #51851, #45535, #13536, #34304 ),
 .UNSPECIFIED., .F., .F.,
 ( 4, 4 ),
 ( 0.1259919275528358917, 0.1829744153748749103 ),
 .UNSPECIFIED. ) ;
#62612=DIRECTION ( 'NONE',  ( -1.000000000000000000, 0.000000000000000000, 0.000000000000000000 ) ) ;
#62622=CARTESIAN_POINT ( 'NONE',  ( -22.17966048971185344, 25.00691465344610265, 6.893343212288939981 ) ) ;
#62629=VERTEX_POINT ( 'NONE', #17785 ) ;
#62640=ORIENTED_EDGE ( 'NONE', *, *, #38012, .T. ) ;
#62646=ORIENTED_EDGE ( 'NONE', *, *, #7939, .T. ) ;
#62648=CARTESIAN_POINT ( 'NONE',  ( -23.73638277007043840, 7.847555861075215411, 0.000000000000000000 ) ) ;
#62651=VECTOR ( 'NONE', #10252, 1000.000000000000000 ) ;
#62662=EDGE_LOOP ( 'NONE', ( #63445, #63111, #4806, #32621 ) ) ;
#62687=CARTESIAN_POINT ( 'NONE',  ( -16.35146342289110422, 18.91109843266242052, 0.000000000000000000 ) ) ;
#62688=EDGE_CURVE ( 'NONE', #35709, #695, #27231, .T. ) ;
#62694=CARTESIAN_POINT ( 'NONE',  ( -65.20298343242130557, -4.613322252418190494, 6.377659838150142091E-18 ) ) ;
#62704=CARTESIAN_POINT ( 'NONE',  ( 16.54503815046451010, -18.74197728628616844, 0.000000000000000000 ) ) ;
#62707=DIRECTION ( 'NONE',  ( 0.000000000000000000, 0.000000000000000000, 1.000000000000000000 ) ) ;
#62717=LINE ( 'NONE', #47543, #36141 ) ;
#62722=EDGE_CURVE ( 'NONE', #476, #15914, #40613, .T. ) ;
#62727=VECTOR ( 'NONE', #39816, 1000.000000000000000 ) ;
#62732=VECTOR ( 'NONE', #7733, 1000.000000000000114 ) ;
#62736=VERTEX_POINT ( 'NONE', #45545 ) ;
#62744=DIRECTION ( 'NONE',  ( -0.000000000000000000, -0.000000000000000000, -1.000000000000000000 ) ) ;
#62748=LINE ( 'NONE', #57809, #4678 ) ;
#62752=DIRECTION ( 'NONE',  ( 0.3930250316539148359, 0.9195277725514544587, 0.000000000000000000 ) ) ;
#62756=VERTEX_POINT ( 'NONE', #61383 ) ;
#62765=CARTESIAN_POINT ( 'NONE',  ( -15.47041015649658391, 73.39774458108210808, 73.58025477438756923 ) ) ;
#62766=EDGE_CURVE ( 'NONE', #40228, #58737, #55400, .T. ) ;
#62771=EDGE_CURVE ( 'NONE', #36722, #15646, #21108, .T. ) ;
#62778=CARTESIAN_POINT ( 'NONE',  ( -34.75846525698938194, -54.92585086258257121, 170.0000000000000000 ) ) ;
#62779=ORIENTED_EDGE ( 'NONE', *, *, #69541, .T. ) ;
#62783=ORIENTED_EDGE ( 'NONE', *, *, #46678, .F. ) ;
#62785=CARTESIAN_POINT ( 'NONE',  ( 3.245026627011502907, -33.26789626822845491, 6.893343212288929323 ) ) ;
#62793=EDGE_LOOP ( 'NONE', ( #33389, #30304, #57983, #32644, #18410, #21063, #60928, #34202, #40264 ) ) ;
#62795=B_SPLINE_CURVE_WITH_KNOTS ( 'NONE', 3,
 ( #4349, #20173, #41627, #18885 ),
 .UNSPECIFIED., .F., .F.,
 ( 4, 4 ),
 ( 0.1259919275528361415, 0.1829744153748754654 ),
 .UNSPECIFIED. ) ;
#62798=FACE_OUTER_BOUND ( 'NONE', #14344, .T. ) ;
#62800=LINE ( 'NONE', #67737, #19153 ) ;
#62804=ORIENTED_EDGE ( 'NONE', *, *, #8082, .T. ) ;
#62843=ORIENTED_EDGE ( 'NONE', *, *, #57121, .T. ) ;
#62845=ORIENTED_EDGE ( 'NONE', *, *, #57723, .F. ) ;
#62848=CARTESIAN_POINT ( 'NONE',  ( -29.72794987547381140, 29.28418937382772569, 13.79046412439885927 ) ) ;
#62850=CARTESIAN_POINT ( 'NONE',  ( 29.86848256228606502, -58.14280299503694494, 6.377659838150125914E-18 ) ) ;
#62853=LINE ( 'NONE', #62146, #42093 ) ;
#62854=VERTEX_POINT ( 'NONE', #36036 ) ;
#62857=ORIENTED_EDGE ( 'NONE', *, *, #11125, .T. ) ;
#62865=LINE ( 'NONE', #51956, #23881 ) ;
#62869=CARTESIAN_POINT ( 'NONE',  ( -56.44201257846588504, -32.26641783793643015, 3.061616997868437868E-16 ) ) ;
#62873=VECTOR ( 'NONE', #39844, 1000.000000000000000 ) ;
#62874=ORIENTED_EDGE ( 'NONE', *, *, #44740, .T. ) ;
#62885=ORIENTED_EDGE ( 'NONE', *, *, #36906, .F. ) ;
#62889=EDGE_CURVE ( 'NONE', #57138, #26335, #33181, .T. ) ;
#62892=CARTESIAN_POINT ( 'NONE',  ( -59.42430146430426419, 27.22983999535709287, 43.58025477438756212 ) ) ;
#62920=ORIENTED_EDGE ( 'NONE', *, *, #25645, .F. ) ;
#62924=( NAMED_UNIT ( * ) SI_UNIT ( $, .STERADIAN. ) SOLID_ANGLE_UNIT ( ) );
#62929=CARTESIAN_POINT ( 'NONE',  ( -51.84164840787130402, -39.21024726209533640, 170.0000000000000000 ) ) ;
#62931=DIRECTION ( 'NONE',  ( 0.000000000000000000, 0.000000000000000000, 1.000000000000000000 ) ) ;
#62951=VERTEX_POINT ( 'NONE', #50740 ) ;
#62953=ORIENTED_EDGE ( 'NONE', *, *, #10851, .T. ) ;
#62956=ADVANCED_FACE ( 'NONE', ( #28599 ), #44776, .T. ) ;
#62976=ORIENTED_EDGE ( 'NONE', *, *, #32018, .F. ) ;
#62985=FACE_OUTER_BOUND ( 'NONE', #67217, .T. ) ;
#62988=ORIENTED_EDGE ( 'NONE', *, *, #33758, .F. ) ;
#63006=VECTOR ( 'NONE', #38373, 1000.000000000000000 ) ;
#63020=ORIENTED_EDGE ( 'NONE', *, *, #22308, .F. ) ;
#63021=EDGE_CURVE ( 'NONE', #21253, #64530, #61643, .T. ) ;
#63026=DIRECTION ( 'NONE',  ( -0.1342332658176522420, -0.9909497617679352555, 0.000000000000000000 ) ) ;
#63028=ORIENTED_EDGE ( 'NONE', *, *, #3920, .T. ) ;
#63030=AXIS2_PLACEMENT_3D ( 'NONE', #69300, #21127, #42571 ) ;
#63035=PLANE ( 'NONE',  #21119 ) ;
#63036=PLANE ( 'NONE',  #2928 ) ;
#63039=PLANE ( 'NONE',  #60878 ) ;
#63040=ADVANCED_FACE ( 'NONE', ( #56716 ), #27820, .T. ) ;
#63043=VECTOR ( 'NONE', #8577, 1000.000000000000114 ) ;
#63057=VECTOR ( 'NONE', #42546, 1000.000000000000000 ) ;
#63063=ORIENTED_EDGE ( 'NONE', *, *, #66253, .T. ) ;
#63066=CARTESIAN_POINT ( 'NONE',  ( -59.09450113343241640, 27.07101652673493319, 40.00000000000003553 ) ) ;
#63068=EDGE_CURVE ( 'NONE', #56795, #21961, #57400, .T. ) ;
#63072=FACE_OUTER_BOUND ( 'NONE', #41473, .T. ) ;
#63081=ORIENTED_EDGE ( 'NONE', *, *, #12539, .T. ) ;
#63087=DIRECTION ( 'NONE',  ( 1.000000000000000000, 0.000000000000000000, 0.000000000000000000 ) ) ;
#63096=CIRCLE ( 'NONE', #2450, 24.99999999999985434 ) ;
#63103=CARTESIAN_POINT ( 'NONE',  ( 63.72039997003725631, -12.83396383267754537, 40.00000000000003553 ) ) ;
#63104=CIRCLE ( 'NONE', #32772, 65.00000000000000000 ) ;
#63109=B_SPLINE_CURVE_WITH_KNOTS ( 'NONE', 3,
 ( #11805, #58014, #54714, #22716 ),
 .UNSPECIFIED., .F., .F.,
 ( 4, 4 ),
 ( 9.900409498990251444E-07, 0.05658314289920113316 ),
 .UNSPECIFIED. ) ;
#63111=ORIENTED_EDGE ( 'NONE', *, *, #59527, .F. ) ;
#63119=DIRECTION ( 'NONE',  ( -0.000000000000000000, -0.000000000000000000, -1.000000000000000000 ) ) ;
#63122=ORIENTED_EDGE ( 'NONE', *, *, #49375, .F. ) ;
#63141=EDGE_CURVE ( 'NONE', #26680, #27057, #12120, .T. ) ;
#63142=DIRECTION ( 'NONE',  ( 0.000000000000000000, 0.000000000000000000, 1.000000000000000000 ) ) ;
#63143=CIRCLE ( 'NONE', #64232, 65.36598343705435354 ) ;
#63144=CARTESIAN_POINT ( 'NONE',  ( -60.57719060482967421, 27.78504214373295511, 34.48241823988800547 ) ) ;
#63149=ORIENTED_EDGE ( 'NONE', *, *, #37558, .T. ) ;
#63150=AXIS2_PLACEMENT_3D ( 'NONE', #32336, #48821, #16492 ) ;
#63163=EDGE_CURVE ( 'NONE', #14371, #41081, #26774, .T. ) ;
#63180=ORIENTED_EDGE ( 'NONE', *, *, #15034, .T. ) ;
#63185=ORIENTED_EDGE ( 'NONE', *, *, #53796, .F. ) ;
#63194=AXIS2_PLACEMENT_3D ( 'NONE', #41749, #63209, #472 ) ;
#63206=ORIENTED_EDGE ( 'NONE', *, *, #13653, .T. ) ;
#63208=VECTOR ( 'NONE', #4111, 1000.000000000000000 ) ;
#63209=DIRECTION ( 'NONE',  ( -0.000000000000000000, -0.000000000000000000, -1.000000000000000000 ) ) ;
#63212=EDGE_CURVE ( 'NONE', #34656, #62854, #64751, .T. ) ;
#63213=LINE ( 'NONE', #57592, #26371 ) ;
#63218=ADVANCED_FACE ( 'NONE', ( #38013 ), #22254, .T. ) ;
#63223=CARTESIAN_POINT ( 'NONE',  ( 36.85262215550149278, -53.56030941157680303, 170.0000000000000000 ) ) ;
#63231=ORIENTED_EDGE ( 'NONE', *, *, #69567, .F. ) ;
#63233=FACE_OUTER_BOUND ( 'NONE', #30761, .T. ) ;
#63237=DIRECTION ( 'NONE',  ( -0.000000000000000000, -0.000000000000000000, -1.000000000000000000 ) ) ;
#63241=LINE ( 'NONE', #41095, #14651 ) ;
#63248=CARTESIAN_POINT ( 'NONE',  ( -36.84489839129339828, 53.54860840895182150, 170.0000000000000000 ) ) ;
#63256=CIRCLE ( 'NONE', #52050, 65.36598343705435354 ) ;
#63259=AXIS2_PLACEMENT_3D ( 'NONE', #60624, #49004, #54641 ) ;
#63263=CARTESIAN_POINT ( 'NONE',  ( 15.68296563925591514, -63.09411298019745828, 170.0000000000000000 ) ) ;
#63273=CARTESIAN_POINT ( 'NONE',  ( 39.77028211725815510, -51.87520073220884598, 41.38025477438755928 ) ) ;
#63275=PLANE ( 'NONE',  #6082 ) ;
#63285=VECTOR ( 'NONE', #47206, 1000.000000000000000 ) ;
#63289=CARTESIAN_POINT ( 'NONE',  ( 6.526941389886052214, 24.13294503563511029, 0.000000000000000000 ) ) ;
#63293=CARTESIAN_POINT ( 'NONE',  ( 20.86596623802176609, -36.13760097092460910, 13.79046412339527805 ) ) ;
#63294=ADVANCED_FACE ( 'NONE', ( #2820 ), #44702, .T. ) ;
#63296=DIRECTION ( 'NONE',  ( 0.9989930665413144784, 0.04486483035051863633, 5.102127870520020458E-18 ) ) ;
#63305=DIRECTION ( 'NONE',  ( 0.000000000000000000, 0.000000000000000000, 1.000000000000000000 ) ) ;
#63321=FACE_OUTER_BOUND ( 'NONE', #40070, .T. ) ;
#63336=DIRECTION ( 'NONE',  ( 1.000000000000000000, 0.000000000000000000, 0.000000000000000000 ) ) ;
#63337=ORIENTED_EDGE ( 'NONE', *, *, #40820, .F. ) ;
#63348=ORIENTED_EDGE ( 'NONE', *, *, #12621, .F. ) ;
#63356=EDGE_CURVE ( 'NONE', #57513, #43949, #5492, .T. ) ;
#63367=ORIENTED_EDGE ( 'NONE', *, *, #12225, .T. ) ;
#63370=LINE ( 'NONE', #20111, #3831 ) ;
#63385=FACE_OUTER_BOUND ( 'NONE', #46278, .T. ) ;
#63389=CARTESIAN_POINT ( 'NONE',  ( 0.000000000000000000, 0.000000000000000000, 0.000000000000000000 ) ) ;
#63394=LINE ( 'NONE', #63741, #19308 ) ;
#63401=AXIS2_PLACEMENT_3D ( 'NONE', #44317, #49942, #27797 ) ;
#63407=CYLINDRICAL_SURFACE ( 'NONE', #15900, 65.36598343705435354 ) ;
#63431=VECTOR ( 'NONE', #54439, 1000.000000000000000 ) ;
#63445=ORIENTED_EDGE ( 'NONE', *, *, #12015, .T. ) ;
#63446=ORIENTED_EDGE ( 'NONE', *, *, #17607, .T. ) ;
#63454=EDGE_CURVE ( 'NONE', #3025, #28173, #12169, .T. ) ;
#63462=CARTESIAN_POINT ( 'NONE',  ( -63.73419499958997392, 12.83646726144839079, 3.061616997868437868E-16 ) ) ;
#63478=DIRECTION ( 'NONE',  ( 0.000000000000000000, 0.000000000000000000, 1.000000000000000000 ) ) ;
#63479=EDGE_LOOP ( 'NONE', ( #54600, #45520, #831, #41116 ) ) ;
#63480=ORIENTED_EDGE ( 'NONE', *, *, #45020, .F. ) ;
#63495=AXIS2_PLACEMENT_3D ( 'NONE', #4030, #51867, #13551 ) ;
#63504=DIRECTION ( 'NONE',  ( -0.000000000000000000, -0.000000000000000000, -1.000000000000000000 ) ) ;
#63508=PLANE ( 'NONE',  #44448 ) ;
#63512=CARTESIAN_POINT ( 'NONE',  ( -4.364688291132793552, 24.74039788130344419, 0.000000000000000000 ) ) ;
#63521=DIRECTION ( 'NONE',  ( -0.9989930665413151445, 0.04486483035050446017, 0.000000000000000000 ) ) ;
#63537=DIRECTION ( 'NONE',  ( 0.9839295885986295565, 0.1785568947986370392, 0.000000000000000000 ) ) ;
#63543=VERTEX_POINT ( 'NONE', #57162 ) ;
#63545=CARTESIAN_POINT ( 'NONE',  ( 0.000000000000000000, 0.000000000000000000, 40.00000000000003553 ) ) ;
#63546=EDGE_CURVE ( 'NONE', #42469, #24394, #13896, .T. ) ;
#63552=EDGE_CURVE ( 'NONE', #7998, #59358, #55776, .T. ) ;
#63554=ORIENTED_EDGE ( 'NONE', *, *, #11015, .T. ) ;
#63555=DIRECTION ( 'NONE',  ( -0.000000000000000000, -0.000000000000000000, -1.000000000000000000 ) ) ;
#63573=ORIENTED_EDGE ( 'NONE', *, *, #61307, .T. ) ;
#63579=CARTESIAN_POINT ( 'NONE',  ( 0.000000000000000000, 0.000000000000000000, 0.000000000000000000 ) ) ;
#63581=PLANE ( 'NONE',  #13634 ) ;
#63588=DIRECTION ( 'NONE',  ( -1.000000000000000000, 0.000000000000000000, 0.000000000000000000 ) ) ;
#63593=DIRECTION ( 'NONE',  ( -1.000000000000000000, 0.000000000000000000, 0.000000000000000000 ) ) ;
#63595=DIRECTION ( 'NONE',  ( 1.000000000000000000, 0.000000000000000000, 0.000000000000000000 ) ) ;
#63598=DIRECTION ( 'NONE',  ( 1.000000000000000000, 0.000000000000000000, 0.000000000000000000 ) ) ;
#63602=EDGE_LOOP ( 'NONE', ( #9173, #26361, #6668, #18843 ) ) ;
#63605=DIRECTION ( 'NONE',  ( 1.000000000000000000, 0.000000000000000000, 0.000000000000000000 ) ) ;
#63609=CARTESIAN_POINT ( 'NONE',  ( 2.129405171194437063, -25.03204795498853841, 0.000000000000000000 ) ) ;
#63612=CARTESIAN_POINT ( 'NONE',  ( -26.69131247781221106, -59.26697088777007849, 40.00000000000003553 ) ) ;
#63615=DIRECTION ( 'NONE',  ( -1.000000000000000000, -0.000000000000000000, 2.312964634635743450E-16 ) ) ;
#63617=VERTEX_POINT ( 'NONE', #58519 ) ;
#63619=LINE ( 'NONE', #68872, #252 ) ;
#63624=CARTESIAN_POINT ( 'NONE',  ( -53.31111153860302210, 37.18770477615724701, 40.00000000000003553 ) ) ;
#63630=CARTESIAN_POINT ( 'NONE',  ( 63.69186821587121017, 39.51023455020778385, 41.38025477438755928 ) ) ;
#63636=CARTESIAN_POINT ( 'NONE',  ( 10.65073749997984898, 36.82468443433825911, 13.32819299319723960 ) ) ;
#63638=ADVANCED_FACE ( 'NONE', ( #65551 ), #36877, .T. ) ;
#63641=ORIENTED_EDGE ( 'NONE', *, *, #10769, .F. ) ;
#63642=CARTESIAN_POINT ( 'NONE',  ( 16.54503815046424009, 18.74197728628641002, 0.000000000000000000 ) ) ;
#63645=CARTESIAN_POINT ( 'NONE',  ( 0.000000000000000000, 0.000000000000000000, 41.38025477438755928 ) ) ;
#63646=AXIS2_PLACEMENT_3D ( 'NONE', #67922, #57356, #4243 ) ;
#63660=PLANE ( 'NONE',  #2212 ) ;
#63663=ORIENTED_EDGE ( 'NONE', *, *, #16289, .T. ) ;
#63664=DIRECTION ( 'NONE',  ( -0.04486483035050447404, -0.9989930665413151445, 0.000000000000000000 ) ) ;
#63665=ORIENTED_EDGE ( 'NONE', *, *, #27390, .F. ) ;
#63669=CARTESIAN_POINT ( 'NONE',  ( 0.000000000000000000, 0.000000000000000000, 40.00000000000003553 ) ) ;
#63675=EDGE_LOOP ( 'NONE', ( #33767, #38306, #49252, #14818 ) ) ;
#63676=ORIENTED_EDGE ( 'NONE', *, *, #44691, .F. ) ;
#63681=FACE_OUTER_BOUND ( 'NONE', #62662, .T. ) ;
#63692=CIRCLE ( 'NONE', #33369, 65.00000000000000000 ) ;
#63703=CARTESIAN_POINT ( 'NONE',  ( 46.76173513940489812, 58.63736118510233553, 43.58025477438756212 ) ) ;
#63714=ORIENTED_EDGE ( 'NONE', *, *, #42167, .T. ) ;
#63718=EDGE_LOOP ( 'NONE', ( #25931, #31943, #19285, #8221 ) ) ;
#63723=VECTOR ( 'NONE', #37885, 1000.000000000000000 ) ;
#63729=VECTOR ( 'NONE', #40493, 1000.000000000000000 ) ;
#63731=EDGE_LOOP ( 'NONE', ( #68350, #26370, #40603, #57776, #22039, #13470, #42986, #67840, #45556 ) ) ;
#63733=LINE ( 'NONE', #46857, #10690 ) ;
#63741=CARTESIAN_POINT ( 'NONE',  ( 34.43940527065477397, -66.63700071734618291, 170.0000000000000000 ) ) ;
#63746=VECTOR ( 'NONE', #566, 1000.000000000000000 ) ;
#63749=LINE ( 'NONE', #26799, #37407 ) ;
#63750=VERTEX_POINT ( 'NONE', #44787 ) ;
#63753=CARTESIAN_POINT ( 'NONE',  ( -65.20298343242134820, 4.613322252417262348, 41.38025477438755928 ) ) ;
#63759=CARTESIAN_POINT ( 'NONE',  ( -8.712114576423529044, -23.56346432108879441, 3.061616997868437868E-16 ) ) ;
#63761=EDGE_CURVE ( 'NONE', #22952, #33925, #32093, .T. ) ;
#63764=CARTESIAN_POINT ( 'NONE',  ( 24.34427655538949509, 5.688250960946272805, 0.000000000000000000 ) ) ;
#63773=DIRECTION ( 'NONE',  ( 1.000000000000000000, 0.000000000000000000, 0.000000000000000000 ) ) ;
#63781=VECTOR ( 'NONE', #62044, 1000.000000000000227 ) ;
#63789=AXIS2_PLACEMENT_3D ( 'NONE', #58765, #17245, #37662 ) ;
#63790=VERTEX_POINT ( 'NONE', #69345 ) ;
#63793=ORIENTED_EDGE ( 'NONE', *, *, #17869, .T. ) ;
#63805=EDGE_LOOP ( 'NONE', ( #37733, #64617, #33946, #66576 ) ) ;
#63807=CARTESIAN_POINT ( 'NONE',  ( 0.000000000000000000, 0.000000000000000000, 73.58025477438756923 ) ) ;
#63808=LINE ( 'NONE', #63462, #35226 ) ;
#63811=DIRECTION ( 'NONE',  ( 0.9959742939952397345, -0.08963930890342655666, 0.000000000000000000 ) ) ;
#63826=VECTOR ( 'NONE', #48175, 1000.000000000000000 ) ;
#63833=CARTESIAN_POINT ( 'NONE',  ( -21.27554331372908081, -61.43430442924895374, 170.0000000000000000 ) ) ;
#63838=EDGE_CURVE ( 'NONE', #59358, #23153, #43622, .T. ) ;
#63841=CARTESIAN_POINT ( 'NONE',  ( 75.00000000000000000, 1.249999999999979350, 170.0000000000000000 ) ) ;
#63864=CARTESIAN_POINT ( 'NONE',  ( 48.39383208188379371, 43.94028683479089636, 43.58025477438756212 ) ) ;
#63870=CARTESIAN_POINT ( 'NONE',  ( -18.15845058245935562, -17.18344181019548955, 0.000000000000000000 ) ) ;
#63877=FACE_OUTER_BOUND ( 'NONE', #67608, .T. ) ;
#63879=AXIS2_PLACEMENT_3D ( 'NONE', #43383, #64328, #33016 ) ;
#63901=ORIENTED_EDGE ( 'NONE', *, *, #35581, .F. ) ;
#63911=FACE_OUTER_BOUND ( 'NONE', #66503, .T. ) ;
#63917=DIRECTION ( 'NONE',  ( 0.6579387259397028176, 0.7530714660036196273, 2.500042656554810340E-16 ) ) ;
#63920=CARTESIAN_POINT ( 'NONE',  ( -46.06722295615723795, -46.37372919877119415, 41.38025477438755928 ) ) ;
#63938=EDGE_CURVE ( 'NONE', #55116, #25227, #9497, .T. ) ;
#63942=CARTESIAN_POINT ( 'NONE',  ( 0.000000000000000000, 0.000000000000000000, 40.00000000000003553 ) ) ;
#63943=EDGE_CURVE ( 'NONE', #61153, #22625, #53869, .T. ) ;
#63959=ORIENTED_EDGE ( 'NONE', *, *, #62148, .T. ) ;
#63961=ORIENTED_EDGE ( 'NONE', *, *, #13762, .F. ) ;
#63969=CARTESIAN_POINT ( 'NONE',  ( -4.364688291132434728, -24.74039788130350459, 3.061616997868437868E-16 ) ) ;
#63971=CARTESIAN_POINT ( 'NONE',  ( -15.76129977463437015, -63.43731725181460490, 41.38025477438755928 ) ) ;
#63983=VECTOR ( 'NONE', #15709, 1000.000000000000114 ) ;
#63986=DIRECTION ( 'NONE',  ( -1.000000000000000000, 0.000000000000000000, 0.000000000000000000 ) ) ;
#63992=CARTESIAN_POINT ( 'NONE',  ( -8.062763165560543399, 40.94272254494899244, 13.79046340968178264 ) ) ;
#63999=ADVANCED_FACE ( 'NONE', ( #10173 ), #10862, .F. ) ;
#64005=EDGE_CURVE ( 'NONE', #42885, #37440, #13331, .T. ) ;
#64010=CARTESIAN_POINT ( 'NONE',  ( 11.70038247058342051, 40.05515948024370232, 13.79046412305353009 ) ) ;
#64015=CARTESIAN_POINT ( 'NONE',  ( 0.000000000000000000, 0.000000000000000000, 170.0000000000000000 ) ) ;
#64028=PLANE ( 'NONE',  #45057 ) ;
#64034=VERTEX_POINT ( 'NONE', #49169 ) ;
#64035=CARTESIAN_POINT ( 'NONE',  ( 74.39890044415633952, 7.951074708187157114, 0.000000000000000000 ) ) ;
#64051=VERTEX_POINT ( 'NONE', #32670 ) ;
#64056=CARTESIAN_POINT ( 'NONE',  ( 10.01137213834873840, 64.59476928204603041, 43.58025477438756212 ) ) ;
#64060=CARTESIAN_POINT ( 'NONE',  ( -13.24252603915519444, -63.63674649211960599, 40.00000000000003553 ) ) ;
#64065=CARTESIAN_POINT ( 'NONE',  ( -24.40147488398704567, -5.437648709335880071, 0.000000000000000000 ) ) ;
#64083=ADVANCED_FACE ( 'NONE', ( #11538 ), #16140, .F. ) ;
#64087=CARTESIAN_POINT ( 'NONE',  ( -8.663926357538780820, -23.45072237845004182, 0.000000000000000000 ) ) ;
#64101=DIRECTION ( 'NONE',  ( -0.000000000000000000, -0.000000000000000000, -1.000000000000000000 ) ) ;
#64103=EDGE_CURVE ( 'NONE', #47168, #21445, #9958, .T. ) ;
#64121=VERTEX_POINT ( 'NONE', #50242 ) ;
#64134=FACE_OUTER_BOUND ( 'NONE', #41383, .T. ) ;
#64138=EDGE_CURVE ( 'NONE', #19844, #15020, #60446, .T. ) ;
#64147=EDGE_LOOP ( 'NONE', ( #63665, #52649, #48380, #15295, #31770, #60145, #8725, #53371, #62512 ) ) ;
#64148=ORIENTED_EDGE ( 'NONE', *, *, #38703, .T. ) ;
#64152=FACE_OUTER_BOUND ( 'NONE', #63479, .T. ) ;
#64157=CARTESIAN_POINT ( 'NONE',  ( 2.129405171194075130, 25.03204795498856683, 3.061616997868437868E-16 ) ) ;
#64159=EDGE_LOOP ( 'NONE', ( #35733, #42375, #15086, #47329 ) ) ;
#64171=VERTEX_POINT ( 'NONE', #2064 ) ;
#64172=ORIENTED_EDGE ( 'NONE', *, *, #37320, .T. ) ;
#64176=AXIS2_PLACEMENT_3D ( 'NONE', #6317, #1050, #44291 ) ;
#64180=LINE ( 'NONE', #65587, #8765 ) ;
#64185=FACE_OUTER_BOUND ( 'NONE', #4423, .T. ) ;
#64188=ADVANCED_FACE ( 'NONE', ( #55873 ), #33724, .T. ) ;
#64189=CARTESIAN_POINT ( 'NONE',  ( -64.97888516016280391, 7.103257987405394935, 43.58025477438756212 ) ) ;
#64191=VECTOR ( 'NONE', #67662, 1000.000000000000000 ) ;
#64200=ORIENTED_EDGE ( 'NONE', *, *, #59924, .T. ) ;
#64207=EDGE_LOOP ( 'NONE', ( #47, #53570, #35798, #57512 ) ) ;
#64216=PLANE ( 'NONE',  #28598 ) ;
#64217=ADVANCED_FACE ( 'NONE', ( #39002 ), #44255, .T. ) ;
#64219=ORIENTED_EDGE ( 'NONE', *, *, #18012, .F. ) ;
#64229=EDGE_CURVE ( 'NONE', #35720, #55116, #10902, .T. ) ;
#64232=AXIS2_PLACEMENT_3D ( 'NONE', #30591, #15102, #64316 ) ;
#64235=VECTOR ( 'NONE', #51379, 1000.000000000000227 ) ;
#64238=DIRECTION ( 'NONE',  ( -0.3090169943749447312, -0.9510565162951544194, 7.147453794906795954E-17 ) ) ;
#64243=EDGE_CURVE ( 'NONE', #4465, #6992, #37634, .T. ) ;
#64248=FACE_OUTER_BOUND ( 'NONE', #39808, .T. ) ;
#64258=DIRECTION ( 'NONE',  ( 0.000000000000000000, 0.000000000000000000, -1.000000000000000000 ) ) ;
#64268=ORIENTED_EDGE ( 'NONE', *, *, #44740, .F. ) ;
#64272=DIRECTION ( 'NONE',  ( -0.000000000000000000, -0.000000000000000000, -1.000000000000000000 ) ) ;
#64280=B_SPLINE_CURVE_WITH_KNOTS ( 'NONE', 3,
 ( #834, #10676, #32150, #38462 ),
 .UNSPECIFIED., .F., .F.,
 ( 4, 4 ),
 ( 0.1259919275528360028, 0.1829744153748751878 ),
 .UNSPECIFIED. ) ;
#64296=CARTESIAN_POINT ( 'NONE',  ( -29.87147652227456263, 100.0000000000000000, 73.58025477438756923 ) ) ;
#64302=LINE ( 'NONE', #4528, #45371 ) ;
#64303=AXIS2_PLACEMENT_3D ( 'NONE', #39157, #12418, #40709 ) ;
#64316=DIRECTION ( 'NONE',  ( -1.000000000000000000, 0.000000000000000000, 0.000000000000000000 ) ) ;
#64318=PLANE ( 'NONE',  #27721 ) ;
#64319=CARTESIAN_POINT ( 'NONE',  ( 70.65683382808231272, -25.18281821780013274, 170.0000000000000000 ) ) ;
#64322=ADVANCED_FACE ( 'NONE', ( #5287 ), #59772, .T. ) ;
#64325=ORIENTED_EDGE ( 'NONE', *, *, #29262, .T. ) ;
#64328=DIRECTION ( 'NONE',  ( -0.000000000000000000, -0.000000000000000000, -1.000000000000000000 ) ) ;
#64329=CIRCLE ( 'NONE', #20542, 65.36598343705435354 ) ;
#64334=CARTESIAN_POINT ( 'NONE',  ( -11.76013725602017779, 57.14197687341855669, 27.58472315868181113 ) ) ;
#64345=LINE ( 'NONE', #10529, #34444 ) ;
#64346=VERTEX_POINT ( 'NONE', #54140 ) ;
#64347=CARTESIAN_POINT ( 'NONE',  ( -14.86595946518020739, 20.25193917588078563, 3.061616997868437868E-16 ) ) ;
#64348=CARTESIAN_POINT ( 'NONE',  ( -74.52723870109949189, 7.962625360374199879, 41.38025477438755928 ) ) ;
#64355=VERTEX_POINT ( 'NONE', #53797 ) ;
#64357=CARTESIAN_POINT ( 'NONE',  ( -61.29635759142585982, -21.66977272663579868, 3.061616997868437868E-16 ) ) ;
#64358=ORIENTED_EDGE ( 'NONE', *, *, #40738, .F. ) ;
#64360=DIRECTION ( 'NONE',  ( -1.000000000000000000, 0.000000000000000000, 0.000000000000000000 ) ) ;
#64365=ADVANCED_FACE ( 'NONE', ( #66141 ), #60134, .T. ) ;
#64369=ORIENTED_EDGE ( 'NONE', *, *, #24546, .T. ) ;
#64372=AXIS2_PLACEMENT_3D ( 'NONE', #36321, #53852, #42624 ) ;
#64373=FACE_OUTER_BOUND ( 'NONE', #20296, .T. ) ;
#64380=EDGE_CURVE ( 'NONE', #65498, #36599, #7383, .T. ) ;
#64382=VERTEX_POINT ( 'NONE', #50291 ) ;
#64388=AXIS2_PLACEMENT_3D ( 'NONE', #12892, #17817, #39273 ) ;
#64389=EDGE_LOOP ( 'NONE', ( #66128, #18411, #11590, #51129 ) ) ;
#64398=FACE_OUTER_BOUND ( 'NONE', #3678, .T. ) ;
#64401=PLANE ( 'NONE',  #12536 ) ;
#64402=ADVANCED_FACE ( 'NONE', ( #23903 ), #52671, .T. ) ;
#64412=LINE ( 'NONE', #32414, #63006 ) ;
#64413=CARTESIAN_POINT ( 'NONE',  ( -44.26023579658939866, 48.10138582123772721, 6.377659838150142091E-18 ) ) ;
#64415=DIRECTION ( 'NONE',  ( -0.000000000000000000, -0.000000000000000000, -1.000000000000000000 ) ) ;
#64421=ORIENTED_EDGE ( 'NONE', *, *, #13379, .T. ) ;
#64425=CARTESIAN_POINT ( 'NONE',  ( 0.000000000000000000, 0.000000000000000000, 41.38025477438755928 ) ) ;
#64433=AXIS2_PLACEMENT_3D ( 'NONE', #40049, #66108, #13658 ) ;
#64434=CARTESIAN_POINT ( 'NONE',  ( -21.03405120204953960, -13.73704776265678440, 0.000000000000000000 ) ) ;
#64443=LINE ( 'NONE', #16252, #26278 ) ;
#64449=CARTESIAN_POINT ( 'NONE',  ( -65.36598343705435354, 0.000000000000000000, 41.38025477438755928 ) ) ;
#64453=B_SPLINE_CURVE_WITH_KNOTS ( 'NONE', 3,
 ( #56677, #20082, #14462, #35221 ),
 .UNSPECIFIED., .F., .F.,
 ( 4, 4 ),
 ( 0.1259919275528356697, 0.1829744153748742441 ),
 .UNSPECIFIED. ) ;
#64459=DIRECTION ( 'NONE',  ( 0.000000000000000000, 0.000000000000000000, 1.000000000000000000 ) ) ;
#64468=EDGE_CURVE ( 'NONE', #25148, #19844, #44667, .T. ) ;
#64473=DIRECTION ( 'NONE',  ( -0.000000000000000000, 0.000000000000000000, -1.000000000000000000 ) ) ;
#64474=CARTESIAN_POINT ( 'NONE',  ( -0.4701925472693525565, 38.33111774246623327, 13.32819397642332149 ) ) ;
#64488=VECTOR ( 'NONE', #23225, 1000.000000000000000 ) ;
#64491=PLANE ( 'NONE',  #3325 ) ;
#64497=VERTEX_POINT ( 'NONE', #46041 ) ;
#64504=DIRECTION ( 'NONE',  ( 0.000000000000000000, 0.000000000000000000, 1.000000000000000000 ) ) ;
#64522=VERTEX_POINT ( 'NONE', #63612 ) ;
#64523=VERTEX_POINT ( 'NONE', #69219 ) ;
#64530=VERTEX_POINT ( 'NONE', #54058 ) ;
#64531=AXIS2_PLACEMENT_3D ( 'NONE', #29769, #51232, #45248 ) ;
#64536=FACE_OUTER_BOUND ( 'NONE', #23611, .T. ) ;
#64553=ORIENTED_EDGE ( 'NONE', *, *, #21405, .T. ) ;
#64559=EDGE_CURVE ( 'NONE', #1423, #40870, #2028, .T. ) ;
#64560=DIRECTION ( 'NONE',  ( 1.000000000000000000, 0.000000000000000000, 0.000000000000000000 ) ) ;
#64565=CARTESIAN_POINT ( 'NONE',  ( -9.964117946889912147, 64.24592483216710548, 43.58025477438756923 ) ) ;
#64572=EDGE_LOOP ( 'NONE', ( #58670, #53302, #7313, #28113, #55897, #42300, #46967, #45103, #14797 ) ) ;
#64580=ORIENTED_EDGE ( 'NONE', *, *, #58535, .F. ) ;
#64582=CONICAL_SURFACE ( 'NONE', #562, 65.00000000000000000, 0.7853981633974497223 ) ;
#64583=AXIS2_PLACEMENT_3D ( 'NONE', #21881, #22239, #10632 ) ;
#64584=ORIENTED_EDGE ( 'NONE', *, *, #20893, .F. ) ;
#64591=CARTESIAN_POINT ( 'NONE',  ( -51.33022611924979373, -5.874856440034677441, 26.66469066592268433 ) ) ;
#64595=EDGE_LOOP ( 'NONE', ( #55720, #29704, #52240, #54436, #8495, #48535, #53435, #60238, #22107 ) ) ;
#64600=DIRECTION ( 'NONE',  ( 1.000000000000000000, 2.220446049250313396E-14, 0.000000000000000000 ) ) ;
#64615=CARTESIAN_POINT ( 'NONE',  ( -9.964117946888929822, -64.24592483216726180, 170.0000000000000000 ) ) ;
#64617=ORIENTED_EDGE ( 'NONE', *, *, #20976, .T. ) ;
#64618=DIRECTION ( 'NONE',  ( 1.000000000000000000, 0.000000000000000000, 0.000000000000000000 ) ) ;
#64622=CARTESIAN_POINT ( 'NONE',  ( 24.79066879238614263, -3.228426989449305839, 0.000000000000000000 ) ) ;
#64636=DIRECTION ( 'NONE',  ( -0.04486483035051863633, 0.9989930665413144784, 0.000000000000000000 ) ) ;
#64645=CIRCLE ( 'NONE', #45561, 65.36598343705435354 ) ;
#64647=AXIS2_PLACEMENT_3D ( 'NONE', #69432, #37417, #54274 ) ;
#64658=DIRECTION ( 'NONE',  ( -0.000000000000000000, -0.000000000000000000, -1.000000000000000000 ) ) ;
#64666=DIRECTION ( 'NONE',  ( 0.8805955318567391110, -0.4738686624729965824, 0.000000000000000000 ) ) ;
#64668=VERTEX_POINT ( 'NONE', #14982 ) ;
#64669=B_SPLINE_CURVE_WITH_KNOTS ( 'NONE', 3,
 ( #240, #38577, #49109, #1298, #948, #32609 ),
 .UNSPECIFIED., .F., .F.,
 ( 4, 2, 4 ),
 ( 1.095770181108978510E-06, 0.03239442681617710207, 0.06478775786217309818 ),
 .UNSPECIFIED. ) ;
#64670=CARTESIAN_POINT ( 'NONE',  ( -31.86613092031432259, -10.09122378784736540, 6.893342932236730114 ) ) ;
#64672=CARTESIAN_POINT ( 'NONE',  ( 0.000000000000000000, 0.000000000000000000, 41.38025477438755928 ) ) ;
#64678=ORIENTED_EDGE ( 'NONE', *, *, #30052, .T. ) ;
#64681=AXIS2_PLACEMENT_3D ( 'NONE', #66646, #54670, #38866 ) ;
#64685=PLANE ( 'NONE',  #40410 ) ;
#64686=CARTESIAN_POINT ( 'NONE',  ( 0.000000000000000000, 0.000000000000000000, 40.00000000000003553 ) ) ;
#64687=DIRECTION ( 'NONE',  ( 1.000000000000000000, 0.000000000000000000, 0.000000000000000000 ) ) ;
#64690=AXIS2_PLACEMENT_3D ( 'NONE', #34605, #18403, #34247 ) ;
#64710=CARTESIAN_POINT ( 'NONE',  ( 24.46491470961361614, -5.710143558202974923, 0.000000000000000000 ) ) ;
#64714=ORIENTED_EDGE ( 'NONE', *, *, #17571, .T. ) ;
#64722=CARTESIAN_POINT ( 'NONE',  ( 0.000000000000000000, 0.000000000000000000, 0.000000000000000000 ) ) ;
#64724=CIRCLE ( 'NONE', #37750, 65.00000000000000000 ) ;
#64728=ORIENTED_EDGE ( 'NONE', *, *, #469, .F. ) ;
#64731=AXIS2_PLACEMENT_3D ( 'NONE', #68853, #20679, #63598 ) ;
#64735=VECTOR ( 'NONE', #434, 1000.000000000000000 ) ;
#64736=AXIS2_PLACEMENT_3D ( 'NONE', #5039, #31776, #44047 ) ;
#64742=CARTESIAN_POINT ( 'NONE',  ( 24.46491470961352732, 5.710143558203322200, 3.061616997868437868E-16 ) ) ;
#64743=VERTEX_POINT ( 'NONE', #13607 ) ;
#64749=EDGE_LOOP ( 'NONE', ( #25288, #15657, #48851, #40107, #56841, #15843, #2777, #17499, #29027 ) ) ;
#64751=LINE ( 'NONE', #733, #67224 ) ;
#64759=ORIENTED_EDGE ( 'NONE', *, *, #61583, .F. ) ;
#64761=CARTESIAN_POINT ( 'NONE',  ( 14.59045944429412600, 20.30070179093326743, 0.000000000000000000 ) ) ;
#64763=DIRECTION ( 'NONE',  ( -0.000000000000000000, -0.000000000000000000, -1.000000000000000000 ) ) ;
#64769=DIRECTION ( 'NONE',  ( -0.000000000000000000, -0.000000000000000000, -1.000000000000000000 ) ) ;
#64779=CIRCLE ( 'NONE', #64731, 65.00000000000000000 ) ;
#64786=VECTOR ( 'NONE', #48542, 1000.000000000000000 ) ;
#64804=B_SPLINE_CURVE_WITH_KNOTS ( 'NONE', 3,
 ( #36409, #10353, #20919, #42372 ),
 .UNSPECIFIED., .F., .F.,
 ( 4, 4 ),
 ( 9.900409499183408838E-07, 0.05658314289920114704 ),
 .UNSPECIFIED. ) ;
#64833=CARTESIAN_POINT ( 'NONE',  ( -15.76129977463530274, 63.43731725181437042, 43.58025477438756212 ) ) ;
#64847=ORIENTED_EDGE ( 'NONE', *, *, #59049, .F. ) ;
#64852=EDGE_CURVE ( 'NONE', #62854, #57856, #20599, .T. ) ;
#64858=ADVANCED_FACE ( 'NONE', ( #37127 ), #59265, .T. ) ;
#64871=ORIENTED_EDGE ( 'NONE', *, *, #47863, .F. ) ;
#64888=VECTOR ( 'NONE', #65457, 1000.000000000000000 ) ;
#64892=CYLINDRICAL_SURFACE ( 'NONE', #35324, 65.00000000000000000 ) ;
#64897=CARTESIAN_POINT ( 'NONE',  ( -74.81012118577224612, 5.477980300262961677, 170.0000000000000000 ) ) ;
#64900=CARTESIAN_POINT ( 'NONE',  ( 0.000000000000000000, 0.000000000000000000, 170.0000000000000000 ) ) ;
#64907=ORIENTED_EDGE ( 'NONE', *, *, #51043, .T. ) ;
#64914=CYLINDRICAL_SURFACE ( 'NONE', #14470, 65.00000000000000000 ) ;
#64915=ORIENTED_EDGE ( 'NONE', *, *, #30493, .T. ) ;
#64934=LINE ( 'NONE', #43455, #2729 ) ;
#64938=DIRECTION ( 'NONE',  ( -0.000000000000000000, -0.000000000000000000, -1.000000000000000000 ) ) ;
#64943=PLANE ( 'NONE',  #54412 ) ;
#64956=CARTESIAN_POINT ( 'NONE',  ( 10.73115448446747244, -22.57968829347487727, 0.000000000000000000 ) ) ;
#64964=CARTESIAN_POINT ( 'NONE',  ( -58.00979178563853367, 29.32343869649098878, 40.00000000000003553 ) ) ;
#64971=DIRECTION ( 'NONE',  ( 1.000000000000000000, 0.000000000000000000, 0.000000000000000000 ) ) ;
#64983=AXIS2_PLACEMENT_3D ( 'NONE', #5290, #53457, #32717 ) ;
#64987=PLANE ( 'NONE',  #3991 ) ;
#64994=CARTESIAN_POINT ( 'NONE',  ( -41.65447218327533818, -2.493917879428980910, 13.79046340968178441 ) ) ;
#65004=FACE_OUTER_BOUND ( 'NONE', #5718, .T. ) ;
#65008=VERTEX_POINT ( 'NONE', #24089 ) ;
#65015=CARTESIAN_POINT ( 'NONE',  ( -25.87147652227456263, 100.0000000000000000, 129.5802547743875550 ) ) ;
#65024=AXIS2_PLACEMENT_3D ( 'NONE', #56095, #24446, #40954 ) ;
#65031=FACE_OUTER_BOUND ( 'NONE', #42853, .T. ) ;
#65051=CARTESIAN_POINT ( 'NONE',  ( -16.35146342289083776, -18.91109843266265500, 0.000000000000000000 ) ) ;
#65052=VERTEX_POINT ( 'NONE', #24776 ) ;
#65060=DIRECTION ( 'NONE',  ( -1.000000000000000000, 0.000000000000000000, 0.000000000000000000 ) ) ;
#65067=CARTESIAN_POINT ( 'NONE',  ( -1.666933348992582609, 64.97862212458815634, 170.0000000000000000 ) ) ;
#65072=ORIENTED_EDGE ( 'NONE', *, *, #36509, .T. ) ;
#65075=VECTOR ( 'NONE', #15006, 1000.000000000000000 ) ;
#65081=DIRECTION ( 'NONE',  ( -0.9009688679024155933, -0.4338837391175656699, 0.000000000000000000 ) ) ;
#65091=CIRCLE ( 'NONE', #44866, 25.12245591505646303 ) ;
#65094=CARTESIAN_POINT ( 'NONE',  ( 0.000000000000000000, 0.000000000000000000, 0.000000000000000000 ) ) ;
#65095=ORIENTED_EDGE ( 'NONE', *, *, #68923, .F. ) ;
#65097=EDGE_CURVE ( 'NONE', #26073, #14985, #35335, .T. ) ;
#65101=EDGE_CURVE ( 'NONE', #55398, #60669, #19039, .T. ) ;
#65102=CARTESIAN_POINT ( 'NONE',  ( -17.89459634713148262, 72.78390022947087346, 41.38025477438755928 ) ) ;
#65103=DIRECTION ( 'NONE',  ( 1.000000000000000000, 0.000000000000000000, 0.000000000000000000 ) ) ;
#65122=CARTESIAN_POINT ( 'NONE',  ( 74.94097818310312675, -1.250000000000021760, 41.38025477438755928 ) ) ;
#65129=EDGE_CURVE ( 'NONE', #53544, #43521, #37018, .T. ) ;
#65130=VECTOR ( 'NONE', #14494, 1000.000000000000000 ) ;
#65135=VECTOR ( 'NONE', #46477, 1000.000000000000000 ) ;
#65140=EDGE_LOOP ( 'NONE', ( #18474, #56540, #60008, #2359 ) ) ;
#65152=DIRECTION ( 'NONE',  ( 0.6910626489868685329, -0.7227948638273878901, 0.000000000000000000 ) ) ;
#65154=CARTESIAN_POINT ( 'NONE',  ( -18.89790202299119315, -62.20684691518632548, 170.0000000000000000 ) ) ;
#65158=ORIENTED_EDGE ( 'NONE', *, *, #14685, .F. ) ;
#65166=EDGE_CURVE ( 'NONE', #634, #19763, #36713, .T. ) ;
#65167=ORIENTED_EDGE ( 'NONE', *, *, #27091, .F. ) ;
#65171=ORIENTED_EDGE ( 'NONE', *, *, #35244, .F. ) ;
#65172=FACE_OUTER_BOUND ( 'NONE', #58947, .T. ) ;
#65182=CARTESIAN_POINT ( 'NONE',  ( 9.962235950565768050, -64.23203137738408941, 170.0000000000000000 ) ) ;
#65189=DIRECTION ( 'NONE',  ( -1.000000000000000000, 0.000000000000000000, 0.000000000000000000 ) ) ;
#65194=CIRCLE ( 'NONE', #11254, 65.00000000000000000 ) ;
#65198=CARTESIAN_POINT ( 'NONE',  ( 4.549306917177319498, -73.43672186181514405, 73.58025477438755502 ) ) ;
#65205=FACE_OUTER_BOUND ( 'NONE', #67657, .T. ) ;
#65209=EDGE_CURVE ( 'NONE', #67138, #33038, #69401, .T. ) ;
#65216=LINE ( 'NONE', #44449, #49502 ) ;
#65229=DIRECTION ( 'NONE',  ( 1.000000000000000000, -1.509903313490212895E-14, 0.000000000000000000 ) ) ;
#65233=CARTESIAN_POINT ( 'NONE',  ( 0.000000000000000000, 0.000000000000000000, 0.000000000000000000 ) ) ;
#65237=CARTESIAN_POINT ( 'NONE',  ( 41.49663191311417165, -50.03028622612021792, 40.00000000000003553 ) ) ;
#65257=DIRECTION ( 'NONE',  ( 0.04486483035050447404, 0.9989930665413151445, 0.000000000000000000 ) ) ;
#65261=DIRECTION ( 'NONE',  ( -0.9639628606958512425, -0.2660368455666826670, 0.000000000000000000 ) ) ;
#65269=PLANE ( 'NONE',  #10208 ) ;
#65271=LINE ( 'NONE', #42762, #54485 ) ;
#65278=LINE ( 'NONE', #17072, #63746 ) ;
#65279=PLANE ( 'NONE',  #28739 ) ;
#65288=EDGE_CURVE ( 'NONE', #64530, #40830, #4477, .T. ) ;
#65295=ADVANCED_FACE ( 'NONE', ( #6423 ), #27877, .F. ) ;
#65296=EDGE_CURVE ( 'NONE', #55255, #32221, #44399, .T. ) ;
#65299=CYLINDRICAL_SURFACE ( 'NONE', #18004, 65.00000000000000000 ) ;
#65309=CARTESIAN_POINT ( 'NONE',  ( 9.962235950564870990, 64.23203137738423152, 73.58025477438756923 ) ) ;
#65315=AXIS2_PLACEMENT_3D ( 'NONE', #36673, #37341, #15561 ) ;
#65316=PLANE ( 'NONE',  #66396 ) ;
#65322=CARTESIAN_POINT ( 'NONE',  ( 0.000000000000000000, 0.000000000000000000, 43.58025477438756212 ) ) ;
#65323=CARTESIAN_POINT ( 'NONE',  ( 39.54205320694412507, -51.58901073076707888, 40.00000000000003553 ) ) ;
#65331=LINE ( 'NONE', #5875, #48838 ) ;
#65337=CARTESIAN_POINT ( 'NONE',  ( -25.10237775011639982, -1.004202417053851937, 0.000000000000000000 ) ) ;
#65345=DIRECTION ( 'NONE',  ( -1.000000000000000000, 0.000000000000000000, 0.000000000000000000 ) ) ;
#65349=AXIS2_PLACEMENT_3D ( 'NONE', #31192, #41399, #8700 ) ;
#65352=EDGE_CURVE ( 'NONE', #60210, #25097, #38078, .T. ) ;
#65354=EDGE_CURVE ( 'NONE', #30082, #36722, #50527, .T. ) ;
#65356=CONICAL_SURFACE ( 'NONE', #49617, 74.95140232871122521, 0.8777644062502172329 ) ;
#65359=ORIENTED_EDGE ( 'NONE', *, *, #58057, .T. ) ;
#65371=DIRECTION ( 'NONE',  ( -0.000000000000000000, -0.000000000000000000, -1.000000000000000000 ) ) ;
#65391=LINE ( 'NONE', #672, #10553 ) ;
#65393=ORIENTED_EDGE ( 'NONE', *, *, #50012, .F. ) ;
#65404=VERTEX_POINT ( 'NONE', #62314 ) ;
#65406=EDGE_LOOP ( 'NONE', ( #62006, #67872, #29911, #46442, #34195, #24442, #32700, #15064, #66601 ) ) ;
#65432=LINE ( 'NONE', #38699, #31861 ) ;
#65434=ADVANCED_FACE ( 'NONE', ( #45090 ), #19753, .T. ) ;
#65437=B_SPLINE_CURVE_WITH_KNOTS ( 'NONE', 3,
 ( #58044, #16161, #15486, #59067 ),
 .UNSPECIFIED., .F., .F.,
 ( 4, 4 ),
 ( 0.1259919275528359750, 0.1829744153748750768 ),
 .UNSPECIFIED. ) ;
#65445=DIRECTION ( 'NONE',  ( -1.084727855779412860E-16, 2.252460601983934209E-16, 1.000000000000000000 ) ) ;
#65448=AXIS2_PLACEMENT_3D ( 'NONE', #23862, #8022, #18576 ) ;
#65450=FACE_OUTER_BOUND ( 'NONE', #28905, .T. ) ;
#65457=DIRECTION ( 'NONE',  ( 0.000000000000000000, 0.000000000000000000, 1.000000000000000000 ) ) ;
#65458=DIRECTION ( 'NONE',  ( -1.000000000000000000, 0.000000000000000000, 0.000000000000000000 ) ) ;
#65459=EDGE_LOOP ( 'NONE', ( #31386, #52461, #2997, #37685 ) ) ;
#65463=AXIS2_PLACEMENT_3D ( 'NONE', #6101, #32843, #54987 ) ;
#65468=CARTESIAN_POINT ( 'NONE',  ( 43.69793103685474023, 27.56441319423685243, 26.66469066592269499 ) ) ;
#65473=DIRECTION ( 'NONE',  ( -0.000000000000000000, -0.000000000000000000, -1.000000000000000000 ) ) ;
#65481=LINE ( 'NONE', #23273, #46706 ) ;
#65494=CARTESIAN_POINT ( 'NONE',  ( -37.03736084664572559, -19.22364826157912177, 13.79046412329102544 ) ) ;
#65498=VERTEX_POINT ( 'NONE', #19402 ) ;
#65505=CARTESIAN_POINT ( 'NONE',  ( -49.77357484059193382, 41.82599373102802787, 41.38025477438755928 ) ) ;
#65509=AXIS2_PLACEMENT_3D ( 'NONE', #35758, #52267, #13945 ) ;
#65510=EDGE_CURVE ( 'NONE', #38709, #39038, #46133, .T. ) ;
#65515=ADVANCED_FACE ( 'NONE', ( #57050 ), #8864, .T. ) ;
#65525=ORIENTED_EDGE ( 'NONE', *, *, #68082, .F. ) ;
#65526=CARTESIAN_POINT ( 'NONE',  ( 56.48035995027147749, -49.34540444547771187, 43.58025477438756212 ) ) ;
#65530=ORIENTED_EDGE ( 'NONE', *, *, #32383, .F. ) ;
#65547=ORIENTED_EDGE ( 'NONE', *, *, #6364, .F. ) ;
#65551=FACE_OUTER_BOUND ( 'NONE', #52641, .T. ) ;
#65555=VECTOR ( 'NONE', #41514, 1000.000000000000114 ) ;
#65557=AXIS2_PLACEMENT_3D ( 'NONE', #54676, #60660, #65601 ) ;
#65558=FACE_OUTER_BOUND ( 'NONE', #38707, .T. ) ;
#65560=CARTESIAN_POINT ( 'NONE',  ( 7.705764017935865517, 66.19838207530922602, 34.48241823979987686 ) ) ;
#65562=CONICAL_SURFACE ( 'NONE', #22873, 65.00000000000000000, 0.7853981633974497223 ) ;
#65571=DIRECTION ( 'NONE',  ( -0.9909497617679331460, -0.1342332658176667304, 0.000000000000000000 ) ) ;
#65572=CARTESIAN_POINT ( 'NONE',  ( 8.904582680624310242, -23.36040254969760355, 0.000000000000000000 ) ) ;
#65574=ORIENTED_EDGE ( 'NONE', *, *, #57350, .T. ) ;
#65575=ORIENTED_EDGE ( 'NONE', *, *, #12015, .F. ) ;
#65578=DIRECTION ( 'NONE',  ( 1.000000000000000000, 0.000000000000000000, 0.000000000000000000 ) ) ;
#65587=CARTESIAN_POINT ( 'NONE',  ( -65.00200000000002376, -1.250000000000021760, 43.58025477438756923 ) ) ;
#65590=CARTESIAN_POINT ( 'NONE',  ( 61.91366885787816443, -28.42865614898931881, 170.0000000000000000 ) ) ;
#65592=CARTESIAN_POINT ( 'NONE',  ( 55.14772863908675049, -34.40534879854660488, 170.0000000000000000 ) ) ;
#65596=VECTOR ( 'NONE', #35250, 1000.000000000000000 ) ;
#65597=EDGE_CURVE ( 'NONE', #1913, #59098, #47500, .T. ) ;
#65598=ORIENTED_EDGE ( 'NONE', *, *, #32385, .F. ) ;
#65600=EDGE_CURVE ( 'NONE', #28345, #48432, #30658, .T. ) ;
#65601=DIRECTION ( 'NONE',  ( -1.000000000000000000, 0.000000000000000000, 0.000000000000000000 ) ) ;
#65606=VECTOR ( 'NONE', #23099, 1000.000000000000227 ) ;
#65608=ORIENTED_EDGE ( 'NONE', *, *, #35967, .F. ) ;
#65609=VECTOR ( 'NONE', #25789, 1000.000000000000227 ) ;
#65612=DIRECTION ( 'NONE',  ( 1.000000000000000000, 0.000000000000000000, 0.000000000000000000 ) ) ;
#65615=CIRCLE ( 'NONE', #22929, 65.36598343705435354 ) ;
#65624=PLANE ( 'NONE',  #6625 ) ;
#65630=DIRECTION ( 'NONE',  ( -0.1342332658176522420, -0.9909497617679351444, 0.000000000000000000 ) ) ;
#65644=CARTESIAN_POINT ( 'NONE',  ( -46.45214378727172999, -35.29454295034832256, 27.58472369410210234 ) ) ;
#65646=EDGE_LOOP ( 'NONE', ( #8702, #44458, #16685, #14997 ) ) ;
#65649=CARTESIAN_POINT ( 'NONE',  ( -72.29721455218913206, 19.95276341750015803, 43.58025477438756212 ) ) ;
#65650=DIRECTION ( 'NONE',  ( 8.784520486428009340E-17, -2.340627113153416505E-16, 1.000000000000000000 ) ) ;
#65656=DIRECTION ( 'NONE',  ( -0.5508969814520944253, -0.8345732537213078617, 0.000000000000000000 ) ) ;
#65662=VECTOR ( 'NONE', #24187, 1000.000000000000000 ) ;
#65664=VERTEX_POINT ( 'NONE', #47166 ) ;
#65667=AXIS2_PLACEMENT_3D ( 'NONE', #31190, #43097, #31866 ) ;
#65671=DIRECTION ( 'NONE',  ( 1.000000000000000000, 0.000000000000000000, 0.000000000000000000 ) ) ;
#65673=CARTESIAN_POINT ( 'NONE',  ( 0.000000000000000000, 0.000000000000000000, 43.58025477438756212 ) ) ;
#65682=LINE ( 'NONE', #49825, #12010 ) ;
#65693=ORIENTED_EDGE ( 'NONE', *, *, #29612, .F. ) ;
#65705=EDGE_CURVE ( 'NONE', #36843, #34467, #25735, .T. ) ;
#65737=ADVANCED_FACE ( 'NONE', ( #65004 ), #16797, .T. ) ;
#65740=CARTESIAN_POINT ( 'NONE',  ( 61.91366885787727625, 28.42865614899003290, 170.0000000000000000 ) ) ;
#65744=ADVANCED_FACE ( 'NONE', ( #12580 ), #50906, .F. ) ;
#65756=VECTOR ( 'NONE', #44368, 1000.000000000000000 ) ;
#65760=CARTESIAN_POINT ( 'NONE',  ( -25.57361468187733422, -28.55671243481888055, 13.32819299319723783 ) ) ;
#65762=LINE ( 'NONE', #55894, #31959 ) ;
#65763=CARTESIAN_POINT ( 'NONE',  ( -1.666933348991701536, -64.97862212458815634, 40.00000000000003553 ) ) ;
#65777=ORIENTED_EDGE ( 'NONE', *, *, #65600, .F. ) ;
#65781=CARTESIAN_POINT ( 'NONE',  ( -30.62628708973294422, -68.47330165179167238, 170.0000000000000000 ) ) ;
#65787=VERTEX_POINT ( 'NONE', #40002 ) ;
#65789=DIRECTION ( 'NONE',  ( -0.000000000000000000, -0.000000000000000000, -1.000000000000000000 ) ) ;
#65795=VERTEX_POINT ( 'NONE', #13615 ) ;
#65796=EDGE_CURVE ( 'NONE', #62016, #55532, #58388, .T. ) ;
#65802=B_SPLINE_CURVE_WITH_KNOTS ( 'NONE', 3,
 ( #16616, #37728, #48262, #53548 ),
 .UNSPECIFIED., .F., .F.,
 ( 4, 4 ),
 ( 0.1259919275528358362, 0.1829744153748747437 ),
 .UNSPECIFIED. ) ;
#65804=CIRCLE ( 'NONE', #23116, 65.00000000000000000 ) ;
#65808=DIRECTION ( 'NONE',  ( 0.1342332658176667304, -0.9909497617679331460, 0.000000000000000000 ) ) ;
#65809=VECTOR ( 'NONE', #26754, 1000.000000000000227 ) ;
#65811=VECTOR ( 'NONE', #19163, 1000.000000000000000 ) ;
#65812=DIRECTION ( 'NONE',  ( -0.000000000000000000, -0.000000000000000000, 1.000000000000000000 ) ) ;
#65820=CARTESIAN_POINT ( 'NONE',  ( -48.12872802574265307, 43.70867239603709464, 41.38025477438755928 ) ) ;
#65830=CARTESIAN_POINT ( 'NONE',  ( 20.79325243092023001, -13.87950479462515396, 0.000000000000000000 ) ) ;
#65836=ADVANCED_FACE ( 'NONE', ( #13960 ), #14994, .T. ) ;
#65843=CARTESIAN_POINT ( 'NONE',  ( 23.05216796272351232, -9.986758404123879274, 0.000000000000000000 ) ) ;
#65848=VERTEX_POINT ( 'NONE', #61797 ) ;
#65850=EDGE_CURVE ( 'NONE', #41788, #56234, #20238, .T. ) ;
#65854=AXIS2_PLACEMENT_3D ( 'NONE', #5415, #43382, #59210 ) ;
#65862=EDGE_CURVE ( 'NONE', #40678, #37904, #18987, .T. ) ;
#65864=CIRCLE ( 'NONE', #60264, 65.00000000000000000 ) ;
#65868=CARTESIAN_POINT ( 'NONE',  ( 0.000000000000000000, 0.000000000000000000, 43.58025477438756212 ) ) ;
#65874=VECTOR ( 'NONE', #25758, 1000.000000000000114 ) ;
#65876=EDGE_LOOP ( 'NONE', ( #49573, #20406, #35766, #62857 ) ) ;
#65879=DIRECTION ( 'NONE',  ( -1.000000000000000000, 0.000000000000000000, 0.000000000000000000 ) ) ;
#65882=DIRECTION ( 'NONE',  ( 1.000000000000000000, 0.000000000000000000, 0.000000000000000000 ) ) ;
#65883=ORIENTED_EDGE ( 'NONE', *, *, #43046, .F. ) ;
#65884=EDGE_CURVE ( 'NONE', #19391, #58062, #25875, .T. ) ;
#65885=CARTESIAN_POINT ( 'NONE',  ( -61.41100614348627573, -43.07262267896732766, 170.0000000000000000 ) ) ;
#65887=ORIENTED_EDGE ( 'NONE', *, *, #51856, .T. ) ;
#65889=EDGE_LOOP ( 'NONE', ( #11307, #65393, #56123, #2202 ) ) ;
#65895=DIRECTION ( 'NONE',  ( -0.000000000000000000, -0.000000000000000000, -1.000000000000000000 ) ) ;
#65899=CARTESIAN_POINT ( 'NONE',  ( 10.78925482157266913, -22.68765681156003566, 0.000000000000000000 ) ) ;
#65901=DIRECTION ( 'NONE',  ( -0.9639628606958512425, -0.2660368455666826670, 0.000000000000000000 ) ) ;
#65910=VERTEX_POINT ( 'NONE', #51602 ) ;
#65911=ORIENTED_EDGE ( 'NONE', *, *, #40488, .F. ) ;
#65912=VECTOR ( 'NONE', #56087, 1000.000000000000000 ) ;
#65914=ORIENTED_EDGE ( 'NONE', *, *, #56052, .F. ) ;
#65918=DIRECTION ( 'NONE',  ( 0.08963930890342654279, 0.9959742939952397345, -0.000000000000000000 ) ) ;
#65919=FACE_OUTER_BOUND ( 'NONE', #32121, .T. ) ;
#65920=EDGE_CURVE ( 'NONE', #63617, #56134, #56887, .T. ) ;
#65929=CARTESIAN_POINT ( 'NONE',  ( -36.60035584460344893, -11.39778684791367702, 13.32819299319725026 ) ) ;
#65930=EDGE_LOOP ( 'NONE', ( #51666, #29105, #12881, #45133, #45356 ) ) ;
#65937=DIRECTION ( 'NONE',  ( -1.000000000000000000, 0.000000000000000000, 0.000000000000000000 ) ) ;
#65939=ORIENTED_EDGE ( 'NONE', *, *, #39483, .T. ) ;
#65942=DIRECTION ( 'NONE',  ( -0.000000000000000000, -0.000000000000000000, -1.000000000000000000 ) ) ;
#65950=ORIENTED_EDGE ( 'NONE', *, *, #2444, .T. ) ;
#65969=VERTEX_POINT ( 'NONE', #38173 ) ;
#65974=VERTEX_POINT ( 'NONE', #26589 ) ;
#65982=CARTESIAN_POINT ( 'NONE',  ( 11.30618213853385967, 74.15344055032308290, 170.0000000000000000 ) ) ;
#65983=CARTESIAN_POINT ( 'NONE',  ( 69.72313848477121212, 27.50266661387133738, 41.38025477438755928 ) ) ;
#66000=EDGE_CURVE ( 'NONE', #15856, #55870, #58431, .T. ) ;
#66015=CARTESIAN_POINT ( 'NONE',  ( 0.000000000000000000, 0.000000000000000000, 41.38025477438755928 ) ) ;
#66019=VECTOR ( 'NONE', #28508, 1000.000000000000000 ) ;
#66023=VERTEX_POINT ( 'NONE', #1243 ) ;
#66025=VERTEX_POINT ( 'NONE', #50478 ) ;
#66026=CARTESIAN_POINT ( 'NONE',  ( 0.000000000000000000, 0.000000000000000000, 40.00000000000003553 ) ) ;
#66027=VECTOR ( 'NONE', #67984, 1000.000000000000000 ) ;
#66030=EDGE_CURVE ( 'NONE', #26757, #40830, #12498, .T. ) ;
#66031=CARTESIAN_POINT ( 'NONE',  ( -30.26163407093831381, -23.53144909134785578, 13.32819299319723605 ) ) ;
#66042=CARTESIAN_POINT ( 'NONE',  ( 0.000000000000000000, 0.000000000000000000, 0.000000000000000000 ) ) ;
#66054=VECTOR ( 'NONE', #51260, 1000.000000000000114 ) ;
#66058=CARTESIAN_POINT ( 'NONE',  ( 0.000000000000000000, 0.000000000000000000, 40.00000000000003553 ) ) ;
#66063=VECTOR ( 'NONE', #34725, 999.9999999999998863 ) ;
#66071=ORIENTED_EDGE ( 'NONE', *, *, #67282, .F. ) ;
#66077=VERTEX_POINT ( 'NONE', #22350 ) ;
#66082=DIRECTION ( 'NONE',  ( 1.000000000000000000, 0.000000000000000000, 0.000000000000000000 ) ) ;
#66083=ADVANCED_FACE ( 'NONE', ( #33958 ), #65624, .T. ) ;
#66086=DIRECTION ( 'NONE',  ( -0.000000000000000000, -0.000000000000000000, -1.000000000000000000 ) ) ;
#66087=CARTESIAN_POINT ( 'NONE',  ( 0.000000000000000000, 0.000000000000000000, 41.38025477438755928 ) ) ;
#66096=DIRECTION ( 'NONE',  ( 1.000000000000000000, 0.000000000000000000, 0.000000000000000000 ) ) ;
#66097=DIRECTION ( 'NONE',  ( 0.6234898018587431423, -0.7818314824680220321, 0.000000000000000000 ) ) ;
#66100=ORIENTED_EDGE ( 'NONE', *, *, #33150, .T. ) ;
#66102=ORIENTED_EDGE ( 'NONE', *, *, #39483, .F. ) ;
#66105=DIRECTION ( 'NONE',  ( 0.000000000000000000, 0.000000000000000000, 1.000000000000000000 ) ) ;
#66108=DIRECTION ( 'NONE',  ( -0.000000000000000000, -0.000000000000000000, -1.000000000000000000 ) ) ;
#66109=EDGE_CURVE ( 'NONE', #24416, #34646, #60682, .T. ) ;
#66120=DIRECTION ( 'NONE',  ( -0.9839295885986321100, 0.1785568947986229116, 0.000000000000000000 ) ) ;
#66124=ORIENTED_EDGE ( 'NONE', *, *, #44151, .T. ) ;
#66125=CARTESIAN_POINT ( 'NONE',  ( 2.051824250824011653, -73.54888393769144272, 73.58025477438755502 ) ) ;
#66128=ORIENTED_EDGE ( 'NONE', *, *, #14938, .T. ) ;
#66138=DIRECTION ( 'NONE',  ( -0.6579387259397136978, 0.7530714660036099684, 2.500042656554810340E-16 ) ) ;
#66139=FACE_OUTER_BOUND ( 'NONE', #21685, .T. ) ;
#66141=FACE_OUTER_BOUND ( 'NONE', #32904, .T. ) ;
#66151=CARTESIAN_POINT ( 'NONE',  ( 6.837602017663892973, -41.16505738580269735, 13.79046412288134249 ) ) ;
#66186=PLANE ( 'NONE',  #44491 ) ;
#66193=ORIENTED_EDGE ( 'NONE', *, *, #43009, .T. ) ;
#66194=DIRECTION ( 'NONE',  ( 1.000000000000000000, 0.000000000000000000, 0.000000000000000000 ) ) ;
#66195=ORIENTED_EDGE ( 'NONE', *, *, #61211, .T. ) ;
#66197=EDGE_CURVE ( 'NONE', #24194, #11802, #25982, .T. ) ;
#66204=EDGE_CURVE ( 'NONE', #49653, #9355, #25143, .T. ) ;
#66213=DIRECTION ( 'NONE',  ( 1.000000000000000000, 0.000000000000000000, -0.000000000000000000 ) ) ;
#66214=CARTESIAN_POINT ( 'NONE',  ( -29.55217150403795401, -15.61897105721054757, 6.893342933764143865 ) ) ;
#66215=CARTESIAN_POINT ( 'NONE',  ( -48.12872802574198516, -43.70867239603780519, 41.38025477438755928 ) ) ;
#66223=DIRECTION ( 'NONE',  ( -0.000000000000000000, -0.000000000000000000, -1.000000000000000000 ) ) ;
#66224=DIRECTION ( 'NONE',  ( 0.7530714660036196273, -0.6579387259397027066, 0.000000000000000000 ) ) ;
#66229=CARTESIAN_POINT ( 'NONE',  ( 0.000000000000000000, 0.000000000000000000, 43.58025477438756212 ) ) ;
#66233=CARTESIAN_POINT ( 'NONE',  ( 0.000000000000000000, 0.000000000000000000, 170.0000000000000000 ) ) ;
#66237=VERTEX_POINT ( 'NONE', #19855 ) ;
#66245=ORIENTED_EDGE ( 'NONE', *, *, #7211, .T. ) ;
#66253=EDGE_CURVE ( 'NONE', #53230, #16637, #2993, .T. ) ;
#66263=CARTESIAN_POINT ( 'NONE',  ( -67.57266509268116295, -32.54128043381741975, 0.000000000000000000 ) ) ;
#66265=ORIENTED_EDGE ( 'NONE', *, *, #31450, .T. ) ;
#66268=CARTESIAN_POINT ( 'NONE',  ( -17.89459634713148262, 72.78390022947087346, 41.38025477438755928 ) ) ;
#66272=CARTESIAN_POINT ( 'NONE',  ( -2.116120943111181152, -74.98056102853681182, 43.58025477438756923 ) ) ;
#66275=CARTESIAN_POINT ( 'NONE',  ( 21.27121078971612889, 61.42097029141972087, 170.0000000000000000 ) ) ;
#66284=VECTOR ( 'NONE', #4979, 1000.000000000000114 ) ;
#66290=DIRECTION ( 'NONE',  ( -1.000000000000000000, 0.000000000000000000, 0.000000000000000000 ) ) ;
#66293=EDGE_LOOP ( 'NONE', ( #18056, #11294, #44039, #40414, #31590, #43948, #22792, #26712, #48238 ) ) ;
#66310=DIRECTION ( 'NONE',  ( -1.000000000000000000, 0.000000000000000000, 0.000000000000000000 ) ) ;
#66318=AXIS2_PLACEMENT_3D ( 'NONE', #38255, #28051, #44222 ) ;
#66325=ORIENTED_EDGE ( 'NONE', *, *, #42021, .T. ) ;
#66330=VERTEX_POINT ( 'NONE', #64833 ) ;
#66340=B_SPLINE_CURVE_WITH_KNOTS ( 'NONE', 3,
 ( #44078, #23356, #65929, #11376 ),
 .UNSPECIFIED., .F., .F.,
 ( 4, 4 ),
 ( 9.900409499190005107E-07, 0.05658314289920114010 ),
 .UNSPECIFIED. ) ;
#66357=DIRECTION ( 'NONE',  ( -1.000000000000000000, 0.000000000000000000, 0.000000000000000000 ) ) ;
#66361=ORIENTED_EDGE ( 'NONE', *, *, #31396, .F. ) ;
#66364=CARTESIAN_POINT ( 'NONE',  ( -8.712114576423861223, 23.56346432108866651, 0.000000000000000000 ) ) ;
#66366=DIRECTION ( 'NONE',  ( -0.000000000000000000, -0.000000000000000000, -1.000000000000000000 ) ) ;
#66371=ORIENTED_EDGE ( 'NONE', *, *, #18423, .F. ) ;
#66381=VECTOR ( 'NONE', #28729, 1000.000000000000227 ) ;
#66386=DIRECTION ( 'NONE',  ( -0.04486483035050447404, -0.9989930665413151445, 0.000000000000000000 ) ) ;
#66389=DIRECTION ( 'NONE',  ( 0.000000000000000000, 0.000000000000000000, 1.000000000000000000 ) ) ;
#66396=AXIS2_PLACEMENT_3D ( 'NONE', #17102, #33317, #31923 ) ;
#66406=ADVANCED_FACE ( 'NONE', ( #11351 ), #16973, .T. ) ;
#66410=EDGE_LOOP ( 'NONE', ( #43199, #17894, #51266, #3658 ) ) ;
#66411=DIRECTION ( 'NONE',  ( -0.000000000000000000, -0.000000000000000000, -1.000000000000000000 ) ) ;
#66421=FACE_OUTER_BOUND ( 'NONE', #42766, .T. ) ;
#66424=EDGE_CURVE ( 'NONE', #12796, #18218, #14146, .T. ) ;
#66440=VERTEX_POINT ( 'NONE', #9212 ) ;
#66442=VERTEX_POINT ( 'NONE', #62687 ) ;
#66463=ORIENTED_EDGE ( 'NONE', *, *, #55018, .F. ) ;
#66465=CARTESIAN_POINT ( 'NONE',  ( -31.90315521289150524, 56.64813493366005304, 170.0000000000000000 ) ) ;
#66466=FACE_OUTER_BOUND ( 'NONE', #20669, .T. ) ;
#66476=VERTEX_POINT ( 'NONE', #3936 ) ;
#66492=DIRECTION ( 'NONE',  ( -0.8345732537213079727, 0.5508969814520945363, 5.102127870520021999E-18 ) ) ;
#66495=VECTOR ( 'NONE', #5758, 1000.000000000000000 ) ;
#66503=EDGE_LOOP ( 'NONE', ( #68629, #58282, #17723, #5004 ) ) ;
#66507=EDGE_LOOP ( 'NONE', ( #60201, #67559, #56491, #36023 ) ) ;
#66508=CARTESIAN_POINT ( 'NONE',  ( -71.96466849523049802, -21.15771699337099321, 170.0000000000000000 ) ) ;
#66527=DIRECTION ( 'NONE',  ( 1.000000000000000000, 0.000000000000000000, 0.000000000000000000 ) ) ;
#66530=CIRCLE ( 'NONE', #54126, 65.00000000000000000 ) ;
#66532=AXIS2_PLACEMENT_3D ( 'NONE', #1757, #8067, #39045 ) ;
#66536=EDGE_LOOP ( 'NONE', ( #38867, #53896, #12338, #66991, #53056, #59035, #62845, #31774, #14786 ) ) ;
#66538=AXIS2_PLACEMENT_3D ( 'NONE', #25321, #21399, #42844 ) ;
#66541=DIRECTION ( 'NONE',  ( -0.000000000000000000, -0.000000000000000000, -1.000000000000000000 ) ) ;
#66564=ADVANCED_FACE ( 'NONE', ( #24712 ), #46145, .T. ) ;
#66576=ORIENTED_EDGE ( 'NONE', *, *, #57130, .F. ) ;
#66586=ORIENTED_EDGE ( 'NONE', *, *, #60925, .T. ) ;
#66588=DIRECTION ( 'NONE',  ( -0.9839295885986295565, -0.1785568947986370392, 0.000000000000000000 ) ) ;
#66594=DIRECTION ( 'NONE',  ( 0.000000000000000000, 0.000000000000000000, 1.000000000000000000 ) ) ;
#66601=ORIENTED_EDGE ( 'NONE', *, *, #7857, .F. ) ;
#66602=ORIENTED_EDGE ( 'NONE', *, *, #28194, .F. ) ;
#66612=CARTESIAN_POINT ( 'NONE',  ( -62.97854483871554976, -16.08424353203763957, 40.00000000000003553 ) ) ;
#66614=CARTESIAN_POINT ( 'NONE',  ( 0.000000000000000000, 0.000000000000000000, 170.0000000000000000 ) ) ;
#66615=ORIENTED_EDGE ( 'NONE', *, *, #4518, .T. ) ;
#66616=VERTEX_POINT ( 'NONE', #37655 ) ;
#66626=CIRCLE ( 'NONE', #23929, 65.36598343705435354 ) ;
#66627=ADVANCED_FACE ( 'NONE', ( #59108 ), #10920, .T. ) ;
#66629=CARTESIAN_POINT ( 'NONE',  ( -24.87827947785777383, -3.494138152041991408, 3.061616997868437868E-16 ) ) ;
#66630=CARTESIAN_POINT ( 'NONE',  ( -27.38060184144623221, 26.82905581235131010, 13.32819299319723250 ) ) ;
#66646=CARTESIAN_POINT ( 'NONE',  ( -25.87147652227456263, 70.00000000000000000, 77.58025477438755502 ) ) ;
#66648=ADVANCED_FACE ( 'NONE', ( #27443 ), #38354, .T. ) ;
#66656=DIRECTION ( 'NONE',  ( 0.5508969814520944253, 0.8345732537213078617, 0.000000000000000000 ) ) ;
#66657=CARTESIAN_POINT ( 'NONE',  ( -63.00000000000000000, 0.000000000000000000, 40.82842712474622004 ) ) ;
#66662=ORIENTED_EDGE ( 'NONE', *, *, #40444, .F. ) ;
#66672=EDGE_CURVE ( 'NONE', #33798, #42059, #27581, .T. ) ;
#66676=VECTOR ( 'NONE', #25615, 1000.000000000000114 ) ;
#66678=EDGE_CURVE ( 'NONE', #29753, #47253, #46404, .T. ) ;
#66679=ORIENTED_EDGE ( 'NONE', *, *, #56060, .T. ) ;
#66686=CARTESIAN_POINT ( 'NONE',  ( 70.65683382808232693, -25.18281821780010787, 43.58025477438756923 ) ) ;
#66688=DIRECTION ( 'NONE',  ( 0.9989930665413151445, -0.04486483035050447404, 2.500042656554809354E-16 ) ) ;
#66694=FACE_OUTER_BOUND ( 'NONE', #64595, .T. ) ;
#66703=CARTESIAN_POINT ( 'NONE',  ( 47.70222499156757578, 57.81185381817647340, 41.38025477438755928 ) ) ;
#66718=DIRECTION ( 'NONE',  ( 0.4338837391175526248, 0.9009688679024218105, -0.000000000000000000 ) ) ;
#66721=LINE ( 'NONE', #24501, #4553 ) ;
#66726=ORIENTED_EDGE ( 'NONE', *, *, #63546, .T. ) ;
#66735=VECTOR ( 'NONE', #61953, 1000.000000000000000 ) ;
#66754=CARTESIAN_POINT ( 'NONE',  ( 0.000000000000000000, 0.000000000000000000, 41.38025477438755928 ) ) ;
#66766=B_SPLINE_CURVE_WITH_KNOTS ( 'NONE', 3,
 ( #11687, #39472, #60233, #28213 ),
 .UNSPECIFIED., .F., .F.,
 ( 4, 4 ),
 ( 9.900409499052487190E-07, 0.05658314289920111928 ),
 .UNSPECIFIED. ) ;
#66768=CIRCLE ( 'NONE', #8313, 24.99999999999985434 ) ;
#66787=DIRECTION ( 'NONE',  ( -0.7071067811865485719, 8.659560562354946417E-17, 0.7071067811865465735 ) ) ;
#66795=EDGE_CURVE ( 'NONE', #32221, #38399, #35164, .T. ) ;
#66799=CARTESIAN_POINT ( 'NONE',  ( 0.000000000000000000, 0.000000000000000000, 41.38025477438755928 ) ) ;
#66801=DIRECTION ( 'NONE',  ( 1.000000000000000000, 3.108624468950438313E-14, 0.000000000000000000 ) ) ;
#66802=ORIENTED_EDGE ( 'NONE', *, *, #17219, .F. ) ;
#66803=CARTESIAN_POINT ( 'NONE',  ( 36.64089410029568228, 65.45232906116417837, 170.0000000000000000 ) ) ;
#66804=CARTESIAN_POINT ( 'NONE',  ( -60.41792053122248518, -24.01035990323518376, 0.000000000000000000 ) ) ;
#66806=LINE ( 'NONE', #23187, #34537 ) ;
#66814=DIRECTION ( 'NONE',  ( 0.4738686624730094610, -0.8805955318567321166, 0.000000000000000000 ) ) ;
#66831=PLANE ( 'NONE',  #18408 ) ;
#66832=AXIS2_PLACEMENT_3D ( 'NONE', #50530, #44558, #8319 ) ;
#66834=CARTESIAN_POINT ( 'NONE',  ( -60.41792053122281914, 24.01035990323430624, 170.0000000000000000 ) ) ;
#66838=DIRECTION ( 'NONE',  ( 1.000000000000000000, 0.000000000000000000, 0.000000000000000000 ) ) ;
#66840=PLANE ( 'NONE',  #24420 ) ;
#66848=ORIENTED_EDGE ( 'NONE', *, *, #25030, .F. ) ;
#66849=DIRECTION ( 'NONE',  ( 0.4738686624730094610, -0.8805955318567321166, 0.000000000000000000 ) ) ;
#66850=CARTESIAN_POINT ( 'NONE',  ( 25.57615740168605711, -44.89060284968904568, 26.66469066592268433 ) ) ;
#66859=DIRECTION ( 'NONE',  ( -0.000000000000000000, -0.000000000000000000, -1.000000000000000000 ) ) ;
#66860=AXIS2_PLACEMENT_3D ( 'NONE', #26874, #7523, #18757 ) ;
#66878=VECTOR ( 'NONE', #22612, 1000.000000000000000 ) ;
#66891=CARTESIAN_POINT ( 'NONE',  ( -34.96012151086515019, 55.23134702900888016, 43.58025477438756212 ) ) ;
#66904=ADVANCED_FACE ( 'NONE', ( #4879 ), #61983, .T. ) ;
#66906=ORIENTED_EDGE ( 'NONE', *, *, #9830, .T. ) ;
#66914=VERTEX_POINT ( 'NONE', #31968 ) ;
#66920=DIRECTION ( 'NONE',  ( -0.7530714660036196273, 0.6579387259397027066, 0.000000000000000000 ) ) ;
#66922=AXIS2_PLACEMENT_3D ( 'NONE', #3197, #55965, #2499 ) ;
#66928=ORIENTED_EDGE ( 'NONE', *, *, #60485, .F. ) ;
#66930=ORIENTED_EDGE ( 'NONE', *, *, #6430, .F. ) ;
#66937=CARTESIAN_POINT ( 'NONE',  ( 9.962235950564870990, 64.23203137738423152, 170.0000000000000000 ) ) ;
#66938=DIRECTION ( 'NONE',  ( -0.9362348706397417564, 0.3513748240813305279, 0.000000000000000000 ) ) ;
#66951=CARTESIAN_POINT ( 'NONE',  ( -6.802008071587399840, 24.18409554641266368, 3.061616997868437868E-16 ) ) ;
#66959=CARTESIAN_POINT ( 'NONE',  ( -54.64247938334378318, 38.15500013578019889, 34.48241823999801881 ) ) ;
#66979=VERTEX_POINT ( 'NONE', #63969 ) ;
#66990=EDGE_CURVE ( 'NONE', #38709, #34764, #24982, .T. ) ;
#66991=ORIENTED_EDGE ( 'NONE', *, *, #12365, .F. ) ;
#67004=LINE ( 'NONE', #30384, #34131 ) ;
#67007=DIRECTION ( 'NONE',  ( 0.000000000000000000, 0.000000000000000000, 1.000000000000000000 ) ) ;
#67013=EDGE_LOOP ( 'NONE', ( #25998, #51402, #76, #33380, #30080, #9407, #65693, #66361, #27548 ) ) ;
#67017=VERTEX_POINT ( 'NONE', #37581 ) ;
#67021=LINE ( 'NONE', #57145, #34231 ) ;
#67023=CARTESIAN_POINT ( 'NONE',  ( 74.39890044415633952, 7.951074708187157114, 41.38025477438755928 ) ) ;
#67049=EDGE_LOOP ( 'NONE', ( #61476, #40974, #67464, #66586 ) ) ;
#67051=EDGE_CURVE ( 'NONE', #31287, #40883, #36191, .T. ) ;
#67052=FACE_OUTER_BOUND ( 'NONE', #61900, .T. ) ;
#67062=ORIENTED_EDGE ( 'NONE', *, *, #55986, .F. ) ;
#67073=ADVANCED_FACE ( 'NONE', ( #59374 ), #60887, .T. ) ;
#67075=EDGE_CURVE ( 'NONE', #66330, #22457, #17149, .T. ) ;
#67078=CARTESIAN_POINT ( 'NONE',  ( 18.19409201603431114, 72.94804796678661774, 133.5802547743875550 ) ) ;
#67082=CARTESIAN_POINT ( 'NONE',  ( 66.63364081668849792, 1.250000000000013323, 34.48241823979189036 ) ) ;
#67084=ADVANCED_FACE ( 'NONE', ( #22443 ), #60432, .T. ) ;
#67107=CARTESIAN_POINT ( 'NONE',  ( 0.000000000000000000, 0.000000000000000000, 40.00000000000003553 ) ) ;
#67111=B_SPLINE_CURVE_WITH_KNOTS ( 'NONE', 3,
 ( #7887, #58989, #247, #23714 ),
 .UNSPECIFIED., .F., .F.,
 ( 4, 4 ),
 ( 0.1259919275528356697, 0.1829744153748742441 ),
 .UNSPECIFIED. ) ;
#67115=CIRCLE ( 'NONE', #24426, 24.99999999999985434 ) ;
#67132=LINE ( 'NONE', #62869, #61729 ) ;
#67138=VERTEX_POINT ( 'NONE', #27714 ) ;
#67147=CARTESIAN_POINT ( 'NONE',  ( 70.34686579112809568, 18.11777090454216577, 170.0000000000000000 ) ) ;
#67158=EDGE_CURVE ( 'NONE', #9035, #7351, #37928, .T. ) ;
#67163=ORIENTED_EDGE ( 'NONE', *, *, #57121, .F. ) ;
#67166=CARTESIAN_POINT ( 'NONE',  ( 74.39890044415633952, 7.951074708187157114, 43.58025477438756923 ) ) ;
#67174=AXIS2_PLACEMENT_3D ( 'NONE', #11942, #28116, #39036 ) ;
#67185=CARTESIAN_POINT ( 'NONE',  ( -52.73319225379935205, 53.34578647582052469, 170.0000000000000000 ) ) ;
#67193=ORIENTED_EDGE ( 'NONE', *, *, #21212, .T. ) ;
#67200=VERTEX_POINT ( 'NONE', #6616 ) ;
#67207=ADVANCED_FACE ( 'NONE', ( #995 ), #17508, .T. ) ;
#67217=EDGE_LOOP ( 'NONE', ( #55784, #10785, #36684, #14261 ) ) ;
#67219=VECTOR ( 'NONE', #50463, 1000.000000000000114 ) ;
#67224=VECTOR ( 'NONE', #16556, 1000.000000000000000 ) ;
#67236=ORIENTED_EDGE ( 'NONE', *, *, #45702, .T. ) ;
#67239=CARTESIAN_POINT ( 'NONE',  ( 74.39890044415651005, -7.951074708186092188, 3.061616997868437868E-16 ) ) ;
#67249=FACE_OUTER_BOUND ( 'NONE', #48964, .T. ) ;
#67252=CARTESIAN_POINT ( 'NONE',  ( 39.77028211725738061, 51.87520073220942152, 43.58025477438756212 ) ) ;
#67253=DIRECTION ( 'NONE',  ( 0.000000000000000000, 0.000000000000000000, 1.000000000000000000 ) ) ;
#67258=DIRECTION ( 'NONE',  ( -1.000000000000000000, 0.000000000000000000, 0.000000000000000000 ) ) ;
#67262=B_SPLINE_CURVE_WITH_KNOTS ( 'NONE', 3,
 ( #20971, #36118, #68472, #25574 ),
 .UNSPECIFIED., .F., .F.,
 ( 4, 4 ),
 ( 9.900409498943429581E-07, 0.05658314289920114704 ),
 .UNSPECIFIED. ) ;
#67263=CIRCLE ( 'NONE', #6585, 24.99999999999985434 ) ;
#67266=DIRECTION ( 'NONE',  ( -1.000000000000000000, 0.000000000000000000, 0.000000000000000000 ) ) ;
#67267=CARTESIAN_POINT ( 'NONE',  ( 64.97411640938599930, 37.36411256620309018, 41.38025477438755928 ) ) ;
#67278=CARTESIAN_POINT ( 'NONE',  ( -40.53976227448249858, 9.891533029231922569, 13.79046412299628344 ) ) ;
#67282=EDGE_CURVE ( 'NONE', #23514, #27926, #2050, .T. ) ;
#67298=VERTEX_POINT ( 'NONE', #29462 ) ;
#67326=CYLINDRICAL_SURFACE ( 'NONE', #11699, 65.36598343705435354 ) ;
#67330=ORIENTED_EDGE ( 'NONE', *, *, #45326, .T. ) ;
#67338=LINE ( 'NONE', #14205, #29547 ) ;
#67342=LINE ( 'NONE', #17759, #68646 ) ;
#67346=DIRECTION ( 'NONE',  ( -0.9009688679024218105, 0.4338837391175525693, 0.000000000000000000 ) ) ;
#67354=CARTESIAN_POINT ( 'NONE',  ( 0.000000000000000000, 0.000000000000000000, 0.000000000000000000 ) ) ;
#67356=PLANE ( 'NONE',  #65024 ) ;
#67357=ORIENTED_EDGE ( 'NONE', *, *, #31315, .F. ) ;
#67364=DIRECTION ( 'NONE',  ( -0.9362348706397369824, -0.3513748240813435175, 0.000000000000000000 ) ) ;
#67390=DIRECTION ( 'NONE',  ( 0.000000000000000000, 0.000000000000000000, 1.000000000000000000 ) ) ;
#67393=CARTESIAN_POINT ( 'NONE',  ( -4.164416015345870470, 64.86646004871185767, 40.00000000000003553 ) ) ;
#67396=VERTEX_POINT ( 'NONE', #5404 ) ;
#67397=ORIENTED_EDGE ( 'NONE', *, *, #26229, .F. ) ;
#67400=CARTESIAN_POINT ( 'NONE',  ( 38.31361596636786260, -1.250000000000021982, 13.32819397642333570 ) ) ;
#67401=CARTESIAN_POINT ( 'NONE',  ( -67.57266509268163190, 32.54128043381644630, 43.58025477438756212 ) ) ;
#67407=EDGE_CURVE ( 'NONE', #40972, #52786, #63808, .T. ) ;
#67409=LINE ( 'NONE', #30458, #55352 ) ;
#67435=CARTESIAN_POINT ( 'NONE',  ( 0.000000000000000000, 0.000000000000000000, 41.38025477438755928 ) ) ;
#67437=EDGE_CURVE ( 'NONE', #16812, #57236, #17704, .T. ) ;
#67440=DIRECTION ( 'NONE',  ( -0.8090169943749422332, -0.5877852522924802425, 0.000000000000000000 ) ) ;
#67444=B_SPLINE_CURVE_WITH_KNOTS ( 'NONE', 3,
 ( #22549, #29223, #28163, #39094 ),
 .UNSPECIFIED., .F., .F.,
 ( 4, 4 ),
 ( 9.900409499097199942E-07, 0.05658314289920114010 ),
 .UNSPECIFIED. ) ;
#67447=ORIENTED_EDGE ( 'NONE', *, *, #57972, .F. ) ;
#67454=EDGE_CURVE ( 'NONE', #32990, #32477, #49763, .T. ) ;
#67455=ADVANCED_FACE ( 'NONE', ( #28603 ), #28239, .T. ) ;
#67463=LINE ( 'NONE', #19255, #37373 ) ;
#67464=ORIENTED_EDGE ( 'NONE', *, *, #26766, .T. ) ;
#67466=CARTESIAN_POINT ( 'NONE',  ( -17.90772993695116355, 72.84144224619130625, 73.58025477438756923 ) ) ;
#67467=DIRECTION ( 'NONE',  ( -0.000000000000000000, -0.000000000000000000, -1.000000000000000000 ) ) ;
#67470=DIRECTION ( 'NONE',  ( 0.7227948638273878901, 0.6910626489868685329, 0.000000000000000000 ) ) ;
#67474=VERTEX_POINT ( 'NONE', #23336 ) ;
#67481=PLANE ( 'NONE',  #766 ) ;
#67486=CIRCLE ( 'NONE', #52840, 65.36598343705435354 ) ;
#67487=CARTESIAN_POINT ( 'NONE',  ( 73.79471914489741380, -13.39176710989671726, 43.58025477438756212 ) ) ;
#67511=FILL_AREA_STYLE ('',( #51676 ) ) ;
#67523=ORIENTED_EDGE ( 'NONE', *, *, #53176, .T. ) ;
#67530=VERTEX_POINT ( 'NONE', #59827 ) ;
#67539=FACE_OUTER_BOUND ( 'NONE', #69570, .T. ) ;
#67541=DIRECTION ( 'NONE',  ( -0.8345732537212999791, -0.5508969814521065267, 2.500042656554809847E-16 ) ) ;
#67549=ORIENTED_EDGE ( 'NONE', *, *, #44739, .T. ) ;
#67559=ORIENTED_EDGE ( 'NONE', *, *, #42926, .F. ) ;
#67560=FACE_OUTER_BOUND ( 'NONE', #43982, .T. ) ;
#67565=DIRECTION ( 'NONE',  ( 0.1342332658176522420, 0.9909497617679352555, 0.000000000000000000 ) ) ;
#67571=DIRECTION ( 'NONE',  ( -0.9009688679024218105, 0.4338837391175525693, 0.000000000000000000 ) ) ;
#67582=AXIS2_PLACEMENT_3D ( 'NONE', #35642, #13826, #34614 ) ;
#67592=EDGE_CURVE ( 'NONE', #29614, #10617, #39690, .T. ) ;
#67594=EDGE_CURVE ( 'NONE', #20715, #4283, #23375, .T. ) ;
#67599=CARTESIAN_POINT ( 'NONE',  ( 18.89356949897823768, 62.19351277735707839, 170.0000000000000000 ) ) ;
#67608=EDGE_LOOP ( 'NONE', ( #3142, #61142, #11832, #17958 ) ) ;
#67611=EDGE_LOOP ( 'NONE', ( #50994, #69199, #9308, #44531 ) ) ;
#67615=CARTESIAN_POINT ( 'NONE',  ( 0.000000000000000000, 0.000000000000000000, 170.0000000000000000 ) ) ;
#67618=EDGE_LOOP ( 'NONE', ( #10815, #49472, #49902, #34721, #69467, #14055, #10228, #31598, #64268 ) ) ;
#67621=AXIS2_PLACEMENT_3D ( 'NONE', #51197, #19521, #61048 ) ;
#67630=ORIENTED_EDGE ( 'NONE', *, *, #53666, .F. ) ;
#67632=VERTEX_POINT ( 'NONE', #13401 ) ;
#67657=EDGE_LOOP ( 'NONE', ( #10626, #69049, #23179, #55621 ) ) ;
#67658=EDGE_CURVE ( 'NONE', #28608, #4543, #56301, .T. ) ;
#67659=B_SPLINE_CURVE_WITH_KNOTS ( 'NONE', 3,
 ( #34009, #12910, #55810, #7277 ),
 .UNSPECIFIED., .F., .F.,
 ( 4, 4 ),
 ( 0.1259919275528362803, 0.1829744153748757984 ),
 .UNSPECIFIED. ) ;
#67662=DIRECTION ( 'NONE',  ( 2.497525279955783991E-16, 1.121639896553914790E-17, 1.000000000000000000 ) ) ;
#67663=CARTESIAN_POINT ( 'NONE',  ( 0.000000000000000000, 0.000000000000000000, 170.0000000000000000 ) ) ;
#67671=DIRECTION ( 'NONE',  ( 1.000000000000000000, -4.352074256530614270E-14, 0.000000000000000000 ) ) ;
#67674=CARTESIAN_POINT ( 'NONE',  ( -59.94154301275507635, -45.09516516490467808, 170.0000000000000000 ) ) ;
#67677=DIRECTION ( 'NONE',  ( 1.000000000000000000, -2.753353101070388220E-14, 0.000000000000000000 ) ) ;
#67683=VERTEX_POINT ( 'NONE', #47124 ) ;
#67688=CARTESIAN_POINT ( 'NONE',  ( 75.00000000000000000, -1.250000000000021094, 170.0000000000000000 ) ) ;
#67691=LINE ( 'NONE', #47244, #29991 ) ;
#67693=CARTESIAN_POINT ( 'NONE',  ( -15.67984581961064450, 63.08044415722863363, 40.00000000000003553 ) ) ;
#67695=VERTEX_POINT ( 'NONE', #46091 ) ;
#67708=VERTEX_POINT ( 'NONE', #14772 ) ;
#67715=DIRECTION ( 'NONE',  ( -0.2225209339563042066, -0.9749279121818259508, 0.000000000000000000 ) ) ;
#67717=AXIS2_PLACEMENT_3D ( 'NONE', #32215, #52955, #31189 ) ;
#67722=DIRECTION ( 'NONE',  ( -1.000000000000000000, 0.000000000000000000, 0.000000000000000000 ) ) ;
#67728=CONICAL_SURFACE ( 'NONE', #16189, 74.95140232871122521, 0.8777644062502172329 ) ;
#67731=VERTEX_POINT ( 'NONE', #68588 ) ;
#67734=AXIS2_PLACEMENT_3D ( 'NONE', #12880, #55783, #54363 ) ;
#67737=CARTESIAN_POINT ( 'NONE',  ( -60.67627457812130132, 44.08389392193514311, 43.58025477438756212 ) ) ;
#67742=ADVANCED_FACE ( 'NONE', ( #67560 ), #35892, .T. ) ;
#67750=EDGE_CURVE ( 'NONE', #21034, #47508, #10180, .T. ) ;
#67765=VERTEX_POINT ( 'NONE', #57695 ) ;
#67766=CIRCLE ( 'NONE', #64372, 25.12245591505646303 ) ;
#67769=DIRECTION ( 'NONE',  ( -1.000000000000000000, 0.000000000000000000, 0.000000000000000000 ) ) ;
#67796=ORIENTED_EDGE ( 'NONE', *, *, #37465, .T. ) ;
#67800=EDGE_CURVE ( 'NONE', #35639, #10115, #67913, .T. ) ;
#67816=VECTOR ( 'NONE', #58130, 1000.000000000000000 ) ;
#67817=EDGE_CURVE ( 'NONE', #62563, #50848, #36927, .T. ) ;
#67827=DIRECTION ( 'NONE',  ( -1.000000000000000000, 0.000000000000000000, 0.000000000000000000 ) ) ;
#67830=DIRECTION ( 'NONE',  ( 1.000000000000000000, 0.000000000000000000, 0.000000000000000000 ) ) ;
#67840=ORIENTED_EDGE ( 'NONE', *, *, #33424, .T. ) ;
#67845=CARTESIAN_POINT ( 'NONE',  ( 57.16566303090297652, -11.64445445351497277, 27.58472315868179692 ) ) ;
#67850=EDGE_CURVE ( 'NONE', #30492, #16812, #2693, .T. ) ;
#67857=CARTESIAN_POINT ( 'NONE',  ( 0.000000000000000000, 0.000000000000000000, 170.0000000000000000 ) ) ;
#67863=CIRCLE ( 'NONE', #37500, 65.36598343705435354 ) ;
#67872=ORIENTED_EDGE ( 'NONE', *, *, #58904, .T. ) ;
#67875=AXIS2_PLACEMENT_3D ( 'NONE', #67354, #8608, #61367 ) ;
#67876=ORIENTED_EDGE ( 'NONE', *, *, #61637, .T. ) ;
#67892=CARTESIAN_POINT ( 'NONE',  ( -74.81012118577218928, -5.477980300263997293, 170.0000000000000000 ) ) ;
#67910=EDGE_CURVE ( 'NONE', #61402, #2404, #53421, .T. ) ;
#67913=LINE ( 'NONE', #19361, #8267 ) ;
#67916=ADVANCED_FACE ( 'NONE', ( #32340 ), #42541, .T. ) ;
#67922=CARTESIAN_POINT ( 'NONE',  ( 0.000000000000000000, 0.000000000000000000, 170.0000000000000000 ) ) ;
#67928=EDGE_LOOP ( 'NONE', ( #26211, #17616, #56111, #64759, #26887, #60781, #25750, #12846, #33770 ) ) ;
#67944=EDGE_CURVE ( 'NONE', #53513, #46155, #4939, .T. ) ;
#67945=VERTEX_POINT ( 'NONE', #15807 ) ;
#67946=ORIENTED_EDGE ( 'NONE', *, *, #11204, .F. ) ;
#67954=DIRECTION ( 'NONE',  ( 0.9362348706397369824, 0.3513748240813435175, 0.000000000000000000 ) ) ;
#67956=ORIENTED_EDGE ( 'NONE', *, *, #63552, .T. ) ;
#67967=VECTOR ( 'NONE', #33199, 1000.000000000000000 ) ;
#67971=AXIS2_PLACEMENT_3D ( 'NONE', #51692, #30586, #36207 ) ;
#67979=LINE ( 'NONE', #19779, #15287 ) ;
#67984=DIRECTION ( 'NONE',  ( -0.8090169943749422332, -0.5877852522924802425, 0.000000000000000000 ) ) ;
#67999=EDGE_CURVE ( 'NONE', #46342, #20715, #65391, .T. ) ;
#68002=CYLINDRICAL_SURFACE ( 'NONE', #22101, 65.00000000000000000 ) ;
#68003=DIRECTION ( 'NONE',  ( 0.000000000000000000, 0.000000000000000000, 1.000000000000000000 ) ) ;
#68007=DIRECTION ( 'NONE',  ( -0.000000000000000000, -0.000000000000000000, -1.000000000000000000 ) ) ;
#68008=ORIENTED_EDGE ( 'NONE', *, *, #63838, .T. ) ;
#68011=CARTESIAN_POINT ( 'NONE',  ( -53.60725281709859757, -37.40286400928327026, 41.38025477438755928 ) ) ;
#68012=FACE_OUTER_BOUND ( 'NONE', #43531, .T. ) ;
#68018=CIRCLE ( 'NONE', #26429, 65.00000000000000000 ) ;
#68019=CYLINDRICAL_SURFACE ( 'NONE', #51431, 65.36598343705435354 ) ;
#68021=DIRECTION ( 'NONE',  ( -0.000000000000000000, -0.000000000000000000, -1.000000000000000000 ) ) ;
#68026=LINE ( 'NONE', #41284, #26523 ) ;
#68027=AXIS2_PLACEMENT_3D ( 'NONE', #52556, #31795, #20537 ) ;
#68030=VECTOR ( 'NONE', #63026, 999.9999999999998863 ) ;
#68037=CARTESIAN_POINT ( 'NONE',  ( -81.83265147652316784, 46.58665115056957973, 73.58025477438758344 ) ) ;
#68049=CARTESIAN_POINT ( 'NONE',  ( -41.50537345350632279, -50.04124777106357413, 170.0000000000000000 ) ) ;
#68060=EDGE_CURVE ( 'NONE', #26272, #21469, #13936, .T. ) ;
#68066=ORIENTED_EDGE ( 'NONE', *, *, #65705, .F. ) ;
#68070=ORIENTED_EDGE ( 'NONE', *, *, #23993, .F. ) ;
#68082=EDGE_CURVE ( 'NONE', #36640, #18239, #55167, .T. ) ;
#68092=ORIENTED_EDGE ( 'NONE', *, *, #58910, .F. ) ;
#68094=ORIENTED_EDGE ( 'NONE', *, *, #35351, .T. ) ;
#68113=EDGE_LOOP ( 'NONE', ( #5070, #33308, #33913, #45532 ) ) ;
#68122=VECTOR ( 'NONE', #34652, 1000.000000000000114 ) ;
#68127=VECTOR ( 'NONE', #11373, 1000.000000000000000 ) ;
#68131=ORIENTED_EDGE ( 'NONE', *, *, #44151, .F. ) ;
#68135=CARTESIAN_POINT ( 'NONE',  ( 0.000000000000000000, 0.000000000000000000, 170.0000000000000000 ) ) ;
#68137=CARTESIAN_POINT ( 'NONE',  ( -18.89790202299119315, -62.20684691518632548, 170.0000000000000000 ) ) ;
#68140=CYLINDRICAL_SURFACE ( 'NONE', #25008, 65.00000000000000000 ) ;
#68160=VERTEX_POINT ( 'NONE', #65309 ) ;
#68168=CARTESIAN_POINT ( 'NONE',  ( -37.03736007212398818, 19.22364788858845230, 13.79046340968178619 ) ) ;
#68173=VERTEX_POINT ( 'NONE', #52999 ) ;
#68177=AXIS2_PLACEMENT_3D ( 'NONE', #28454, #35168, #29899 ) ;
#68201=ORIENTED_EDGE ( 'NONE', *, *, #5622, .F. ) ;
#68202=DIRECTION ( 'NONE',  ( -1.000000000000000000, 0.000000000000000000, 0.000000000000000000 ) ) ;
#68208=DIRECTION ( 'NONE',  ( -0.000000000000000000, -0.000000000000000000, 1.000000000000000000 ) ) ;
#68216=VECTOR ( 'NONE', #66849, 1000.000000000000114 ) ;
#68227=ADVANCED_FACE ( 'NONE', ( #23454 ), #1998, .F. ) ;
#68244=ADVANCED_FACE ( 'NONE', ( #6564 ), #28547, .T. ) ;
#68294=VECTOR ( 'NONE', #65257, 1000.000000000000114 ) ;
#68299=VERTEX_POINT ( 'NONE', #28721 ) ;
#68305=VERTEX_POINT ( 'NONE', #33657 ) ;
#68314=AXIS2_PLACEMENT_3D ( 'NONE', #13406, #66541, #56307 ) ;
#68318=ADVANCED_FACE ( 'NONE', ( #49807 ), #1633, .F. ) ;
#68324=PLANE ( 'NONE',  #42138 ) ;
#68327=FACE_OUTER_BOUND ( 'NONE', #2010, .T. ) ;
#68332=CARTESIAN_POINT ( 'NONE',  ( 9.962235950564870990, 64.23203137738423152, 133.5802547743875550 ) ) ;
#68341=DIRECTION ( 'NONE',  ( -1.000000000000000000, 0.000000000000000000, 0.000000000000000000 ) ) ;
#68349=EDGE_LOOP ( 'NONE', ( #50446, #57370, #27782, #46919 ) ) ;
#68350=ORIENTED_EDGE ( 'NONE', *, *, #58743, .F. ) ;
#68352=CARTESIAN_POINT ( 'NONE',  ( 23.05216796272351232, -9.986758404123879274, 0.000000000000000000 ) ) ;
#68353=DIRECTION ( 'NONE',  ( 0.000000000000000000, -0.000000000000000000, -1.000000000000000000 ) ) ;
#68360=CARTESIAN_POINT ( 'NONE',  ( -74.58602291351357394, -7.967916035252095242, 170.0000000000000000 ) ) ;
#68363=DIRECTION ( 'NONE',  ( -0.000000000000000000, -0.000000000000000000, 1.000000000000000000 ) ) ;
#68367=DIRECTION ( 'NONE',  ( 2.616877698022258092E-18, -4.379915515250366329E-18, -1.000000000000000000 ) ) ;
#68368=EDGE_CURVE ( 'NONE', #24023, #40116, #61420, .T. ) ;
#68383=CYLINDRICAL_SURFACE ( 'NONE', #27424, 65.00000000000000000 ) ;
#68386=ORIENTED_EDGE ( 'NONE', *, *, #2696, .F. ) ;
#68390=CARTESIAN_POINT ( 'NONE',  ( -55.15976438495108169, -34.41253982194112382, 170.0000000000000000 ) ) ;
#68399=AXIS2_PLACEMENT_3D ( 'NONE', #12931, #33692, #38965 ) ;
#68407=VERTEX_POINT ( 'NONE', #69012 ) ;
#68410=CARTESIAN_POINT ( 'NONE',  ( 0.000000000000000000, 0.000000000000000000, 40.00000000000003553 ) ) ;
#68412=CARTESIAN_POINT ( 'NONE',  ( -33.17493614366368604, 47.98885325116288669, 27.58472369403420643 ) ) ;
#68423=CARTESIAN_POINT ( 'NONE',  ( -30.63688085183209253, 13.36654888745402836, 6.893342933764156300 ) ) ;
#68443=ADVANCED_FACE ( 'NONE', ( #35038 ), #31735, .T. ) ;
#68450=DIRECTION ( 'NONE',  ( 1.000000000000000000, 0.000000000000000000, 0.000000000000000000 ) ) ;
#68456=ORIENTED_EDGE ( 'NONE', *, *, #69325, .T. ) ;
#68459=CYLINDRICAL_SURFACE ( 'NONE', #36032, 65.00000000000000000 ) ;
#68461=EDGE_CURVE ( 'NONE', #59075, #31099, #42634, .T. ) ;
#68466=EDGE_CURVE ( 'NONE', #25958, #417, #68674, .T. ) ;
#68468=DIRECTION ( 'NONE',  ( -0.5877852522924802425, 0.8090169943749422332, 5.102127870520019688E-18 ) ) ;
#68469=CARTESIAN_POINT ( 'NONE',  ( -12.71198166530320606, 21.52685583500265665, 0.000000000000000000 ) ) ;
#68471=ORIENTED_EDGE ( 'NONE', *, *, #54533, .F. ) ;
#68472=CARTESIAN_POINT ( 'NONE',  ( -37.26544795852028358, 8.987879696173472155, 13.32819299319723605 ) ) ;
#68473=ORIENTED_EDGE ( 'NONE', *, *, #34942, .F. ) ;
#68484=DIRECTION ( 'NONE',  ( -0.000000000000000000, -0.000000000000000000, -1.000000000000000000 ) ) ;
#68496=VECTOR ( 'NONE', #41555, 1000.000000000000227 ) ;
#68498=LINE ( 'NONE', #57604, #30944 ) ;
#68507=CARTESIAN_POINT ( 'NONE',  ( 35.38849213634181723, -46.38060988817211694, 27.58472315868180402 ) ) ;
#68508=CYLINDRICAL_SURFACE ( 'NONE', #57671, 65.00000000000000000 ) ;
#68509=PLANE ( 'NONE',  #9759 ) ;
#68513=DIRECTION ( 'NONE',  ( -0.000000000000000000, -0.000000000000000000, -1.000000000000000000 ) ) ;
#68518=FACE_OUTER_BOUND ( 'NONE', #65930, .T. ) ;
#68519=ORIENTED_EDGE ( 'NONE', *, *, #40356, .T. ) ;
#68521=LINE ( 'NONE', #63248, #28587 ) ;
#68529=EDGE_CURVE ( 'NONE', #25377, #64121, #15905, .T. ) ;
#68530=EDGE_LOOP ( 'NONE', ( #13024, #42235, #30141, #47349, #30632, #13553, #59055, #61296, #39616 ) ) ;
#68533=VECTOR ( 'NONE', #48310, 1000.000000000000000 ) ;
#68539=FACE_OUTER_BOUND ( 'NONE', #34154, .T. ) ;
#68547=LINE ( 'NONE', #47418, #31693 ) ;
#68560=VERTEX_POINT ( 'NONE', #64434 ) ;
#68566=B_SPLINE_CURVE_WITH_KNOTS ( 'NONE', 3,
 ( #44580, #1667, #6242, #7297 ),
 .UNSPECIFIED., .F., .F.,
 ( 4, 4 ),
 ( 9.900409499072286585E-07, 0.05658314289920115397 ),
 .UNSPECIFIED. ) ;
#68578=AXIS2_PLACEMENT_3D ( 'NONE', #52920, #4745, #25536 ) ;
#68586=CARTESIAN_POINT ( 'NONE',  ( 55.61348889666937367, 50.24791103897128863, 41.38025477438755928 ) ) ;
#68587=ORIENTED_EDGE ( 'NONE', *, *, #33424, .F. ) ;
#68588=CARTESIAN_POINT ( 'NONE',  ( 39.54205320694412507, -51.58901073076707888, 40.00000000000003553 ) ) ;
#68592=B_SPLINE_CURVE_WITH_KNOTS ( 'NONE', 3,
 ( #63066, #41610, #19460, #46187 ),
 .UNSPECIFIED., .F., .F.,
 ( 4, 4 ),
 ( 9.900409498985715583E-07, 0.05658314289920115397 ),
 .UNSPECIFIED. ) ;
#68593=PLANE ( 'NONE',  #10901 ) ;
#68604=CARTESIAN_POINT ( 'NONE',  ( 39.77028211725815510, -51.87520073220884598, 43.58025477438756212 ) ) ;
#68610=CARTESIAN_POINT ( 'NONE',  ( 4.165045035621076863, -64.88046627338039229, 43.58025477438756923 ) ) ;
#68619=ORIENTED_EDGE ( 'NONE', *, *, #18660, .T. ) ;
#68629=ORIENTED_EDGE ( 'NONE', *, *, #61996, .T. ) ;
#68631=ORIENTED_EDGE ( 'NONE', *, *, #12613, .T. ) ;
#68646=VECTOR ( 'NONE', #8241, 1000.000000000000114 ) ;
#68650=LINE ( 'NONE', #36308, #19213 ) ;
#68653=DIRECTION ( 'NONE',  ( -2.201526392813400543E-16, -1.184691869787096980E-16, 1.000000000000000000 ) ) ;
#68663=CARTESIAN_POINT ( 'NONE',  ( -4.337405327941355360, 24.62086340933515416, 0.000000000000000000 ) ) ;
#68665=FACE_OUTER_BOUND ( 'NONE', #50871, .T. ) ;
#68669=CARTESIAN_POINT ( 'NONE',  ( 19.21260320704901403, -55.08522762473832302, 27.58472369377037126 ) ) ;
#68674=LINE ( 'NONE', #10615, #35274 ) ;
#68676=ORIENTED_EDGE ( 'NONE', *, *, #21801, .F. ) ;
#68678=ORIENTED_EDGE ( 'NONE', *, *, #67800, .T. ) ;
#68680=DIRECTION ( 'NONE',  ( -1.000000000000000000, 0.000000000000000000, 0.000000000000000000 ) ) ;
#68681=DIRECTION ( 'NONE',  ( -1.000000000000000000, 0.000000000000000000, 0.000000000000000000 ) ) ;
#68682=CARTESIAN_POINT ( 'NONE',  ( -24.51966494718108081, 5.470267094204372960, 3.061616997868437868E-16 ) ) ;
#68686=DIRECTION ( 'NONE',  ( -1.000000000000000000, 0.000000000000000000, 0.000000000000000000 ) ) ;
#68691=CARTESIAN_POINT ( 'NONE',  ( -8.712114576423861223, 23.56346432108866651, 0.000000000000000000 ) ) ;
#68711=DIRECTION ( 'NONE',  ( 0.000000000000000000, 0.000000000000000000, 1.000000000000000000 ) ) ;
#68715=CARTESIAN_POINT ( 'NONE',  ( -13.32397999417976564, -63.99361958670536410, 43.58025477438756212 ) ) ;
#68735=DIRECTION ( 'NONE',  ( -0.000000000000000000, -0.000000000000000000, -1.000000000000000000 ) ) ;
#68747=CARTESIAN_POINT ( 'NONE',  ( -23.14886993799584047, 9.760512885996790899, 3.061616997868437868E-16 ) ) ;
#68753=EDGE_CURVE ( 'NONE', #61903, #34081, #50691, .T. ) ;
#68761=VECTOR ( 'NONE', #14999, 1000.000000000000000 ) ;
#68782=ORIENTED_EDGE ( 'NONE', *, *, #5904, .F. ) ;
#68784=EDGE_CURVE ( 'NONE', #2078, #35908, #51398, .T. ) ;
#68789=ORIENTED_EDGE ( 'NONE', *, *, #20192, .F. ) ;
#68793=AXIS2_PLACEMENT_3D ( 'NONE', #19062, #61285, #29275 ) ;
#68794=DIRECTION ( 'NONE',  ( -1.000000000000000000, 0.000000000000000000, 0.000000000000000000 ) ) ;
#68796=VECTOR ( 'NONE', #31302, 1000.000000000000114 ) ;
#68797=LINE ( 'NONE', #52960, #25242 ) ;
#68798=VERTEX_POINT ( 'NONE', #45768 ) ;
#68799=CARTESIAN_POINT ( 'NONE',  ( 64.52696037203369883, -10.43950074664763683, 41.38025477438755928 ) ) ;
#68804=CARTESIAN_POINT ( 'NONE',  ( 63.74253542338254164, 39.54050679744534591, 170.0000000000000000 ) ) ;
#68806=CARTESIAN_POINT ( 'NONE',  ( 22.07550062443499428, -11.73338281062043364, 0.000000000000000000 ) ) ;
#68816=DIRECTION ( 'NONE',  ( -0.8345732537213078617, 0.5508969814520945363, 0.000000000000000000 ) ) ;
#68818=ORIENTED_EDGE ( 'NONE', *, *, #26883, .F. ) ;
#68828=CARTESIAN_POINT ( 'NONE',  ( -84.49322488516129681, 0.000000000000000000, 43.58025477438756212 ) ) ;
#68832=ORIENTED_EDGE ( 'NONE', *, *, #68898, .T. ) ;
#68836=CARTESIAN_POINT ( 'NONE',  ( 19.62566184736102315, -15.48655536434847413, 0.000000000000000000 ) ) ;
#68843=CIRCLE ( 'NONE', #19445, 65.36598343705435354 ) ;
#68853=CARTESIAN_POINT ( 'NONE',  ( 0.000000000000000000, 0.000000000000000000, 40.00000000000003553 ) ) ;
#68854=AXIS2_PLACEMENT_3D ( 'NONE', #18953, #40399, #61845 ) ;
#68872=CARTESIAN_POINT ( 'NONE',  ( 69.77839676787858991, 27.52340539440040956, 170.0000000000000000 ) ) ;
#68876=VERTEX_POINT ( 'NONE', #14784 ) ;
#68879=ORIENTED_EDGE ( 'NONE', *, *, #22647, .F. ) ;
#68884=CARTESIAN_POINT ( 'NONE',  ( 44.01696072966022655, -47.84694004974146253, 170.0000000000000000 ) ) ;
#68885=ORIENTED_EDGE ( 'NONE', *, *, #4289, .F. ) ;
#68888=LINE ( 'NONE', #14747, #37309 ) ;
#68889=VECTOR ( 'NONE', #18169, 1000.000000000000114 ) ;
#68892=AXIS2_PLACEMENT_3D ( 'NONE', #50344, #61915, #66194 ) ;
#68893=EDGE_CURVE ( 'NONE', #41788, #66440, #7370, .T. ) ;
#68898=EDGE_CURVE ( 'NONE', #38050, #38689, #20704, .T. ) ;
#68903=ORIENTED_EDGE ( 'NONE', *, *, #10397, .F. ) ;
#68910=DIRECTION ( 'NONE',  ( 0.000000000000000000, 0.000000000000000000, 1.000000000000000000 ) ) ;
#68911=CARTESIAN_POINT ( 'NONE',  ( -9.964117946888970678, -64.24592483216726180, 3.061616997868437868E-16 ) ) ;
#68923=EDGE_CURVE ( 'NONE', #56044, #13483, #58379, .T. ) ;
#68925=CARTESIAN_POINT ( 'NONE',  ( 6.564829507346455983, -24.24955267099640110, 0.000000000000000000 ) ) ;
#68928=ORIENTED_EDGE ( 'NONE', *, *, #49402, .T. ) ;
#68932=VERTEX_POINT ( 'NONE', #686 ) ;
#68935=LINE ( 'NONE', #49108, #14324 ) ;
#68939=VERTEX_POINT ( 'NONE', #64347 ) ;
#68941=ORIENTED_EDGE ( 'NONE', *, *, #18062, .F. ) ;
#68948=CIRCLE ( 'NONE', #12787, 25.12245591505646303 ) ;
#68956=PLANE ( 'NONE',  #46758 ) ;
#68962=ORIENTED_EDGE ( 'NONE', *, *, #13379, .F. ) ;
#68971=VERTEX_POINT ( 'NONE', #17191 ) ;
#68980=CARTESIAN_POINT ( 'NONE',  ( -10.27459169636330749, -50.63337651310006038, 26.66469066592268788 ) ) ;
#68984=CARTESIAN_POINT ( 'NONE',  ( 74.39890044415633952, 7.951074708187157114, 170.0000000000000000 ) ) ;
#68993=AXIS2_PLACEMENT_3D ( 'NONE', #99, #21555, #64473 ) ;
#68997=ORIENTED_EDGE ( 'NONE', *, *, #48734, .F. ) ;
#69007=CARTESIAN_POINT ( 'NONE',  ( 14.07802376132189970, -39.28261699430611742, 13.79046412305352121 ) ) ;
#69011=CARTESIAN_POINT ( 'NONE',  ( -2.113472939309121834, -74.92159864268212743, 41.38025477438755928 ) ) ;
#69012=CARTESIAN_POINT ( 'NONE',  ( 18.07314801315404296, -17.44990292519077002, 0.000000000000000000 ) ) ;
#69013=CARTESIAN_POINT ( 'NONE',  ( -15.24379698450855436, -38.84509498579587472, 13.79046412320005288 ) ) ;
#69016=DIRECTION ( 'NONE',  ( -1.000000000000000000, 0.000000000000000000, 0.000000000000000000 ) ) ;
#69018=LINE ( 'NONE', #42642, #12778 ) ;
#69027=CARTESIAN_POINT ( 'NONE',  ( -36.84489839129265931, -53.54860840895233309, 40.00000000000003553 ) ) ;
#69028=VECTOR ( 'NONE', #64238, 1000.000000000000000 ) ;
#69041=VECTOR ( 'NONE', #57055, 1000.000000000000114 ) ;
#69045=CIRCLE ( 'NONE', #48849, 65.36598343705435354 ) ;
#69047=CARTESIAN_POINT ( 'NONE',  ( -34.96012151086435438, -55.23134702900938464, 3.125053320693577513E-16 ) ) ;
#69049=ORIENTED_EDGE ( 'NONE', *, *, #63212, .T. ) ;
#69051=CARTESIAN_POINT ( 'NONE',  ( 57.30278335769613562, -48.40406511297320691, 43.58025477438756923 ) ) ;
#69055=DIRECTION ( 'NONE',  ( -0.5508969814521065267, 0.8345732537212999791, 0.000000000000000000 ) ) ;
#69061=DIRECTION ( 'NONE',  ( -1.000000000000000000, 0.000000000000000000, 0.000000000000000000 ) ) ;
#69062=DIRECTION ( 'NONE',  ( -1.000000000000000000, 0.000000000000000000, 0.000000000000000000 ) ) ;
#69067=VERTEX_POINT ( 'NONE', #27753 ) ;
#69069=PLANE ( 'NONE',  #49101 ) ;
#69071=CARTESIAN_POINT ( 'NONE',  ( -42.32797523529131922, 61.85511477251419166, 41.38025477438755928 ) ) ;
#69074=CARTESIAN_POINT ( 'NONE',  ( -59.94154301275570873, 45.09516516490385385, 170.0000000000000000 ) ) ;
#69077=ORIENTED_EDGE ( 'NONE', *, *, #61875, .T. ) ;
#69091=CARTESIAN_POINT ( 'NONE',  ( 48.39383208188444030, -43.94028683479018582, 43.58025477438756212 ) ) ;
#69094=EDGE_LOOP ( 'NONE', ( #8059, #41445, #29382, #541, #13565, #20029, #29493, #35243, #2702 ) ) ;
#69095=ORIENTED_EDGE ( 'NONE', *, *, #32463, .T. ) ;
#69106=DIRECTION ( 'NONE',  ( -0.000000000000000000, -0.000000000000000000, -1.000000000000000000 ) ) ;
#69109=CARTESIAN_POINT ( 'NONE',  ( 36.61292551086603453, 65.40035471292272007, 41.38025477438755928 ) ) ;
#69110=CARTESIAN_POINT ( 'NONE',  ( -65.36598343705435354, 0.000000000000000000, 41.38025477438755928 ) ) ;
#69115=B_SPLINE_CURVE_WITH_KNOTS ( 'NONE', 3,
 ( #13160, #55714, #7540, #28996, #23708, #45149 ),
 .UNSPECIFIED., .F., .F.,
 ( 4, 2, 4 ),
 ( 0.03218937259408886919, 0.06469834484649494843, 0.09720731709890104155 ),
 .UNSPECIFIED. ) ;
#69119=CARTESIAN_POINT ( 'NONE',  ( -15.47041015649555185, -73.39774458108232125, 170.0000000000000000 ) ) ;
#69123=VERTEX_POINT ( 'NONE', #1376 ) ;
#69124=ADVANCED_FACE ( 'NONE', ( #21778 ), #43226, .F. ) ;
#69130=AXIS2_PLACEMENT_3D ( 'NONE', #30087, #19520, #67722 ) ;
#69131=B_SPLINE_CURVE_WITH_KNOTS ( 'NONE', 3,
 ( #31003, #52450, #35235, #56690, #4267, #25730 ),
 .UNSPECIFIED., .F., .F.,
 ( 4, 2, 4 ),
 ( 1.095770181103599004E-06, 0.03239442681617710207, 0.06478775786217309818 ),
 .UNSPECIFIED. ) ;
#69145=CARTESIAN_POINT ( 'NONE',  ( 51.85299110299497016, -39.21848821248376282, 41.38025477438755928 ) ) ;
#69146=AXIS2_PLACEMENT_3D ( 'NONE', #4714, #47610, #63811 ) ;
#69151=CIRCLE ( 'NONE', #64690, 65.36598343705435354 ) ;
#69152=DIRECTION ( 'NONE',  ( 0.000000000000000000, 0.000000000000000000, 1.000000000000000000 ) ) ;
#69158=EDGE_LOOP ( 'NONE', ( #1605, #65575, #4312, #19029 ) ) ;
#69160=ADVANCED_FACE ( 'NONE', ( #61166 ), #29849, .T. ) ;
#69164=LINE ( 'NONE', #31888, #69028 ) ;
#69172=CARTESIAN_POINT ( 'NONE',  ( 29.69502258243350923, 57.82046033912877903, 170.0000000000000000 ) ) ;
#69196=VECTOR ( 'NONE', #100, 1000.000000000000000 ) ;
#69199=ORIENTED_EDGE ( 'NONE', *, *, #54505, .T. ) ;
#69204=CYLINDRICAL_SURFACE ( 'NONE', #9755, 65.00000000000000000 ) ;
#69205=CIRCLE ( 'NONE', #25397, 65.00000000000000000 ) ;
#69207=DIRECTION ( 'NONE',  ( 0.6579387259397138088, -0.7530714660036099684, 0.000000000000000000 ) ) ;
#69215=FACE_OUTER_BOUND ( 'NONE', #19454, .T. ) ;
#69217=DIRECTION ( 'NONE',  ( 0.000000000000000000, 0.000000000000000000, 1.000000000000000000 ) ) ;
#69219=CARTESIAN_POINT ( 'NONE',  ( -44.00727179482577611, 47.83680621839560132, 170.0000000000000000 ) ) ;
#69227=CARTESIAN_POINT ( 'NONE',  ( 0.000000000000000000, 0.000000000000000000, 73.58025477438756923 ) ) ;
#69236=DIRECTION ( 'NONE',  ( 0.000000000000000000, 0.000000000000000000, 1.000000000000000000 ) ) ;
#69250=AXIS2_PLACEMENT_3D ( 'NONE', #31209, #63555, #52975 ) ;
#69256=ORIENTED_EDGE ( 'NONE', *, *, #31936, .F. ) ;
#69261=EDGE_CURVE ( 'NONE', #58577, #48517, #25625, .T. ) ;
#69264=DIRECTION ( 'NONE',  ( 2.377681859532301304E-16, -7.725556675377196710E-17, 1.000000000000000000 ) ) ;
#69289=CARTESIAN_POINT ( 'NONE',  ( 57.25833571151937207, -48.36523237396138342, 41.38025477438755928 ) ) ;
#69292=CARTESIAN_POINT ( 'NONE',  ( 56.74421265833558436, 32.44697398030905333, 43.58025477438756212 ) ) ;
#69294=ORIENTED_EDGE ( 'NONE', *, *, #8361, .F. ) ;
#69300=CARTESIAN_POINT ( 'NONE',  ( 0.000000000000000000, 0.000000000000000000, 0.000000000000000000 ) ) ;
#69304=AXIS2_PLACEMENT_3D ( 'NONE', #57700, #47129, #25359 ) ;
#69319=ADVANCED_FACE ( 'NONE', ( #68518 ), #19993, .F. ) ;
#69323=VERTEX_POINT ( 'NONE', #4160 ) ;
#69324=EDGE_CURVE ( 'NONE', #6967, #13968, #26388, .T. ) ;
#69325=EDGE_CURVE ( 'NONE', #53557, #42385, #24924, .T. ) ;
#69339=VECTOR ( 'NONE', #33415, 1000.000000000000000 ) ;
#69341=ORIENTED_EDGE ( 'NONE', *, *, #30555, .T. ) ;
#69344=CARTESIAN_POINT ( 'NONE',  ( 24.46491470961352732, 5.710143558203322200, 3.061616997868437868E-16 ) ) ;
#69345=CARTESIAN_POINT ( 'NONE',  ( -42.36049017605873956, -61.90437280228297112, 43.58025477438756212 ) ) ;
#69348=DIRECTION ( 'NONE',  ( -1.000000000000000000, 0.000000000000000000, 0.000000000000000000 ) ) ;
#69350=CARTESIAN_POINT ( 'NONE',  ( 0.000000000000000000, 0.000000000000000000, 40.00000000000003553 ) ) ;
#69355=FACE_OUTER_BOUND ( 'NONE', #6656, .T. ) ;
#69359=ORIENTED_EDGE ( 'NONE', *, *, #13414, .T. ) ;
#69360=CARTESIAN_POINT ( 'NONE',  ( -65.00000000000000000, 0.000000000000000000, 170.0000000000000000 ) ) ;
#69369=CARTESIAN_POINT ( 'NONE',  ( 22.07550062443481664, 11.73338281062075872, 0.000000000000000000 ) ) ;
#69401=LINE ( 'NONE', #21221, #33665 ) ;
#69402=LINE ( 'NONE', #20516, #2393 ) ;
#69404=B_SPLINE_CURVE_WITH_KNOTS ( 'NONE', 3,
 ( #20422, #48171, #10900, #53108, #42900, #32371 ),
 .UNSPECIFIED., .F., .F.,
 ( 4, 2, 4 ),
 ( 1.095770181124384134E-06, 0.03239442681617711595, 0.06478775786217309818 ),
 .UNSPECIFIED. ) ;
#69405=VECTOR ( 'NONE', #25251, 1000.000000000000114 ) ;
#69425=VERTEX_POINT ( 'NONE', #597 ) ;
#69429=FACE_OUTER_BOUND ( 'NONE', #38678, .T. ) ;
#69432=CARTESIAN_POINT ( 'NONE',  ( 0.000000000000000000, 70.00000000000000000, 0.000000000000000000 ) ) ;
#69436=EDGE_LOOP ( 'NONE', ( #54487, #54999, #33950, #31977 ) ) ;
#69438=AXIS2_PLACEMENT_3D ( 'NONE', #12307, #38335, #28840 ) ;
#69440=CARTESIAN_POINT ( 'NONE',  ( 0.000000000000000000, 0.000000000000000000, 0.000000000000000000 ) ) ;
#69443=VECTOR ( 'NONE', #51361, 1000.000000000000227 ) ;
#69445=CARTESIAN_POINT ( 'NONE',  ( -2.113472939310175658, 74.92159864268209901, 41.38025477438755928 ) ) ;
#69446=CARTESIAN_POINT ( 'NONE',  ( 0.000000000000000000, 0.000000000000000000, 40.00000000000003553 ) ) ;
#69448=ORIENTED_EDGE ( 'NONE', *, *, #34877, .F. ) ;
#69463=FACE_OUTER_BOUND ( 'NONE', #19314, .T. ) ;
#69467=ORIENTED_EDGE ( 'NONE', *, *, #27350, .F. ) ;
#69476=VERTEX_POINT ( 'NONE', #17105 ) ;
#69482=ORIENTED_EDGE ( 'NONE', *, *, #34499, .F. ) ;
#69485=AXIS2_PLACEMENT_3D ( 'NONE', #66058, #50204, #5886 ) ;
#69488=AXIS2_PLACEMENT_3D ( 'NONE', #16826, #21415, #15800 ) ;
#69489=DIRECTION ( 'NONE',  ( 0.9009688679024155933, 0.4338837391175656699, 0.000000000000000000 ) ) ;
#69490=LINE ( 'NONE', #15351, #53318 ) ;
#69491=ORIENTED_EDGE ( 'NONE', *, *, #7857, .T. ) ;
#69506=CARTESIAN_POINT ( 'NONE',  ( -29.70166638324878150, -57.83280658984300970, 41.38025477438755928 ) ) ;
#69513=DIRECTION ( 'NONE',  ( 4.258099457802021297E-18, 2.810746842852143592E-18, -1.000000000000000000 ) ) ;
#69517=CARTESIAN_POINT ( 'NONE',  ( -1.683356153842345604, -65.34430428700412108, 43.58025477438756212 ) ) ;
#69518=CARTESIAN_POINT ( 'NONE',  ( 29.69502258243432635, -57.82046033912835270, 40.00000000000003553 ) ) ;
#69525=EDGE_CURVE ( 'NONE', #24447, #47168, #3134, .T. ) ;
#69535=EDGE_LOOP ( 'NONE', ( #59069, #12258, #6831, #56180 ) ) ;
#69539=CARTESIAN_POINT ( 'NONE',  ( -45.14452675491352096, -49.02628165194661847, 34.48241824012613677 ) ) ;
#69541=EDGE_CURVE ( 'NONE', #45468, #21445, #16432, .T. ) ;
#69567=EDGE_CURVE ( 'NONE', #35709, #7827, #17829, .T. ) ;
#69568=EDGE_CURVE ( 'NONE', #24108, #51034, #60389, .T. ) ;
#69570=EDGE_LOOP ( 'NONE', ( #44404, #37098, #41183, #14296 ) ) ;
ENDSEC;
END-ISO-10303-21;
